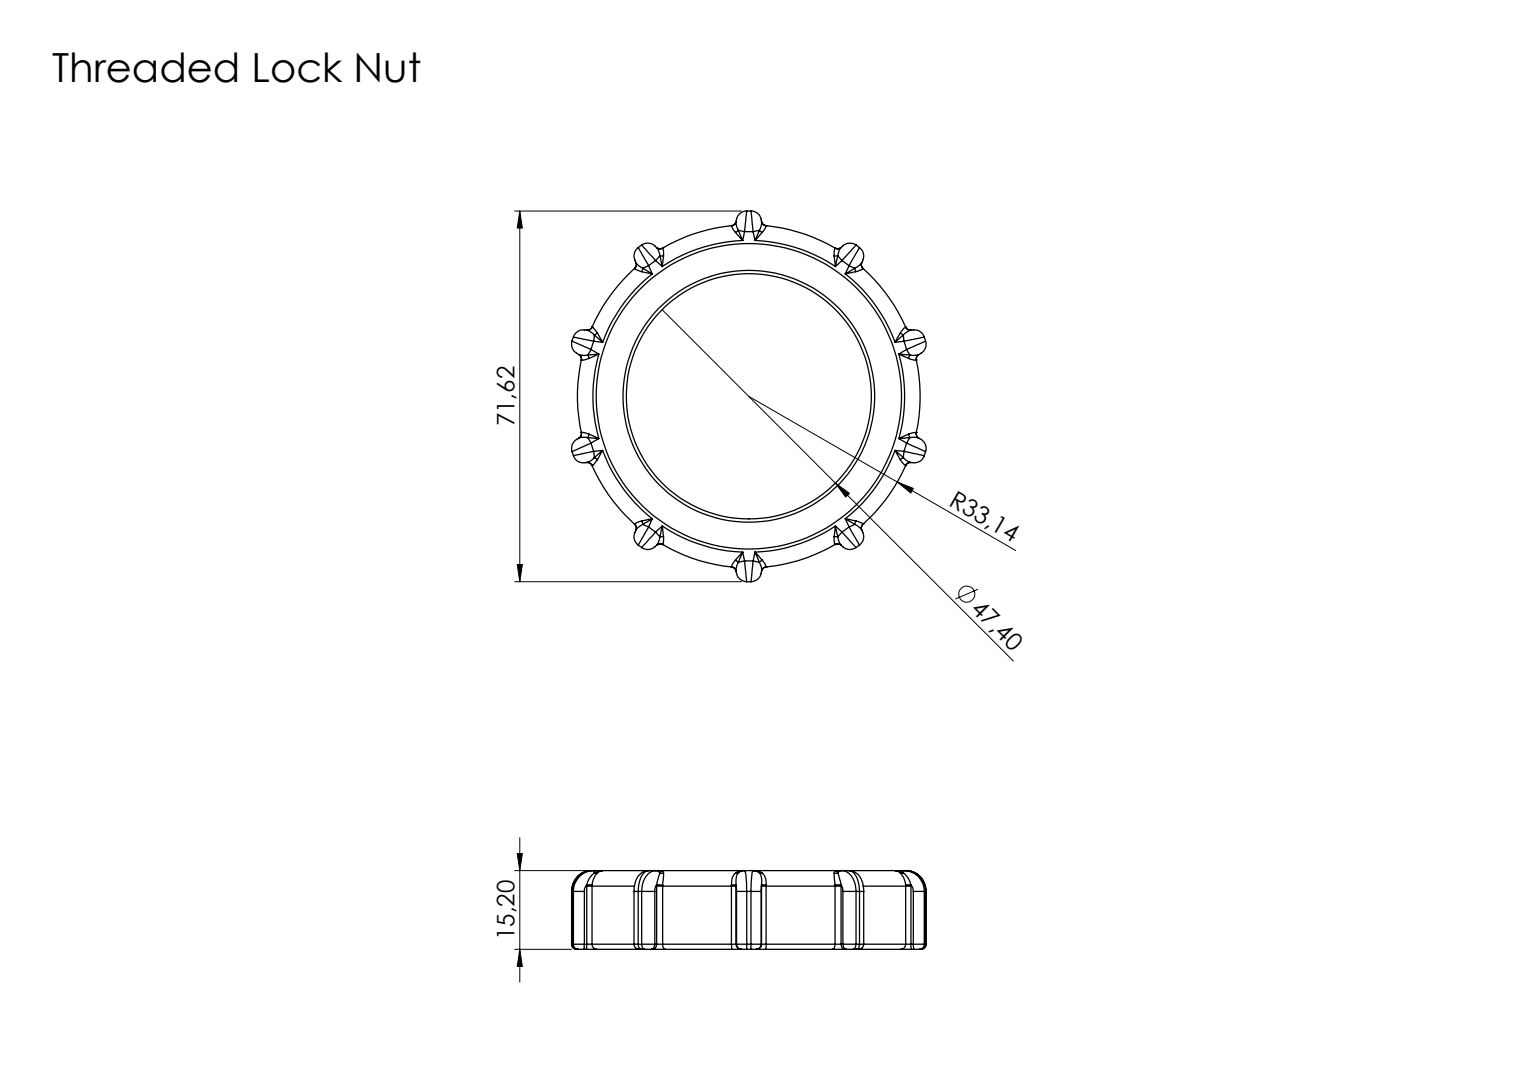
ISO-10303-21;
HEADER;
FILE_DESCRIPTION (('STEP AP214'),
    '1' );
FILE_NAME ('Threaded Lock Nut.step',
    '2026-10-06T09:49:54',
    ( '' ),
    ( '' ),
    'SwSTEP 2.0',
    'SolidWorks 2020',
    '' );
FILE_SCHEMA (( 'AUTOMOTIVE_DESIGN' ));
ENDSEC;

DATA;
#14=( BOUNDED_SURFACE ( )  B_SPLINE_SURFACE ( 3, 2, ( 
 ( #99288, #98203, #90906 ),
 ( #48377, #13076, #82520 ),
 ( #4699, #39956, #23138 ),
 ( #107158, #74130, #50021 ),
 ( #94768, #67940, #76875 ),
 ( #33745, #24238, #102047 ) ),
 .UNSPECIFIED., .F., .F., .F. ) 
 B_SPLINE_SURFACE_WITH_KNOTS ( ( 4, 2, 4 ),
 ( 3, 3 ),
 ( -1.474514954580286030E-17, 0.001312027981647312597, 0.002624055963294639939 ),
 ( 0.000000000000000000, 1.000000000000000000 ),
 .UNSPECIFIED. ) 
 GEOMETRIC_REPRESENTATION_ITEM ( )  RATIONAL_B_SPLINE_SURFACE ( (
 ( 1.000000000000000000, 0.9376006582765906705, 1.000000000000000000),
 ( 1.000000000000000000, 0.9569320108021501792, 1.000000000000000000),
 ( 1.000000000000000000, 0.9725743441620362528, 1.000000000000000000),
 ( 1.000000000000000000, 0.9942095667134138726, 1.000000000000000000),
 ( 1.000000000000000000, 1.000043666450818769, 1.000000000000000000),
 ( 1.000000000000000000, 1.000000000000000000, 1.000000000000000000) ) ) 
 REPRESENTATION_ITEM ( '' )  SURFACE ( )  );
#35=AXIS2_PLACEMENT_3D ( 'NONE', #53186, #17882, #45348 ) ;
#47=ORIENTED_EDGE ( 'NONE', *, *, #28974, .T. ) ;
#67=CARTESIAN_POINT ( 'NONE',  ( -1.491506560153236682, 1512.187213306747481, 242.6732489767341576 ) ) ;
#79=CARTESIAN_POINT ( 'NONE',  ( 21.64985223704960049, 1524.547395018738371, 234.6923279487310197 ) ) ;
#92=AXIS2_PLACEMENT_3D ( 'NONE', #81436, #4747, #22069 ) ;
#98=CARTESIAN_POINT ( 'NONE',  ( 32.97913964219430483, 1512.187213306747481, 197.9697544589745632 ) ) ;
#103=CARTESIAN_POINT ( 'NONE',  ( -2.622430729442981168, 1523.621879633028584, 242.1535192357228254 ) ) ;
#104=CARTESIAN_POINT ( 'NONE',  ( 2.470168521978398868, 1512.187213306747481, 175.3649660270905315 ) ) ;
#113=ORIENTED_EDGE ( 'NONE', *, *, #67279, .T. ) ;
#132=AXIS2_PLACEMENT_3D ( 'NONE', #29173, #87435, #11285 ) ;
#135=ORIENTED_EDGE ( 'NONE', *, *, #51675, .F. ) ;
#155=ORIENTED_EDGE ( 'NONE', *, *, #76478, .F. ) ;
#158=DIRECTION ( 'NONE',  ( 0.8672669759446630655, 0.000000000000000000, -0.4978433412588735285 ) ) ;
#164=AXIS2_PLACEMENT_3D ( 'NONE', #96746, #87233, #71584 ) ;
#171=ORIENTED_EDGE ( 'NONE', *, *, #62426, .F. ) ;
#178=DIRECTION ( 'NONE',  ( 0.000000000000000000, 0.000000000000000000, 1.000000000000000000 ) ) ;
#184=CIRCLE ( 'NONE', #28783, 1.000000000000007994 ) ;
#191=CARTESIAN_POINT ( 'NONE',  ( -20.12564951288306503, 1512.187213306747481, 180.7149624981946658 ) ) ;
#194=DIRECTION ( 'NONE',  ( -0.000000000000000000, -1.000000000000000000, 0.000000000000000000 ) ) ;
#196=CARTESIAN_POINT ( 'NONE',  ( 17.03788438627352519, 1524.775785348137333, 181.0918340916085754 ) ) ;
#216=CARTESIAN_POINT ( 'NONE',  ( 21.50855465202003813, 1524.374578187333327, 184.1253178261501660 ) ) ;
#237=VERTEX_POINT ( 'NONE', #65385 ) ;
#265=EDGE_CURVE ( 'NONE', #68013, #83547, #85444, .T. ) ;
#275=EDGE_LOOP ( 'NONE', ( #35605, #7044, #107686, #49764, #7625 ) ) ;
#282=AXIS2_PLACEMENT_3D ( 'NONE', #69728, #96558, #36645 ) ;
#285=LINE ( 'NONE', #92652, #110374 ) ;
#287=B_SPLINE_CURVE_WITH_KNOTS ( 'NONE', 3,
 ( #66514, #15499, #49697, #83827, #109592, #28341 ),
 .UNSPECIFIED., .F., .F.,
 ( 4, 2, 4 ),
 ( 2.797157557069881010E-17, 0.001087661325621732452, 0.002175322651243436715 ),
 .UNSPECIFIED. ) ;
#298=CARTESIAN_POINT ( 'NONE',  ( 18.86027053263898168, 1512.187213306747481, 230.7762769316004778 ) ) ;
#313=CARTESIAN_POINT ( 'NONE',  ( 31.55762699681125127, 1523.390106123591067, 196.3178534513329794 ) ) ;
#324=EDGE_CURVE ( 'NONE', #40683, #47896, #52438, .T. ) ;
#330=DIRECTION ( 'NONE',  ( -0.4978433412588676998, 0.000000000000000000, 0.8672669759446663962 ) ) ;
#338=B_SPLINE_CURVE_WITH_KNOTS ( 'NONE', 3,
 ( #14649, #33638, #59986, #52681 ),
 .UNSPECIFIED., .F., .F.,
 ( 4, 4 ),
 ( 0.000000000000000000, 0.0002960034161023847852 ),
 .UNSPECIFIED. ) ;
#359=EDGE_CURVE ( 'NONE', #10483, #4434, #57345, .T. ) ;
#394=TOROIDAL_SURFACE ( 'NONE', #71885, 30.13701971169416538, 3.000000000000000000 ) ;
#397=CARTESIAN_POINT ( 'NONE',  ( -29.67375955050042791, 1525.697946996596102, 221.2718133379099186 ) ) ;
#411=CARTESIAN_POINT ( 'NONE',  ( -33.93019615848938741, 1501.977400791986611, 220.5829544587966211 ) ) ;
#425=CARTESIAN_POINT ( 'NONE',  ( 2.570812331889315683, 1525.317349363550647, 176.7848501982247740 ) ) ;
#431=CARTESIAN_POINT ( 'NONE',  ( 16.66231036550702882, 1523.604703353109699, 180.4882076302513383 ) ) ;
#442=CARTESIAN_POINT ( 'NONE',  ( 0.000000000000000000, 1523.382868172864164, 209.1218459616979999 ) ) ;
#447=CARTESIAN_POINT ( 'NONE',  ( -19.53786426059057746, 1512.187213306747481, 181.5239794925695946 ) ) ;
#457=LINE ( 'NONE', #76585, #6239 ) ;
#461=CARTESIAN_POINT ( 'NONE',  ( 2.470955845399090300, 1523.580203803270933, 175.3687159542604377 ) ) ;
#490=DIRECTION ( 'NONE',  ( -0.000000000000000000, -1.000000000000000000, -0.000000000000000000 ) ) ;
#492=ORIENTED_EDGE ( 'NONE', *, *, #6899, .T. ) ;
#498=EDGE_LOOP ( 'NONE', ( #7346, #75123, #33311, #49048 ) ) ;
#501=CARTESIAN_POINT ( 'NONE',  ( -2.478666945488134932, 1524.659148609483054, 175.7709333987998548 ) ) ;
#506=CARTESIAN_POINT ( 'NONE',  ( 34.18677586421181758, 1522.382868172863937, 198.4504086008745389 ) ) ;
#518=DIRECTION ( 'NONE',  ( 0.000000000000000000, 0.000000000000000000, 1.000000000000000000 ) ) ;
#554=DIRECTION ( 'NONE',  ( -0.9942586961433764747, 0.000000000000000000, -0.1070030146457237041 ) ) ;
#563=DIRECTION ( 'NONE',  ( 0.000000000000000000, 0.000000000000000000, 1.000000000000000000 ) ) ;
#621=LINE ( 'NONE', #33094, #954 ) ;
#626=B_SPLINE_CURVE_WITH_KNOTS ( 'NONE', 3,
 ( #68362, #23563, #84575, #93517, #75649, #76185, #40921, #67801 ),
 .UNSPECIFIED., .F., .F.,
 ( 4, 2, 2, 4 ),
 ( 3.035766082959412415E-18, 0.001073044933456185606, 0.001609567400184306381, 0.002146089866912427591 ),
 .UNSPECIFIED. ) ;
#645=ORIENTED_EDGE ( 'NONE', *, *, #26884, .F. ) ;
#650=LINE ( 'NONE', #52152, #84998 ) ;
#657=ORIENTED_EDGE ( 'NONE', *, *, #45659, .F. ) ;
#680=CARTESIAN_POINT ( 'NONE',  ( -16.68062049856743201, 1524.382868172863937, 181.4122394607864521 ) ) ;
#682=( BOUNDED_CURVE ( )  B_SPLINE_CURVE ( 3, ( #67217, #42542, #1115, #52615 ),
 .UNSPECIFIED., .F., .F. ) 
 B_SPLINE_CURVE_WITH_KNOTS ( ( 4, 4 ),
 ( 2.436781329611985569, 3.141592653589793116 ),
 .UNSPECIFIED. ) 
 CURVE ( )  GEOMETRIC_REPRESENTATION_ITEM ( )  RATIONAL_B_SPLINE_CURVE ( ( 1.000000000000000000, 0.9590300661663091475, 0.9590300661663091475, 1.000000000000000000 ) ) 
 REPRESENTATION_ITEM ( '' )  );
#718=LINE ( 'NONE', #6885, #16918 ) ;
#728=CARTESIAN_POINT ( 'NONE',  ( -19.53786426059057746, 1512.187213306747481, 179.5239794925695946 ) ) ;
#736=CARTESIAN_POINT ( 'NONE',  ( 17.24701964721146297, 1523.844782250842400, 180.8504346226932569 ) ) ;
#749=FACE_OUTER_BOUND ( 'NONE', #68574, .T. ) ;
#812=CARTESIAN_POINT ( 'NONE',  ( 156.6846457583361882, 1524.382868172863937, 340.9912860285725174 ) ) ;
#821=CARTESIAN_POINT ( 'NONE',  ( 20.06033034266344828, 1526.189892541618974, 233.0619703228597643 ) ) ;
#830=EDGE_LOOP ( 'NONE', ( #94254, #75571, #96496 ) ) ;
#838=CARTESIAN_POINT ( 'NONE',  ( 34.68852446352940433, 1522.382868172863937, 199.9946320047950223 ) ) ;
#845=DIRECTION ( 'NONE',  ( -0.9125304618754018771, 0.000000000000000000, 0.4090087482554204401 ) ) ;
#848=CARTESIAN_POINT ( 'NONE',  ( 18.66420869458043441, 1526.382868172864164, 185.4599087859680537 ) ) ;
#850=ORIENTED_EDGE ( 'NONE', *, *, #22937, .F. ) ;
#858=CARTESIAN_POINT ( 'NONE',  ( 18.69816095120771493, 1522.382868172863937, 234.8576566410002897 ) ) ;
#863=EDGE_CURVE ( 'NONE', #108182, #30075, #109280, .T. ) ;
#870=EDGE_CURVE ( 'NONE', #24039, #32377, #39575, .T. ) ;
#875=EDGE_LOOP ( 'NONE', ( #11921, #86315, #53502, #106235 ) ) ;
#897=CARTESIAN_POINT ( 'NONE',  ( -30.95751052620455468, 1525.821544997590081, 201.4531494772889744 ) ) ;
#911=VERTEX_POINT ( 'NONE', #76256 ) ;
#912=FACE_OUTER_BOUND ( 'NONE', #72919, .T. ) ;
#941=CARTESIAN_POINT ( 'NONE',  ( -30.57821243133623668, 1525.253972588461693, 221.5701747116904130 ) ) ;
#942=VECTOR ( 'NONE', #92209, 1000.000000000000000 ) ;
#949=CARTESIAN_POINT ( 'NONE',  ( 22.08622291482349809, 1523.382868172864164, 233.8253038720783650 ) ) ;
#954=VECTOR ( 'NONE', #58866, 1000.000000000000114 ) ;
#956=EDGE_CURVE ( 'NONE', #90273, #106841, #7354, .T. ) ;
#957=DIRECTION ( 'NONE',  ( 0.000000000000000000, 1.000000000000000000, 0.000000000000000000 ) ) ;
#967=VERTEX_POINT ( 'NONE', #52531 ) ;
#970=CARTESIAN_POINT ( 'NONE',  ( 3.351189091698004940, 1524.075132568163781, 176.2264789961865006 ) ) ;
#972=CARTESIAN_POINT ( 'NONE',  ( -30.15585515321768995, 1524.425415513989719, 195.8365654344459870 ) ) ;
#988=FACE_OUTER_BOUND ( 'NONE', #72451, .T. ) ;
#989=DIRECTION ( 'NONE',  ( 0.000000000000000000, 0.000000000000000000, -1.000000000000000000 ) ) ;
#996=LINE ( 'NONE', #18854, #12421 ) ;
#1008=DIRECTION ( 'NONE',  ( 6.938893903907222067E-15, 0.000000000000000000, 1.000000000000000000 ) ) ;
#1017=DIRECTION ( 'NONE',  ( 0.03006000153033951128, -0.4884709562387339332, -0.8720622232497018400 ) ) ;
#1019=ADVANCED_FACE ( 'NONE', ( #35713 ), #50299, .T. ) ;
#1042=ORIENTED_EDGE ( 'NONE', *, *, #56606, .F. ) ;
#1054=DIRECTION ( 'NONE',  ( 0.000000000000000000, 1.000000000000000000, 0.000000000000000000 ) ) ;
#1071=CIRCLE ( 'NONE', #13577, 1.000000000000000888 ) ;
#1087=DIRECTION ( 'NONE',  ( 0.9977304882603014180, -0.06733403890946067227, 0.000000000000000000 ) ) ;
#1091=CARTESIAN_POINT ( 'NONE',  ( 30.04668324475564489, 1524.739563915922872, 195.9292732422738084 ) ) ;
#1093=CARTESIAN_POINT ( 'NONE',  ( -16.50400130224786466, 1525.907212628473644, 181.9890130758379030 ) ) ;
#1098=CARTESIAN_POINT ( 'NONE',  ( -1.336192060408252891, 1526.382868172863937, 178.6759496289172091 ) ) ;
#1115=CARTESIAN_POINT ( 'NONE',  ( 33.28034951413929576, 1522.862737210649584, 217.4407153818819438 ) ) ;
#1118=EDGE_CURVE ( 'NONE', #65949, #81284, #12787, .T. ) ;
#1127=EDGE_LOOP ( 'NONE', ( #104674, #75950, #35545, #11204 ) ) ;
#1142=DIRECTION ( 'NONE',  ( -0.7454942576402798782, -1.849942558231146277E-14, 0.6665120492724555534 ) ) ;
#1143=DIRECTION ( 'NONE',  ( 0.000000000000000000, 0.000000000000000000, 1.000000000000000000 ) ) ;
#1159=CARTESIAN_POINT ( 'NONE',  ( -30.04822308544821041, 1524.382868172804365, 221.7633950662771838 ) ) ;
#1193=CARTESIAN_POINT ( 'NONE',  ( -20.58427237330537096, 1512.187213306747481, 216.4826520421591738 ) ) ;
#1195=ORIENTED_EDGE ( 'NONE', *, *, #21286, .F. ) ;
#1198=CARTESIAN_POINT ( 'NONE',  ( 0.000000000000000000, 1518.913060387330006, 209.1218459616979999 ) ) ;
#1228=CARTESIAN_POINT ( 'NONE',  ( 29.86461515634908892, 1525.960063244516959, 197.2746849027934957 ) ) ;
#1229=CARTESIAN_POINT ( 'NONE',  ( -21.15382147014703662, 1525.425665131969254, 234.2558076767862190 ) ) ;
#1233=ORIENTED_EDGE ( 'NONE', *, *, #80838, .T. ) ;
#1250=EDGE_CURVE ( 'NONE', #83385, #104688, #28736, .T. ) ;
#1252=CARTESIAN_POINT ( 'NONE',  ( 17.73223409949387275, 1524.152444737676660, 237.7705223289944172 ) ) ;
#1265=CARTESIAN_POINT ( 'NONE',  ( 32.38845791999495560, 1518.913060387330006, 202.1182848005512085 ) ) ;
#1268=FACE_OUTER_BOUND ( 'NONE', #50912, .T. ) ;
#1287=CARTESIAN_POINT ( 'NONE',  ( 16.62425451295026946, 1524.075000532257491, 180.5391494807173842 ) ) ;
#1297=CARTESIAN_POINT ( 'NONE',  ( -19.53786426059057746, 1501.977400791986611, 181.5239794925695946 ) ) ;
#1306=CARTESIAN_POINT ( 'NONE',  ( 21.30905559964021023, 1524.964230758883104, 184.3256122676305893 ) ) ;
#1308=CARTESIAN_POINT ( 'NONE',  ( -0.4151546846821903003, 1512.187213306747481, 174.3106345060153046 ) ) ;
#1319=CARTESIAN_POINT ( 'NONE',  ( 32.78250617288045987, 1511.187213306747708, 218.3079823578266314 ) ) ;
#1324=ORIENTED_EDGE ( 'NONE', *, *, #28391, .T. ) ;
#1350=CARTESIAN_POINT ( 'NONE',  ( -31.34137657934001098, 1512.187213306747481, 221.9025654077414345 ) ) ;
#1362=ORIENTED_EDGE ( 'NONE', *, *, #19366, .T. ) ;
#1381=FACE_OUTER_BOUND ( 'NONE', #3200, .T. ) ;
#1385=DIRECTION ( 'NONE',  ( -0.000000000000000000, -1.000000000000000000, 0.000000000000000000 ) ) ;
#1386=ADVANCED_FACE ( 'NONE', ( #90829 ), #74050, .T. ) ;
#1398=CARTESIAN_POINT ( 'NONE',  ( -31.81407709660784988, 1522.382868172863937, 196.2902540610631945 ) ) ;
#1400=DIRECTION ( 'NONE',  ( -0.03006000153037464637, -0.4884709562387478665, -0.8720622232496929582 ) ) ;
#1431=CARTESIAN_POINT ( 'NONE',  ( -32.09351624765574940, 1524.374142163904025, 201.5415833658115901 ) ) ;
#1433=CARTESIAN_POINT ( 'NONE',  ( 16.66231036550724198, 1523.604703353109699, 237.7554842931445478 ) ) ;
#1438=DIRECTION ( 'NONE',  ( -0.9942586961433761417, -1.225281874271768203E-16, -0.1070030146457283393 ) ) ;
#1452=ORIENTED_EDGE ( 'NONE', *, *, #34105, .T. ) ;
#1464=EDGE_CURVE ( 'NONE', #13274, #40624, #28589, .T. ) ;
#1467=EDGE_CURVE ( 'NONE', #89438, #10483, #27113, .T. ) ;
#1481=CARTESIAN_POINT ( 'NONE',  ( 17.17241001986483795, 1512.187213306747481, 179.6185504016043240 ) ) ;
#1485=EDGE_LOOP ( 'NONE', ( #33168, #31647, #63478, #110389 ) ) ;
#1487=CARTESIAN_POINT ( 'NONE',  ( 2.470168521978401088, 1523.481610426287716, 242.8787258963054683 ) ) ;
#1506=EDGE_LOOP ( 'NONE', ( #67420, #97199, #19165, #75833 ) ) ;
#1516=CARTESIAN_POINT ( 'NONE',  ( -30.24841015875323791, 1524.082740465118832, 195.7700776127339566 ) ) ;
#1525=CARTESIAN_POINT ( 'NONE',  ( 2.397475438392864255, 1525.713797967456685, 243.2249543484664400 ) ) ;
#1531=CIRCLE ( 'NONE', #87365, 1.000000000000000888 ) ;
#1539=CIRCLE ( 'NONE', #69491, 2.000000000000001776 ) ;
#1550=VERTEX_POINT ( 'NONE', #21250 ) ;
#1567=DIRECTION ( 'NONE',  ( 0.000000000000000000, 0.000000000000000000, -1.000000000000000000 ) ) ;
#1568=CARTESIAN_POINT ( 'NONE',  ( 8.840620885073873225, 1512.187213306747481, 223.8289249455313268 ) ) ;
#1575=DIRECTION ( 'NONE',  ( 0.000000000000000000, 0.000000000000000000, 1.000000000000000000 ) ) ;
#1576=EDGE_CURVE ( 'NONE', #57810, #42994, #14529, .T. ) ;
#1584=DIRECTION ( 'NONE',  ( 0.000000000000000000, 0.000000000000000000, -1.000000000000000000 ) ) ;
#1594=ORIENTED_EDGE ( 'NONE', *, *, #76038, .T. ) ;
#1617=VECTOR ( 'NONE', #90374, 1000.000000000000114 ) ;
#1648=CARTESIAN_POINT ( 'NONE',  ( -32.86802468386279941, 1523.382868172864164, 217.2040256693919957 ) ) ;
#1651=CARTESIAN_POINT ( 'NONE',  ( 19.37374569213946174, 1526.382868172863937, 234.3668155954418921 ) ) ;
#1654=CARTESIAN_POINT ( 'NONE',  ( -22.69876404240057965, 1501.977400791986611, 236.8953202675781426 ) ) ;
#1665=CARTESIAN_POINT ( 'NONE',  ( -1.191524307911308700, 1526.382868172864164, 239.2353018730791518 ) ) ;
#1677=CARTESIAN_POINT ( 'NONE',  ( 30.90487439922560498, 1525.907212628473644, 216.4335774778780035 ) ) ;
#1685=EDGE_LOOP ( 'NONE', ( #19186, #71769, #109831, #40295 ) ) ;
#1689=CARTESIAN_POINT ( 'NONE',  ( -16.66936639845609491, 1523.382868172864164, 237.7608804993221838 ) ) ;
#1710=EDGE_CURVE ( 'NONE', #5224, #18098, #40044, .T. ) ;
#1737=VECTOR ( 'NONE', #83866, 1000.000000000000227 ) ;
#1751=DIRECTION ( 'NONE',  ( -0.7414773880254664773, 0.000000000000000000, 0.6709778558543730842 ) ) ;
#1753=EDGE_CURVE ( 'NONE', #23788, #59464, #24444, .T. ) ;
#1757=CARTESIAN_POINT ( 'NONE',  ( 17.84338787571921969, 1512.187213306747481, 180.3600277896298110 ) ) ;
#1790=VECTOR ( 'NONE', #84858, 1000.000000000000000 ) ;
#1795=DIRECTION ( 'NONE',  ( -0.000000000000000000, -1.000000000000000000, -0.000000000000000000 ) ) ;
#1813=CARTESIAN_POINT ( 'NONE',  ( -32.92528853941059452, 1523.611961620354123, 217.2368972417797863 ) ) ;
#1832=DIRECTION ( 'NONE',  ( 0.000000000000000000, 1.000000000000000000, 0.000000000000000000 ) ) ;
#1834=CARTESIAN_POINT ( 'NONE',  ( -30.15498238787951379, 1525.730671215514803, 196.9950476445848722 ) ) ;
#1854=CARTESIAN_POINT ( 'NONE',  ( 3.246772394788719929, 1511.187213306747708, 177.1492560608742224 ) ) ;
#1865=DIRECTION ( 'NONE',  ( 7.105427357601001859E-15, 0.000000000000000000, 1.000000000000000000 ) ) ;
#1870=CARTESIAN_POINT ( 'NONE',  ( -34.18677586421173231, 1512.187213306747481, 219.7932833225216882 ) ) ;
#1872=ORIENTED_EDGE ( 'NONE', *, *, #17077, .F. ) ;
#1875=CARTESIAN_POINT ( 'NONE',  ( 21.42841630977322254, 1524.678872986481338, 184.2224299175816782 ) ) ;
#1879=CARTESIAN_POINT ( 'NONE',  ( -32.37018134260410562, 1511.187213306747708, 200.1723992780599986 ) ) ;
#1882=CARTESIAN_POINT ( 'NONE',  ( 0.4151546846821903003, 1512.187213306747481, 174.3106345060153046 ) ) ;
#1895=VERTEX_POINT ( 'NONE', #51314 ) ;
#1919=FACE_OUTER_BOUND ( 'NONE', #94382, .T. ) ;
#1926=DIRECTION ( 'NONE',  ( 0.000000000000000000, 0.000000000000000000, -1.000000000000000000 ) ) ;
#1932=CARTESIAN_POINT ( 'NONE',  ( 30.15954682509860518, 1524.412928176728883, 222.4099428256023145 ) ) ;
#1963=EDGE_LOOP ( 'NONE', ( #6488, #63190, #36975, #109476, #109814 ) ) ;
#1974=CIRCLE ( 'NONE', #59192, 2.000000000000001776 ) ;
#1975=B_SPLINE_CURVE_WITH_KNOTS ( 'NONE', 3,
 ( #55220, #37302, #79860, #82037, #11547, #12644 ),
 .UNSPECIFIED., .F., .F.,
 ( 4, 2, 4 ),
 ( -1.285435071114344984E-05, 0.001079388306740470182, 0.002171630964192083728 ),
 .UNSPECIFIED. ) ;
#1999=ORIENTED_EDGE ( 'NONE', *, *, #72805, .F. ) ;
#2007=CARTESIAN_POINT ( 'NONE',  ( -32.54505059146748636, 1524.547395018738371, 201.1603553390793877 ) ) ;
#2029=AXIS2_PLACEMENT_3D ( 'NONE', #73611, #81412, #69901 ) ;
#2032=CARTESIAN_POINT ( 'NONE',  ( 30.31052258194596760, 1523.604703353109699, 222.4930856806589645 ) ) ;
#2039=ORIENTED_EDGE ( 'NONE', *, *, #25225, .T. ) ;
#2049=CARTESIAN_POINT ( 'NONE',  ( -29.86461515634905695, 1525.960063244516959, 220.9690070206026178 ) ) ;
#2057=CARTESIAN_POINT ( 'NONE',  ( 21.84020450211309949, 1523.481610118014487, 234.9798068777342621 ) ) ;
#2062=TOROIDAL_SURFACE ( 'NONE', #27074, 2.000000000000000000, 1.000000000000000000 ) ;
#2073=CARTESIAN_POINT ( 'NONE',  ( -19.91074080903786481, 1526.211528530236592, 184.7300577086374460 ) ) ;
#2075=AXIS2_PLACEMENT_3D ( 'NONE', #44071, #94439, #26132 ) ;
#2084=CARTESIAN_POINT ( 'NONE',  ( 34.18677586421183889, 1524.726013923371283, 198.4504086008744821 ) ) ;
#2104=ADVANCED_FACE ( 'NONE', ( #59734 ), #62997, .F. ) ;
#2107=DIRECTION ( 'NONE',  ( -0.000000000000000000, -1.000000000000000000, -0.000000000000000000 ) ) ;
#2119=CARTESIAN_POINT ( 'NONE',  ( 21.41971086555086501, 1512.187213306747481, 185.1638823089577670 ) ) ;
#2133=DIRECTION ( 'NONE',  ( 0.9942586961433768078, -1.225281874271768203E-16, 0.1070030146457215670 ) ) ;
#2134=ORIENTED_EDGE ( 'NONE', *, *, #30820, .F. ) ;
#2142=AXIS2_PLACEMENT_3D ( 'NONE', #10875, #61851, #26549 ) ;
#2148=( BOUNDED_CURVE ( )  B_SPLINE_CURVE ( 3, ( #59261, #8266, #50841, #58699 ),
 .UNSPECIFIED., .F., .T. ) 
 B_SPLINE_CURVE_WITH_KNOTS ( ( 4, 4 ),
 ( 0.000000000000000000, 0.7048113239778038830 ),
 .UNSPECIFIED. ) 
 CURVE ( )  GEOMETRIC_REPRESENTATION_ITEM ( )  RATIONAL_B_SPLINE_CURVE ( ( 1.000000000000000000, 0.9590300661663093695, 0.9590300661663093695, 1.000000000000000000 ) ) 
 REPRESENTATION_ITEM ( '' )  );
#2152=CARTESIAN_POINT ( 'NONE',  ( -76.99707197885047094, 1526.382868172863937, 398.8876973329340672 ) ) ;
#2166=CARTESIAN_POINT ( 'NONE',  ( -28.27139721233049485, 1526.382868172864164, 198.6830693683576499 ) ) ;
#2182=FACE_BOUND ( 'NONE', #61413, .T. ) ;
#2207=ADVANCED_FACE ( 'NONE', ( #57418 ), #23769, .T. ) ;
#2212=EDGE_LOOP ( 'NONE', ( #89470, #53230, #10682, #27900 ) ) ;
#2214=FACE_OUTER_BOUND ( 'NONE', #35175, .T. ) ;
#2219=AXIS2_PLACEMENT_3D ( 'NONE', #101752, #25040, #67643 ) ;
#2234=AXIS2_PLACEMENT_3D ( 'NONE', #36746, #10997, #20467 ) ;
#2236=DIRECTION ( 'NONE',  ( 0.000000000000000000, 0.000000000000000000, 1.000000000000000000 ) ) ;
#2251=CARTESIAN_POINT ( 'NONE',  ( -32.09337683451324352, 1524.374578187333555, 216.7020508011439972 ) ) ;
#2268=EDGE_CURVE ( 'NONE', #106220, #56418, #68854, .T. ) ;
#2279=CARTESIAN_POINT ( 'NONE',  ( 32.09337683451773415, 1524.374578187332645, 201.5416411222501267 ) ) ;
#2305=ORIENTED_EDGE ( 'NONE', *, *, #6899, .F. ) ;
#2326=ORIENTED_EDGE ( 'NONE', *, *, #108860, .T. ) ;
#2351=CARTESIAN_POINT ( 'NONE',  ( -18.88880210473032761, 1524.667648926078527, 179.4140113511354855 ) ) ;
#2354=( BOUNDED_SURFACE ( )  B_SPLINE_SURFACE ( 3, 2, ( 
 ( #65120, #13571, #21961 ),
 ( #48879, #74620, #64030 ),
 ( #48321, #30945, #98144 ),
 ( #4651, #30392, #5760 ),
 ( #38243, #99231, #22509 ),
 ( #56711, #90846, #14131 ),
 ( #99787, #64582, #107103 ),
 ( #98702, #90290, #47211 ),
 ( #5194, #23078, #55630 ),
 ( #15224, #4118, #39901 ) ),
 .UNSPECIFIED., .F., .F., .T. ) 
 B_SPLINE_SURFACE_WITH_KNOTS ( ( 4, 2, 2, 2, 4 ),
 ( 3, 3 ),
 ( 1.570796326794896558, 1.963495408493620697, 2.356194490192344837, 2.748893571891068976, 3.141592653589793116 ),
 ( 0.000000000000000000, 1.000000000000000000 ),
 .UNSPECIFIED. ) 
 GEOMETRIC_REPRESENTATION_ITEM ( )  RATIONAL_B_SPLINE_SURFACE ( (
 ( 1.000000000000000000, 0.7071067811865862085, 1.000000000000000000),
 ( 1.000000000000000000, 0.7166207884822426433, 1.000000000000000000),
 ( 1.000000000000000000, 0.7259222650906650420, 1.000000000000000000),
 ( 1.000000000000000000, 0.7428408967930791862, 1.000000000000000000),
 ( 1.000000000000000000, 0.7504512394528564112, 1.000000000000000000),
 ( 1.000000000000000000, 0.7630177051946440692, 1.000000000000000000),
 ( 1.000000000000000000, 0.7679730451973161287, 1.000000000000000000),
 ( 1.000000000000000000, 0.7746454561797309069, 1.000000000000000000),
 ( 1.000000000000000000, 0.7763684247035169683, 1.000000000000000000),
 ( 1.000000000000000000, 0.7763623250684379418, 1.000000000000000000) ) ) 
 REPRESENTATION_ITEM ( '' )  SURFACE ( )  );
#2363=DIRECTION ( 'NONE',  ( 0.000000000000000000, 1.000000000000000000, 0.000000000000000000 ) ) ;
#2365=ADVANCED_FACE ( 'NONE', ( #55352 ), #21144, .T. ) ;
#2377=CARTESIAN_POINT ( 'NONE',  ( 20.79738390328738973, 1512.187213306747481, 237.0406858230487899 ) ) ;
#2379=CARTESIAN_POINT ( 'NONE',  ( 17.43549085681724620, 1525.211473355384896, 237.2113236654630555 ) ) ;
#2387=CARTESIAN_POINT ( 'NONE',  ( 19.53786426059039982, 1512.187213306747481, 236.7197124308265188 ) ) ;
#2394=DIRECTION ( 'NONE',  ( -0.8090169943749422332, 0.000000000000000000, 0.5877852522924802425 ) ) ;
#2406=DIRECTION ( 'NONE',  ( -0.000000000000000000, -1.000000000000000000, -0.000000000000000000 ) ) ;
#2419=DIRECTION ( 'NONE',  ( -0.9510565162951559737, 0.000000000000000000, 0.3090169943749403458 ) ) ;
#2428=( LENGTH_UNIT ( ) NAMED_UNIT ( * ) SI_UNIT ( .MILLI., .METRE. ) );
#2431=ORIENTED_EDGE ( 'NONE', *, *, #101280, .T. ) ;
#2450=ORIENTED_EDGE ( 'NONE', *, *, #90057, .F. ) ;
#2457=FACE_OUTER_BOUND ( 'NONE', #57047, .T. ) ;
#2465=DIRECTION ( 'NONE',  ( 0.000000000000000000, 0.000000000000000000, 1.000000000000000000 ) ) ;
#2470=B_SPLINE_CURVE_WITH_KNOTS ( 'NONE', 3,
 ( #80697, #56045, #90172, #47644, #14015, #91291, #48205, #99120, #82343, #65559 ),
 .UNSPECIFIED., .F., .F.,
 ( 4, 2, 2, 2, 4 ),
 ( 0.000000000000000000, 0.0007403986298595355894, 0.001480797259719071179, 0.002221195889578606551, 0.002961594519438142357 ),
 .UNSPECIFIED. ) ;
#2472=ORIENTED_EDGE ( 'NONE', *, *, #39779, .T. ) ;
#2479=DIRECTION ( 'NONE',  ( -0.5877852522924780221, 0.000000000000000000, -0.8090169943749438985 ) ) ;
#2486=CARTESIAN_POINT ( 'NONE',  ( -31.55061275096994322, 1525.712830164893376, 217.0331825386441835 ) ) ;
#2494=CARTESIAN_POINT ( 'NONE',  ( -16.55387768533248760, 1524.739563915921963, 237.4558587828119300 ) ) ;
#2514=LINE ( 'NONE', #19254, #14480 ) ;
#2553=CIRCLE ( 'NONE', #40081, 33.13701971169416538 ) ;
#2560=DIRECTION ( 'NONE',  ( 0.000000000000000000, 0.000000000000000000, 1.000000000000000000 ) ) ;
#2566=CARTESIAN_POINT ( 'NONE',  ( -32.70818033930468971, 1524.201670966335314, 201.1172547305815499 ) ) ;
#2568=CARTESIAN_POINT ( 'NONE',  ( 32.37018134260406299, 1511.187213306747708, 218.0712926453362002 ) ) ;
#2574=VERTEX_POINT ( 'NONE', #32870 ) ;
#2598=LINE ( 'NONE', #45147, #87430 ) ;
#2608=ORIENTED_EDGE ( 'NONE', *, *, #64704, .T. ) ;
#2614=CARTESIAN_POINT ( 'NONE',  ( -41.95590887306661187, 1512.187213306747481, 225.5974093378525254 ) ) ;
#2627=CARTESIAN_POINT ( 'NONE',  ( -20.79738390328697761, 1512.187213306747481, 237.0406858230491025 ) ) ;
#2634=CARTESIAN_POINT ( 'NONE',  ( -34.09079054513859575, 1524.667648926078755, 200.3377533957330172 ) ) ;
#2635=CARTESIAN_POINT ( 'NONE',  ( -20.87481493262672316, 1525.712830164893376, 234.0672365764787628 ) ) ;
#2643=CARTESIAN_POINT ( 'NONE',  ( 0.4260839224734190300, 1523.429859730332510, 244.8289481157567593 ) ) ;
#2650=CARTESIAN_POINT ( 'NONE',  ( -2.136371150128812957, 1525.856065479248173, 241.3693944374256546 ) ) ;
#2664=ORIENTED_EDGE ( 'NONE', *, *, #37056, .F. ) ;
#2667=CARTESIAN_POINT ( 'NONE',  ( -18.69816095120731347, 1522.382868172863937, 234.8576566410005171 ) ) ;
#2676=AXIS2_PLACEMENT_3D ( 'NONE', #83147, #74218, #41693 ) ;
#2690=ORIENTED_EDGE ( 'NONE', *, *, #104370, .F. ) ;
#2696=FACE_OUTER_BOUND ( 'NONE', #32323, .T. ) ;
#2698=DIRECTION ( 'NONE',  ( 0.8386695113602744556, -0.4884709562387554715, 0.2408932868012610695 ) ) ;
#2719=AXIS2_PLACEMENT_3D ( 'NONE', #1308, #2982, #44980 ) ;
#2724=DIRECTION ( 'NONE',  ( -0.000000000000000000, -1.000000000000000000, -0.000000000000000000 ) ) ;
#2760=B_SPLINE_CURVE_WITH_KNOTS ( 'NONE', 3,
 ( #91547, #40036, #5890, #83688, #100491, #6984, #76396, #68026, #75852, #57959, #24862, #25414 ),
 .UNSPECIFIED., .F., .F.,
 ( 4, 2, 2, 2, 2, 4 ),
 ( 0.000000000000000000, 0.0007194225121803652289, 0.001079133768270242044, 0.001438845024360118968, 0.002158267536539317053, 0.002877690048718515789 ),
 .UNSPECIFIED. ) ;
#2805=CARTESIAN_POINT ( 'NONE',  ( 32.37018134260397062, 1512.187213306747481, 200.1723992780595438 ) ) ;
#2812=ORIENTED_EDGE ( 'NONE', *, *, #94728, .T. ) ;
#2813=VERTEX_POINT ( 'NONE', #60303 ) ;
#2828=CARTESIAN_POINT ( 'NONE',  ( 22.08622291482349809, 1523.456872492435195, 233.8253038720783366 ) ) ;
#2834=CIRCLE ( 'NONE', #61915, 0.9999999999999981126 ) ;
#2854=LINE ( 'NONE', #9023, #17151 ) ;
#2862=CARTESIAN_POINT ( 'NONE',  ( 19.37374569213945463, 1524.382868172863937, 234.3668155954418637 ) ) ;
#2876=ADVANCED_FACE ( 'NONE', ( #80412 ), #17111, .F. ) ;
#2877=VECTOR ( 'NONE', #103941, 1000.000000000000000 ) ;
#2896=CARTESIAN_POINT ( 'NONE',  ( -19.67623451925548039, 1525.581535527370761, 181.0581612214988638 ) ) ;
#2910=CARTESIAN_POINT ( 'NONE',  ( -17.17241001986463189, 1523.382868172864164, 238.6251415217917895 ) ) ;
#2920=ADVANCED_FACE ( 'NONE', ( #14838 ), #57974, .T. ) ;
#2926=CARTESIAN_POINT ( 'NONE',  ( 32.22536377336282953, 1523.621879633028811, 216.8351145222429466 ) ) ;
#2934=ORIENTED_EDGE ( 'NONE', *, *, #96685, .F. ) ;
#2937=CARTESIAN_POINT ( 'NONE',  ( 33.42844755917185751, 1522.382868172863937, 196.1165140606791226 ) ) ;
#2941=CARTESIAN_POINT ( 'NONE',  ( -29.75841426815548019, 1525.320827368860364, 196.2321946361128653 ) ) ;
#2953=DIRECTION ( 'NONE',  ( -3.469446951953611033E-14, 0.000000000000000000, 1.000000000000000000 ) ) ;
#2957=LINE ( 'NONE', #64506, #87287 ) ;
#2964=FACE_OUTER_BOUND ( 'NONE', #105643, .T. ) ;
#2973=DIRECTION ( 'NONE',  ( -0.000000000000000000, -1.000000000000000000, -0.000000000000000000 ) ) ;
#2982=DIRECTION ( 'NONE',  ( -1.000000000000000000, -0.000000000000000000, -0.000000000000000000 ) ) ;
#2998=EDGE_CURVE ( 'NONE', #65697, #94153, #105190, .T. ) ;
#3001=EDGE_LOOP ( 'NONE', ( #74480, #135, #9524, #81135 ) ) ;
#3015=B_SPLINE_CURVE_WITH_KNOTS ( 'NONE', 3,
 ( #84972, #110740, #16106, #42999 ),
 .UNSPECIFIED., .F., .F.,
 ( 4, 4 ),
 ( 0.000000000000000000, 0.0002960034161023847310 ),
 .UNSPECIFIED. ) ;
#3020=ORIENTED_EDGE ( 'NONE', *, *, #23524, .F. ) ;
#3024=DIRECTION ( 'NONE',  ( -0.8672669759446620663, -1.225281874271767957E-16, 0.4978433412588753049 ) ) ;
#3035=CARTESIAN_POINT ( 'NONE',  ( -31.34491535884016855, 1525.848196786131666, 217.0523381734421662 ) ) ;
#3038=CARTESIAN_POINT ( 'NONE',  ( -3.246772394788723481, 1512.187213306747481, 177.1492560608742224 ) ) ;
#3044=CARTESIAN_POINT ( 'NONE',  ( -17.50742245788202922, 1524.972383263453139, 237.3784165796199375 ) ) ;
#3046=CARTESIAN_POINT ( 'NONE',  ( 29.00779973304128134, 1526.382868172864164, 217.2942086403122630 ) ) ;
#3092=DIRECTION ( 'NONE',  ( 0.000000000000000000, -1.000000000000000000, -0.000000000000000000 ) ) ;
#3110=DIRECTION ( 'NONE',  ( -0.9510565162951566398, 0.000000000000000000, -0.3090169943749383474 ) ) ;
#3114=ADVANCED_FACE ( 'NONE', ( #29317 ), #55103, .T. ) ;
#3115=CARTESIAN_POINT ( 'NONE',  ( -32.06267705388219014, 1524.739563915922645, 202.1338641996698016 ) ) ;
#3124=ORIENTED_EDGE ( 'NONE', *, *, #73570, .F. ) ;
#3134=ORIENTED_EDGE ( 'NONE', *, *, #50453, .T. ) ;
#3148=CIRCLE ( 'NONE', #17389, 1.000000000000000888 ) ;
#3158=CARTESIAN_POINT ( 'NONE',  ( -30.95265250778393806, 1524.659148609483054, 221.7851970717786685 ) ) ;
#3174=CARTESIAN_POINT ( 'NONE',  ( 21.53981368633951377, 1523.542365884048422, 183.9340804168593309 ) ) ;
#3182=DIRECTION ( 'NONE',  ( -0.5877852522924562617, 0.000000000000000000, 0.8090169943749596637 ) ) ;
#3200=EDGE_LOOP ( 'NONE', ( #15746, #77246, #26481, #24802 ) ) ;
#3207=CARTESIAN_POINT ( 'NONE',  ( -2.389870119416070082, 1525.253996226948402, 242.0501772481331386 ) ) ;
#3209=CYLINDRICAL_SURFACE ( 'NONE', #54484, 1.000000000000000888 ) ;
#3217=VERTEX_POINT ( 'NONE', #11300 ) ;
#3220=CYLINDRICAL_SURFACE ( 'NONE', #35381, 3.999999999999993339 ) ;
#3237=VECTOR ( 'NONE', #94239, 1000.000000000000000 ) ;
#3239=CYLINDRICAL_SURFACE ( 'NONE', #30010, 0.9999999999999943379 ) ;
#3267=ADVANCED_FACE ( 'NONE', ( #108507 ), #46009, .F. ) ;
#3270=ORIENTED_EDGE ( 'NONE', *, *, #22830, .T. ) ;
#3281=VECTOR ( 'NONE', #62003, 1000.000000000000000 ) ;
#3303=CARTESIAN_POINT ( 'NONE',  ( 32.22536377336271585, 1523.621879633028584, 201.4085774011528542 ) ) ;
#3309=CARTESIAN_POINT ( 'NONE',  ( 2.485146179491022345, 1524.547395018738143, 242.5342643028157852 ) ) ;
#3311=CARTESIAN_POINT ( 'NONE',  ( 3.448830483803564828, 1512.187213306747481, 175.1594891075192209 ) ) ;
#3316=DIRECTION ( 'NONE',  ( 0.5877852522924831291, 0.000000000000000000, 0.8090169943749401238 ) ) ;
#3321=LINE ( 'NONE', #53729, #4841 ) ;
#3332=CARTESIAN_POINT ( 'NONE',  ( -3.059301852550817102, 1525.343727714918259, 176.8478560800957666 ) ) ;
#3337=CARTESIAN_POINT ( 'NONE',  ( -17.12202622828511522, 1526.104292489133286, 235.9427193670834697 ) ) ;
#3349=CARTESIAN_POINT ( 'NONE',  ( -30.90487439922542734, 1525.907212628473644, 216.4335774778784014 ) ) ;
#3352=EDGE_LOOP ( 'NONE', ( #106947, #4880, #33350, #100023, #30456 ) ) ;
#3363=CARTESIAN_POINT ( 'NONE',  ( -2.372478608332516892, 1522.382868172863937, 174.8996806668726549 ) ) ;
#3365=EDGE_LOOP ( 'NONE', ( #58598, #82587, #92902, #20201 ) ) ;
#3367=B_SPLINE_CURVE_WITH_KNOTS ( 'NONE', 3,
 ( #16187, #25142, #102412, #108618, #49833, #109187 ),
 .UNSPECIFIED., .F., .F.,
 ( 4, 2, 4 ),
 ( -1.285435071109398989E-05, 0.001079388306740562773, 0.002171630964192219470 ),
 .UNSPECIFIED. ) ;
#3371=DIRECTION ( 'NONE',  ( -0.000000000000000000, -1.000000000000000000, -0.000000000000000000 ) ) ;
#3372=CARTESIAN_POINT ( 'NONE',  ( 31.32941610406347266, 1525.856065479242716, 201.1886151593328123 ) ) ;
#3385=AXIS2_PLACEMENT_3D ( 'NONE', #2627, #105625, #3182 ) ;
#3395=ORIENTED_EDGE ( 'NONE', *, *, #68151, .F. ) ;
#3399=ORIENTED_EDGE ( 'NONE', *, *, #91858, .T. ) ;
#3422=CARTESIAN_POINT ( 'NONE',  ( 2.038847259689249736, 1522.382868172863937, 173.3106345060153046 ) ) ;
#3442=DIRECTION ( 'NONE',  ( 0.000000000000000000, 1.000000000000000000, 0.000000000000000000 ) ) ;
#3451=DIRECTION ( 'NONE',  ( -0.5030436214085118873, 0.000000000000000000, 0.8642610224696064547 ) ) ;
#3460=CARTESIAN_POINT ( 'NONE',  ( -21.38516915558527742, 1522.906561336852519, 237.8497028174197965 ) ) ;
#3483=CARTESIAN_POINT ( 'NONE',  ( 30.79697748855962303, 1526.178928173327677, 196.3997152352017110 ) ) ;
#3486=CARTESIAN_POINT ( 'NONE',  ( -30.64453888532113268, 1525.163527997504843, 196.6301324186591160 ) ) ;
#3487=AXIS2_PLACEMENT_3D ( 'NONE', #447, #19973, #10478 ) ;
#3488=CARTESIAN_POINT ( 'NONE',  ( 3.347801439296141268, 1518.913060387330006, 176.1543725841967500 ) ) ;
#3489=CARTESIAN_POINT ( 'NONE',  ( 19.30300490008626468, 1526.348417187218047, 233.1578084719440653 ) ) ;
#3504=DIRECTION ( 'NONE',  ( -0.8642610224695904675, 0.000000000000000000, 0.5030436214085395319 ) ) ;
#3505=DIRECTION ( 'NONE',  ( -0.3090169943749447312, -0.000000000000000000, 0.9510565162951544194 ) ) ;
#3517=CYLINDRICAL_SURFACE ( 'NONE', #87453, 1.999999999999998668 ) ;
#3523=AXIS2_PLACEMENT_3D ( 'NONE', #13851, #98969, #13297 ) ;
#3527=ORIENTED_EDGE ( 'NONE', *, *, #9754, .T. ) ;
#3547=AXIS2_PLACEMENT_3D ( 'NONE', #96990, #88590, #88047 ) ;
#3549=ORIENTED_EDGE ( 'NONE', *, *, #64421, .T. ) ;
#3554=CARTESIAN_POINT ( 'NONE',  ( 32.72609422369145449, 1524.152349020271004, 217.1332896956630520 ) ) ;
#3558=AXIS2_PLACEMENT_3D ( 'NONE', #22540, #5792, #107690 ) ;
#3565=ORIENTED_EDGE ( 'NONE', *, *, #91748, .F. ) ;
#3568=ORIENTED_EDGE ( 'NONE', *, *, #9882, .T. ) ;
#3584=CARTESIAN_POINT ( 'NONE',  ( -32.80315919379393819, 1523.919943579690425, 217.1667904774563453 ) ) ;
#3592=CARTESIAN_POINT ( 'NONE',  ( -17.12670006681592128, 1524.374142163904253, 237.3021637559003523 ) ) ;
#3593=AXIS2_PLACEMENT_3D ( 'NONE', #48663, #91738, #72750 ) ;
#3613=CARTESIAN_POINT ( 'NONE',  ( -18.83964618864532881, 1526.382868172863937, 232.8185072403850313 ) ) ;
#3614=TOROIDAL_SURFACE ( 'NONE', #66194, 1.000000000000000000, 1.000000000000000000 ) ;
#3621=AXIS2_PLACEMENT_3D ( 'NONE', #4859, #38463, #72639 ) ;
#3623=CARTESIAN_POINT ( 'NONE',  ( 20.20959865099491992, 1512.187213306747481, 236.2316688286738611 ) ) ;
#3626=CARTESIAN_POINT ( 'NONE',  ( -33.14208818188998151, 1524.841055067850220, 197.8283574329105647 ) ) ;
#3649=TOROIDAL_SURFACE ( 'NONE', #35, 1.000000000000000000, 1.000000000000000000 ) ;
#3677=CARTESIAN_POINT ( 'NONE',  ( -16.81611548244668342, 1526.382868172864164, 183.6985842798727049 ) ) ;
#3681=ORIENTED_EDGE ( 'NONE', *, *, #18018, .T. ) ;
#3692=VECTOR ( 'NONE', #69071, 1000.000000000000000 ) ;
#3693=FACE_OUTER_BOUND ( 'NONE', #70319, .T. ) ;
#3697=CARTESIAN_POINT ( 'NONE',  ( -30.61618914730555119, 1525.211473355384669, 196.6453055283535889 ) ) ;
#3715=ORIENTED_EDGE ( 'NONE', *, *, #63601, .F. ) ;
#3724=AXIS2_PLACEMENT_3D ( 'NONE', #5683, #89127, #40366 ) ;
#3741=CARTESIAN_POINT ( 'NONE',  ( -29.30029655192934257, 1525.907212628473644, 221.3719603026177367 ) ) ;
#3745=FACE_OUTER_BOUND ( 'NONE', #71128, .T. ) ;
#3748=ORIENTED_EDGE ( 'NONE', *, *, #10708, .F. ) ;
#3750=EDGE_CURVE ( 'NONE', #10960, #67163, #71013, .T. ) ;
#3755=CARTESIAN_POINT ( 'NONE',  ( 1.435939366446196575, 1526.382868172863937, 239.4992070516220508 ) ) ;
#3780=EDGE_CURVE ( 'NONE', #81290, #58486, #53436, .T. ) ;
#3791=CARTESIAN_POINT ( 'NONE',  ( 34.31402925621353006, 1524.244163922423468, 200.2096061136539618 ) ) ;
#3809=ORIENTED_EDGE ( 'NONE', *, *, #19899, .T. ) ;
#3821=ORIENTED_EDGE ( 'NONE', *, *, #47977, .F. ) ;
#3827=AXIS2_PLACEMENT_3D ( 'NONE', #16214, #50418, #79473 ) ;
#3848=ORIENTED_EDGE ( 'NONE', *, *, #109496, .T. ) ;
#3857=CARTESIAN_POINT ( 'NONE',  ( 32.38845791999494850, 1523.382868172864164, 202.1182848005511801 ) ) ;
#3861=CARTESIAN_POINT ( 'NONE',  ( 2.700472180933962907, 1524.678541297860875, 241.8613664836760506 ) ) ;
#3876=CARTESIAN_POINT ( 'NONE',  ( -32.06031249785756643, 1524.760046179776054, 202.1360311646459422 ) ) ;
#3878=CARTESIAN_POINT ( 'NONE',  ( -3.351006924987864455, 1524.082582765195411, 176.2279596953965779 ) ) ;
#3883=CARTESIAN_POINT ( 'NONE',  ( 33.93019615848955084, 1522.382868172863937, 220.5829544587961095 ) ) ;
#3888=LINE ( 'NONE', #106320, #16463 ) ;
#3906=CARTESIAN_POINT ( 'NONE',  ( 2.622430729442982056, 1523.621879633028584, 242.1535192357228254 ) ) ;
#3917=DIRECTION ( 'NONE',  ( -0.000000000000000000, -1.000000000000000000, -0.000000000000000000 ) ) ;
#3923=CARTESIAN_POINT ( 'NONE',  ( 31.97146249857578937, 1524.678872986499073, 201.5731023188606912 ) ) ;
#3926=CARTESIAN_POINT ( 'NONE',  ( 31.22294729666619162, 1523.678648413191695, 195.3480975247479705 ) ) ;
#3931=ADVANCED_FACE ( 'NONE', ( #49428 ), #87143, .F. ) ;
#3941=EDGE_CURVE ( 'NONE', #20620, #41312, #69230, .T. ) ;
#3950=DIRECTION ( 'NONE',  ( 0.000000000000000000, 1.000000000000000000, 0.000000000000000000 ) ) ;
#3974=CARTESIAN_POINT ( 'NONE',  ( 0.6235920161070117596, 1525.878013734321485, 175.2961586039432120 ) ) ;
#3980=CARTESIAN_POINT ( 'NONE',  ( -18.02257621027557377, 1526.382868172863937, 235.3484976865589147 ) ) ;
#3994=LINE ( 'NONE', #105332, #99178 ) ;
#3997=CARTESIAN_POINT ( 'NONE',  ( 16.55212241053982325, 1524.756004293092246, 237.4472295103155091 ) ) ;
#4001=CARTESIAN_POINT ( 'NONE',  ( -19.53786426058999481, 1512.187213306747481, 236.7197124308268030 ) ) ;
#4004=DIRECTION ( 'NONE',  ( 0.9983395709201744461, 0.05760296116452706672, 0.000000000000000000 ) ) ;
#4007=CARTESIAN_POINT ( 'NONE',  ( -19.37374569213905318, 1526.382868172863937, 234.3668155954421479 ) ) ;
#4015=CARTESIAN_POINT ( 'NONE',  ( 18.19590854888146580, 1522.382868172863937, 180.0410247165184217 ) ) ;
#4020=CARTESIAN_POINT ( 'NONE',  ( 20.64339891394559601, 1523.429859730330236, 179.9837476533122640 ) ) ;
#4025=ORIENTED_EDGE ( 'NONE', *, *, #48403, .F. ) ;
#4032=CARTESIAN_POINT ( 'NONE',  ( 3.347801439296147041, 1523.382868172864164, 176.1543725841967500 ) ) ;
#4041=ADVANCED_FACE ( 'NONE', ( #9601 ), #9961, .T. ) ;
#4043=ORIENTED_EDGE ( 'NONE', *, *, #59929, .T. ) ;
#4059=CARTESIAN_POINT ( 'NONE',  ( 16.53242990339596474, 1526.073434386619283, 235.9344106296537120 ) ) ;
#4096=B_SPLINE_CURVE_WITH_KNOTS ( 'NONE', 3,
 ( #25862, #52214, #60621, #10187, #2379, #26997, #27545, #1252, #35391, #37042 ),
 .UNSPECIFIED., .F., .F.,
 ( 4, 2, 2, 2, 4 ),
 ( 0.000000000000000000, 0.0007406479101618162336, 0.001481295820323632467, 0.002221943730485448701, 0.002962591640647264934 ),
 .UNSPECIFIED. ) ;
#4105=EDGE_LOOP ( 'NONE', ( #83933, #6129, #93015, #63228 ) ) ;
#4118=CARTESIAN_POINT ( 'NONE',  ( -22.69876404240115519, 1522.382868172864164, 181.3483716558183119 ) ) ;
#4128=CARTESIAN_POINT ( 'NONE',  ( 29.86461515634917774, 1525.960063244516959, 220.9690070206021062 ) ) ;
#4138=CARTESIAN_POINT ( 'NONE',  ( 16.81049281788159178, 1526.143142182266047, 182.6472226615215675 ) ) ;
#4142=EDGE_LOOP ( 'NONE', ( #40394, #38865, #62593, #78516 ) ) ;
#4169=ORIENTED_EDGE ( 'NONE', *, *, #52921, .T. ) ;
#4173=CARTESIAN_POINT ( 'NONE',  ( -19.91075572344583478, 1526.211523310372513, 233.5136430000777921 ) ) ;
#4185=ORIENTED_EDGE ( 'NONE', *, *, #91619, .T. ) ;
#4194=LINE ( 'NONE', #82555, #96942 ) ;
#4204=CARTESIAN_POINT ( 'NONE',  ( -17.19739463999676232, 1525.960063244516959, 181.9833109756550868 ) ) ;
#4213=CARTESIAN_POINT ( 'NONE',  ( -29.30029655192942784, 1525.907212628473872, 196.8717316207789736 ) ) ;
#4217=ORIENTED_EDGE ( 'NONE', *, *, #64472, .T. ) ;
#4222=ORIENTED_EDGE ( 'NONE', *, *, #9770, .F. ) ;
#4231=DIRECTION ( 'NONE',  ( 0.4978433412588735285, 0.000000000000000000, 0.8672669759446630655 ) ) ;
#4238=CARTESIAN_POINT ( 'NONE',  ( -31.32995031131179786, 1523.678648413191922, 221.9013357025049231 ) ) ;
#4246=EDGE_LOOP ( 'NONE', ( #1324, #22500, #53830, #103827, #58472 ) ) ;
#4249=CARTESIAN_POINT ( 'NONE',  ( 49.24962907673571522, 1526.382868172863937, 407.9033880519289710 ) ) ;
#4255=VECTOR ( 'NONE', #76634, 1000.000000000000000 ) ;
#4256=ADVANCED_FACE ( 'NONE', ( #40182 ), #87121, .T. ) ;
#4266=ADVANCED_FACE ( 'NONE', ( #31777 ), #65964, .T. ) ;
#4267=CIRCLE ( 'NONE', #88344, 1.999999999999994893 ) ;
#4289=CARTESIAN_POINT ( 'NONE',  ( 31.55061275097025586, 1525.712830164893376, 201.2105093847520436 ) ) ;
#4292=CARTESIAN_POINT ( 'NONE',  ( -3.351189091698004940, 1524.075132568163781, 242.0172129272094992 ) ) ;
#4307=DIRECTION ( 'NONE',  ( -0.9942586961433765858, 0.000000000000000000, -0.1070030146457237041 ) ) ;
#4322=CARTESIAN_POINT ( 'NONE',  ( 32.59719044532401711, 1523.982201850120191, 201.1951351303495130 ) ) ;
#4325=ORIENTED_EDGE ( 'NONE', *, *, #69514, .T. ) ;
#4333=DIRECTION ( 'NONE',  ( 0.7882878497005212370, 0.000000000000000000, -0.6153066438894746470 ) ) ;
#4336=CARTESIAN_POINT ( 'NONE',  ( -30.29107790644756903, 1523.847233649538339, 222.4926083870301454 ) ) ;
#4343=ORIENTED_EDGE ( 'NONE', *, *, #104951, .T. ) ;
#4383=ADVANCED_FACE ( 'NONE', ( #64178 ), #47800, .T. ) ;
#4392=CARTESIAN_POINT ( 'NONE',  ( 30.31940284289302667, 1523.456924617338245, 222.4933038711250219 ) ) ;
#4401=EDGE_CURVE ( 'NONE', #39734, #98871, #3148, .T. ) ;
#4429=ORIENTED_EDGE ( 'NONE', *, *, #64747, .F. ) ;
#4433=CARTESIAN_POINT ( 'NONE',  ( -22.69876404240057965, 1522.382868172863937, 236.8953202675781426 ) ) ;
#4434=VERTEX_POINT ( 'NONE', #49028 ) ;
#4436=ORIENTED_EDGE ( 'NONE', *, *, #58396, .F. ) ;
#4452=CIRCLE ( 'NONE', #31287, 1.000000000000000000 ) ;
#4488=VERTEX_POINT ( 'NONE', #80957 ) ;
#4489=CIRCLE ( 'NONE', #24113, 1.000000000000000888 ) ;
#4506=ORIENTED_EDGE ( 'NONE', *, *, #50041, .T. ) ;
#4508=CARTESIAN_POINT ( 'NONE',  ( 2.180465155517681275, 1524.667648926078527, 173.9851435850430050 ) ) ;
#4510=CARTESIAN_POINT ( 'NONE',  ( 16.89233068642487723, 1526.349684470114653, 234.8971439265459935 ) ) ;
#4524=VERTEX_POINT ( 'NONE', #74233 ) ;
#4534=CARTESIAN_POINT ( 'NONE',  ( 16.64685887467730296, 1523.847248782568840, 237.7436681237527125 ) ) ;
#4542=CARTESIAN_POINT ( 'NONE',  ( -21.19880661588985760, 1524.382868172863937, 233.5487980989313144 ) ) ;
#4562=ORIENTED_EDGE ( 'NONE', *, *, #60333, .F. ) ;
#4567=DIRECTION ( 'NONE',  ( 0.8200914087126649488, -0.4884709562386962411, 0.2980708074718669276 ) ) ;
#4570=CARTESIAN_POINT ( 'NONE',  ( 2.407253779970412566, 1523.313115944345554, 243.1783812783781116 ) ) ;
#4573=CARTESIAN_POINT ( 'NONE',  ( -17.06401309437957892, 1526.329757971584741, 237.1783921619734770 ) ) ;
#4576=DIRECTION ( 'NONE',  ( 0.000000000000000000, 1.000000000000000000, 0.000000000000000000 ) ) ;
#4594=CARTESIAN_POINT ( 'NONE',  ( -31.23437356469425907, 1523.382868172864164, 222.8968241038848248 ) ) ;
#4595=CARTESIAN_POINT ( 'NONE',  ( 17.84338787571943996, 1523.481610426287716, 237.8836641337660467 ) ) ;
#4624=CARTESIAN_POINT ( 'NONE',  ( -16.81464677261302754, 1526.382868172863937, 234.5384874912344344 ) ) ;
#4626=VERTEX_POINT ( 'NONE', #85345 ) ;
#4636=EDGE_LOOP ( 'NONE', ( #19188, #39513, #92344, #51745 ) ) ;
#4638=ORIENTED_EDGE ( 'NONE', *, *, #56372, .T. ) ;
#4639=DIRECTION ( 'NONE',  ( 0.9510565162951518658, 0.000000000000000000, -0.3090169943749528914 ) ) ;
#4640=B_SPLINE_CURVE_WITH_KNOTS ( 'NONE', 3,
 ( #21411, #99223, #80803, #81328, #72417, #6287, #13562, #97603, #39341, #55620 ),
 .UNSPECIFIED., .F., .F.,
 ( 4, 2, 2, 2, 4 ),
 ( 2.797157557069881010E-17, 0.0007406479101618366166, 0.001481295820323645261, 0.002221943730485453905, 0.002962591640647262332 ),
 .UNSPECIFIED. ) ;
#4651=CARTESIAN_POINT ( 'NONE',  ( -20.38673671613278771, 1525.878013734320575, 182.1228282333744914 ) ) ;
#4657=EDGE_CURVE ( 'NONE', #83547, #40664, #20996, .T. ) ;
#4665=CARTESIAN_POINT ( 'NONE',  ( -2.273033093151318962, 1525.821544997590308, 177.3097463090895474 ) ) ;
#4699=CARTESIAN_POINT ( 'NONE',  ( -19.92151515271921980, 1526.208281990535852, 184.7237256173605431 ) ) ;
#4727=LINE ( 'NONE', #73050, #1617 ) ;
#4730=FACE_OUTER_BOUND ( 'NONE', #16698, .T. ) ;
#4740=ORIENTED_EDGE ( 'NONE', *, *, #95366, .F. ) ;
#4747=DIRECTION ( 'NONE',  ( 0.000000000000000000, 1.000000000000000000, 0.000000000000000000 ) ) ;
#4770=CARTESIAN_POINT ( 'NONE',  ( -30.51923195337130679, 1524.059547553518769, 221.8697090587693879 ) ) ;
#4780=FACE_OUTER_BOUND ( 'NONE', #40171, .T. ) ;
#4808=ORIENTED_EDGE ( 'NONE', *, *, #14876, .F. ) ;
#4809=CARTESIAN_POINT ( 'NONE',  ( -21.12212911287049977, 1512.187213306747481, 182.4210318429776976 ) ) ;
#4813=CARTESIAN_POINT ( 'NONE',  ( -17.73225504275565712, 1524.152349020271004, 237.7705388627552452 ) ) ;
#4816=CARTESIAN_POINT ( 'NONE',  ( -2.865545859819519148, 1525.651285554128663, 241.1072462093984825 ) ) ;
#4831=ORIENTED_EDGE ( 'NONE', *, *, #70025, .F. ) ;
#4833=DIRECTION ( 'NONE',  ( 0.4090087482554252696, 0.000000000000000000, -0.9125304618753996566 ) ) ;
#4839=FACE_OUTER_BOUND ( 'NONE', #39781, .T. ) ;
#4841=VECTOR ( 'NONE', #104644, 1000.000000000000000 ) ;
#4845=CARTESIAN_POINT ( 'NONE',  ( -19.37182493330903554, 1526.345556099435726, 185.3206052367970358 ) ) ;
#4848=CARTESIAN_POINT ( 'NONE',  ( 34.18677586421183179, 1522.382868172863937, 198.4504086008745389 ) ) ;
#4851=ORIENTED_EDGE ( 'NONE', *, *, #79634, .T. ) ;
#4853=EDGE_CURVE ( 'NONE', #91781, #5224, #285, .T. ) ;
#4858=CARTESIAN_POINT ( 'NONE',  ( 0.000000000000000000, 1524.340287715038357, 209.1218459616979999 ) ) ;
#4859=CARTESIAN_POINT ( 'NONE',  ( -14.22993178683297266, 1512.187213306747481, 236.2420368605362455 ) ) ;
#4862=DIRECTION ( 'NONE',  ( 0.5032920991128869703, 0.8641163480518950779, 0.000000000000000000 ) ) ;
#4868=ORIENTED_EDGE ( 'NONE', *, *, #109812, .F. ) ;
#4871=CIRCLE ( 'NONE', #67483, 1.000000000000000888 ) ;
#4876=DIRECTION ( 'NONE',  ( 0.8090169943749507819, -0.000000000000000000, 0.5877852522924685852 ) ) ;
#4880=ORIENTED_EDGE ( 'NONE', *, *, #70826, .T. ) ;
#4899=EDGE_CURVE ( 'NONE', #81284, #7253, #83585, .T. ) ;
#4901=CARTESIAN_POINT ( 'NONE',  ( -32.85805783624297760, 1523.678648413191695, 217.1983043299907763 ) ) ;
#4902=CARTESIAN_POINT ( 'NONE',  ( 32.02808312589922224, 1512.187213306747481, 219.9649204700462235 ) ) ;
#4910=CARTESIAN_POINT ( 'NONE',  ( 32.02808312589916540, 1512.187213306747481, 198.2787714533495489 ) ) ;
#4913=DIRECTION ( 'NONE',  ( 0.7414773880254664773, 0.000000000000000000, -0.6709778558543730842 ) ) ;
#4917=FACE_OUTER_BOUND ( 'NONE', #83327, .T. ) ;
#4918=CARTESIAN_POINT ( 'NONE',  ( -18.69816095120789612, 1522.382868172863937, 183.3860352823957953 ) ) ;
#4920=AXIS2_PLACEMENT_3D ( 'NONE', #49390, #14667, #75694 ) ;
#4928=B_SPLINE_CURVE_WITH_KNOTS ( 'NONE', 3,
 ( #87832, #44164, #9443, #104610 ),
 .UNSPECIFIED., .F., .F.,
 ( 4, 4 ),
 ( 0.000000000000000000, 0.0002220129587134778832 ),
 .UNSPECIFIED. ) ;
#4931=CARTESIAN_POINT ( 'NONE',  ( -16.66231036550740541, 1523.604703353109699, 180.4882076302515372 ) ) ;
#4934=CARTESIAN_POINT ( 'NONE',  ( -21.83863729849021951, 1523.580204110583736, 183.2673815993471464 ) ) ;
#4939=ORIENTED_EDGE ( 'NONE', *, *, #76019, .F. ) ;
#4943=CARTESIAN_POINT ( 'NONE',  ( 18.19590854888146580, 1501.977400791986611, 180.0410247165184217 ) ) ;
#4948=CARTESIAN_POINT ( 'NONE',  ( -30.61443310237114446, 1523.382868172864164, 221.8243310972803783 ) ) ;
#4950=CIRCLE ( 'NONE', #81842, 33.13701971169416538 ) ;
#4955=CARTESIAN_POINT ( 'NONE',  ( 32.38114538885255200, 1523.604703353109699, 216.1203639561429100 ) ) ;
#4958=EDGE_CURVE ( 'NONE', #94153, #88502, #4871, .T. ) ;
#4961=CARTESIAN_POINT ( 'NONE',  ( -31.88717309313515713, 1525.425665131969481, 217.0217438353934369 ) ) ;
#4962=ORIENTED_EDGE ( 'NONE', *, *, #64747, .T. ) ;
#4969=CARTESIAN_POINT ( 'NONE',  ( 1.484157417262786494, 1526.349684470114653, 178.3401290187298684 ) ) ;
#4970=CARTESIAN_POINT ( 'NONE',  ( 2.620401159596264851, 1523.462669333490567, 242.1631858338582788 ) ) ;
#4977=FACE_OUTER_BOUND ( 'NONE', #60016, .T. ) ;
#4978=VERTEX_POINT ( 'NONE', #51094 ) ;
#4981=CARTESIAN_POINT ( 'NONE',  ( 17.07724394729159911, 1524.330813522192102, 237.1903650275838800 ) ) ;
#5002=DIRECTION ( 'NONE',  ( 0.000000000000000000, 1.000000000000000000, 0.000000000000000000 ) ) ;
#5004=ORIENTED_EDGE ( 'NONE', *, *, #54592, .F. ) ;
#5027=EDGE_CURVE ( 'NONE', #38078, #23627, #85342, .T. ) ;
#5032=AXIS2_PLACEMENT_3D ( 'NONE', #93054, #16327, #84651 ) ;
#5040=VERTEX_POINT ( 'NONE', #84123 ) ;
#5069=CARTESIAN_POINT ( 'NONE',  ( -21.38516915557943321, 1522.382868172863937, 237.8497028174240313 ) ) ;
#5079=CARTESIAN_POINT ( 'NONE',  ( 29.30029655192931770, 1525.907212628473872, 221.3719603026171114 ) ) ;
#5082=CARTESIAN_POINT ( 'NONE',  ( 20.49599333844834348, 1525.960063244517187, 184.3798832129035077 ) ) ;
#5085=CARTESIAN_POINT ( 'NONE',  ( 32.02808312589922224, 1512.187213306747481, 221.9649204700462235 ) ) ;
#5090=CARTESIAN_POINT ( 'NONE',  ( 18.88880210473194765, 1524.667648926078982, 179.4140113511355423 ) ) ;
#5097=CARTESIAN_POINT ( 'NONE',  ( -16.49279218151803050, 1525.408327360769363, 181.2883303505538493 ) ) ;
#5108=CARTESIAN_POINT ( 'NONE',  ( 17.84338787571921614, 1523.481610426287716, 180.3600277896298110 ) ) ;
#5112=CARTESIAN_POINT ( 'NONE',  ( 1.488474718485413906, 1526.348417187221685, 178.3303222095514400 ) ) ;
#5137=CIRCLE ( 'NONE', #60636, 1.000000000000000888 ) ;
#5169=ADVANCED_FACE ( 'NONE', ( #29728 ), #52169, .T. ) ;
#5181=ORIENTED_EDGE ( 'NONE', *, *, #70326, .T. ) ;
#5183=AXIS2_PLACEMENT_3D ( 'NONE', #103286, #110608, #16514 ) ;
#5194=CARTESIAN_POINT ( 'NONE',  ( -21.38516915558021125, 1522.906561336852519, 180.3939891059724516 ) ) ;
#5197=CARTESIAN_POINT ( 'NONE',  ( 16.16632277704800558, 1511.187213306747708, 236.8966194768523508 ) ) ;
#5201=AXIS2_PLACEMENT_3D ( 'NONE', #49841, #85612, #75601 ) ;
#5208=CARTESIAN_POINT ( 'NONE',  ( 19.37374569213924502, 1526.382868172863937, 183.8768763279539655 ) ) ;
#5210=ORIENTED_EDGE ( 'NONE', *, *, #75298, .T. ) ;
#5223=CIRCLE ( 'NONE', #83939, 0.9999999999999930056 ) ;
#5224=VERTEX_POINT ( 'NONE', #21848 ) ;
#5227=CARTESIAN_POINT ( 'NONE',  ( -32.85805783624300602, 1523.678648413191695, 217.1983043299907763 ) ) ;
#5242=DIRECTION ( 'NONE',  ( -0.000000000000000000, -1.000000000000000000, -0.000000000000000000 ) ) ;
#5247=CARTESIAN_POINT ( 'NONE',  ( -31.18497486287767728, 1524.152349020271004, 221.8763673812615878 ) ) ;
#5251=CARTESIAN_POINT ( 'NONE',  ( 31.65139097221404541, 1525.320849883639767, 216.1854601993777294 ) ) ;
#5258=EDGE_CURVE ( 'NONE', #49199, #29269, #2470, .T. ) ;
#5272=CIRCLE ( 'NONE', #35641, 2.000000000000001776 ) ;
#5296=CARTESIAN_POINT ( 'NONE',  ( 21.55808780551086556, 1523.844782250846038, 234.2610829425819361 ) ) ;
#5300=DIRECTION ( 'NONE',  ( 0.000000000000000000, 1.000000000000000000, 0.000000000000000000 ) ) ;
#5302=CARTESIAN_POINT ( 'NONE',  ( -29.86461515634922037, 1525.960063244517187, 197.2746849027940641 ) ) ;
#5319=ORIENTED_EDGE ( 'NONE', *, *, #102056, .T. ) ;
#5338=VECTOR ( 'NONE', #14091, 1000.000000000000000 ) ;
#5349=CARTESIAN_POINT ( 'NONE',  ( 31.81407709660777883, 1522.382868172863937, 221.9534378623329474 ) ) ;
#5355=CARTESIAN_POINT ( 'NONE',  ( 21.83550407203919974, 1523.678648413191695, 234.9693198511250785 ) ) ;
#5366=CARTESIAN_POINT ( 'NONE',  ( 20.39893125378086580, 1526.069472839386208, 185.1113182959254857 ) ) ;
#5373=CARTESIAN_POINT ( 'NONE',  ( 32.10254378951870535, 1525.211473355384896, 201.2198347410968893 ) ) ;
#5377=CARTESIAN_POINT ( 'NONE',  ( -32.38114538885259464, 1523.604703353109699, 202.1233279672532888 ) ) ;
#5388=ORIENTED_EDGE ( 'NONE', *, *, #73718, .T. ) ;
#5411=CARTESIAN_POINT ( 'NONE',  ( 16.50400130224771544, 1525.907212628473644, 236.2546788475581820 ) ) ;
#5426=CIRCLE ( 'NONE', #7185, 2.000000000000009770 ) ;
#5429=EDGE_LOOP ( 'NONE', ( #19653, #94004, #43352, #4868, #80229 ) ) ;
#5444=CARTESIAN_POINT ( 'NONE',  ( -17.29393938232498229, 1523.621879633028811, 180.8572348224460882 ) ) ;
#5453=AXIS2_PLACEMENT_3D ( 'NONE', #71828, #2406, #2953 ) ;
#5456=CARTESIAN_POINT ( 'NONE',  ( 2.372478608332516892, 1522.382868172863937, 174.8996806668726549 ) ) ;
#5462=ORIENTED_EDGE ( 'NONE', *, *, #43482, .F. ) ;
#5493=FACE_OUTER_BOUND ( 'NONE', #7590, .T. ) ;
#5498=B_SPLINE_CURVE_WITH_KNOTS ( 'NONE', 3,
 ( #43797, #104806, #43255, #44929, #105362, #103128 ),
 .UNSPECIFIED., .F., .F.,
 ( 4, 2, 4 ),
 ( -1.285435071108283616E-05, 0.001079388306740611128, 0.002171630964192305339 ),
 .UNSPECIFIED. ) ;
#5514=ADVANCED_FACE ( 'NONE', ( #44212 ), #90706, .T. ) ;
#5548=CARTESIAN_POINT ( 'NONE',  ( 18.69816095120750532, 1526.382868172863937, 183.3860352823955679 ) ) ;
#5550=DIRECTION ( 'NONE',  ( 0.000000000000000000, 0.000000000000000000, -1.000000000000000000 ) ) ;
#5582=CARTESIAN_POINT ( 'NONE',  ( -32.37018134260392799, 1511.187213306747708, 218.0712926453366833 ) ) ;
#5584=ORIENTED_EDGE ( 'NONE', *, *, #89323, .T. ) ;
#5587=EDGE_CURVE ( 'NONE', #95653, #19317, #64329, .T. ) ;
#5591=ADVANCED_FACE ( 'NONE', ( #97354 ), #73829, .T. ) ;
#5614=CARTESIAN_POINT ( 'NONE',  ( 29.79244380917030455, 1525.556090473947052, 196.8434936746641881 ) ) ;
#5617=CIRCLE ( 'NONE', #12732, 2.000000000000001776 ) ;
#5619=EDGE_CURVE ( 'NONE', #37975, #94335, #103323, .T. ) ;
#5625=ADVANCED_FACE ( 'NONE', ( #81100 ), #13324, .T. ) ;
#5632=VECTOR ( 'NONE', #96233, 1000.000000000000114 ) ;
#5638=VECTOR ( 'NONE', #55237, 1000.000000000000000 ) ;
#5642=EDGE_CURVE ( 'NONE', #83952, #99467, #48065, .T. ) ;
#5649=ADVANCED_FACE ( 'NONE', ( #90044, #31250 ), #73264, .F. ) ;
#5651=CARTESIAN_POINT ( 'NONE',  ( 0.000000000000000000, 1522.051704408389924, 233.8211094035767985 ) ) ;
#5654=FACE_OUTER_BOUND ( 'NONE', #94713, .T. ) ;
#5656=DIRECTION ( 'NONE',  ( -0.000000000000000000, -1.000000000000000000, -0.000000000000000000 ) ) ;
#5664=CARTESIAN_POINT ( 'NONE',  ( -16.48227125551525418, 1525.651285554130027, 181.5607879932552464 ) ) ;
#5678=CARTESIAN_POINT ( 'NONE',  ( -17.07724394728933248, 1524.330813522192102, 237.1903650275824589 ) ) ;
#5683=CARTESIAN_POINT ( 'NONE',  ( 32.28466283162156714, 1512.187213306747481, 219.1752493337713190 ) ) ;
#5684=EDGE_LOOP ( 'NONE', ( #12010, #46230, #77091 ) ) ;
#5703=CYLINDRICAL_SURFACE ( 'NONE', #55438, 2.000000000000003997 ) ;
#5709=ADVANCED_FACE ( 'NONE', ( #57583 ), #67562, .T. ) ;
#5711=ORIENTED_EDGE ( 'NONE', *, *, #24212, .T. ) ;
#5737=CARTESIAN_POINT ( 'NONE',  ( -2.470168522031893854, 1523.481610118013577, 242.8787258960506961 ) ) ;
#5740=CARTESIAN_POINT ( 'NONE',  ( 30.04019103850634664, 1524.756004293092019, 222.3084691776629711 ) ) ;
#5743=ORIENTED_EDGE ( 'NONE', *, *, #42395, .F. ) ;
#5750=VERTEX_POINT ( 'NONE', #67088 ) ;
#5754=CARTESIAN_POINT ( 'NONE',  ( -1.491506560153236904, 1511.187213306747708, 242.6732489767341576 ) ) ;
#5760=CARTESIAN_POINT ( 'NONE',  ( -21.61975802671013369, 1524.130440953581001, 183.7557183496595599 ) ) ;
#5763=CARTESIAN_POINT ( 'NONE',  ( 2.472529913803022783, 1523.678648413191695, 175.3762130535718597 ) ) ;
#5771=CARTESIAN_POINT ( 'NONE',  ( -17.19739463999606599, 1525.960063244516959, 236.2603809477411971 ) ) ;
#5776=DIRECTION ( 'NONE',  ( 0.000000000000000000, 0.000000000000000000, 1.000000000000000000 ) ) ;
#5783=CARTESIAN_POINT ( 'NONE',  ( 17.19739463999641416, 1525.960063244516959, 181.9833109756548879 ) ) ;
#5785=ADVANCED_FACE ( 'NONE', ( #19260 ), #69405, .T. ) ;
#5788=CARTESIAN_POINT ( 'NONE',  ( 20.79738390328718367, 1512.187213306747481, 181.2030061003470394 ) ) ;
#5789=VERTEX_POINT ( 'NONE', #97104 ) ;
#5792=DIRECTION ( 'NONE',  ( 0.000000000000000000, 1.000000000000000000, 0.000000000000000000 ) ) ;
#5805=EDGE_CURVE ( 'NONE', #83932, #72812, #42512, .T. ) ;
#5806=FACE_OUTER_BOUND ( 'NONE', #14080, .T. ) ;
#5814=CARTESIAN_POINT ( 'NONE',  ( -30.01999388067554619, 1525.848198008145346, 221.1300202120172003 ) ) ;
#5886=CARTESIAN_POINT ( 'NONE',  ( 28.72841836131054194, 1526.333389947990099, 198.1146668274930107 ) ) ;
#5890=CARTESIAN_POINT ( 'NONE',  ( -22.04555908422410582, 1524.082740465118377, 233.7638702259614263 ) ) ;
#5905=DIRECTION ( 'NONE',  ( 0.8672669759446630655, 0.000000000000000000, -0.4978433412588735285 ) ) ;
#5908=EDGE_LOOP ( 'NONE', ( #82449, #56903, #10950, #27179 ) ) ;
#5931=CARTESIAN_POINT ( 'NONE',  ( 32.85805783624304155, 1523.678648413191695, 201.0453875934054508 ) ) ;
#5947=VERTEX_POINT ( 'NONE', #64070 ) ;
#5950=CARTESIAN_POINT ( 'NONE',  ( -20.49599333844828664, 1525.960063244516959, 233.8638087104926058 ) ) ;
#5955=DIRECTION ( 'NONE',  ( 0.000000000000000000, 0.000000000000000000, 1.000000000000000000 ) ) ;
#5980=ORIENTED_EDGE ( 'NONE', *, *, #33687, .F. ) ;
#6001=AXIS2_PLACEMENT_3D ( 'NONE', #71815, #63404, #78520 ) ;
#6008=DIRECTION ( 'NONE',  ( 0.000000000000000000, 1.000000000000000000, 0.000000000000000000 ) ) ;
#6018=CARTESIAN_POINT ( 'NONE',  ( -17.84338787571901364, 1523.481610426287716, 237.8836641337663309 ) ) ;
#6036=EDGE_CURVE ( 'NONE', #97770, #67358, #53252, .T. ) ;
#6059=CARTESIAN_POINT ( 'NONE',  ( -30.31940284292399923, 1523.382868172864164, 222.4933038710547635 ) ) ;
#6089=CARTESIAN_POINT ( 'NONE',  ( -22.07680858347428909, 1523.847233649538339, 184.4451117503444664 ) ) ;
#6092=CARTESIAN_POINT ( 'NONE',  ( 31.44837959398582328, 1511.187213306747708, 197.3353852117981262 ) ) ;
#6102=CARTESIAN_POINT ( 'NONE',  ( 30.37359097063795588, 1526.143142182265819, 201.3152257445537714 ) ) ;
#6109=FACE_OUTER_BOUND ( 'NONE', #105250, .T. ) ;
#6125=CARTESIAN_POINT ( 'NONE',  ( -31.23437356469455040, 1511.187213306747708, 195.3468678195118287 ) ) ;
#6129=ORIENTED_EDGE ( 'NONE', *, *, #52429, .T. ) ;
#6166=ORIENTED_EDGE ( 'NONE', *, *, #45039, .F. ) ;
#6175=DIRECTION ( 'NONE',  ( -0.000000000000000000, 1.000000000000000000, -0.000000000000000000 ) ) ;
#6179=CARTESIAN_POINT ( 'NONE',  ( 31.92108011125350231, 1511.187213306747708, 220.9591791661896139 ) ) ;
#6181=AXIS2_PLACEMENT_3D ( 'NONE', #52948, #36138, #2560 ) ;
#6183=CARTESIAN_POINT ( 'NONE',  ( -21.84020450222019250, 1501.977400791986611, 234.9798068779743403 ) ) ;
#6192=EDGE_LOOP ( 'NONE', ( #12769, #72333, #88301, #56256, #29573 ) ) ;
#6204=CARTESIAN_POINT ( 'NONE',  ( -20.92767404034479028, 1511.187213306747708, 235.3888156262297571 ) ) ;
#6207=CARTESIAN_POINT ( 'NONE',  ( 2.472529913803023227, 1523.678648413191695, 242.8674788698241400 ) ) ;
#6216=ORIENTED_EDGE ( 'NONE', *, *, #60493, .T. ) ;
#6236=VECTOR ( 'NONE', #42122, 999.9999999999998863 ) ;
#6239=VECTOR ( 'NONE', #25609, 1000.000000000000000 ) ;
#6241=EDGE_LOOP ( 'NONE', ( #67711, #37297, #18313, #71605, #62776 ) ) ;
#6253=EDGE_CURVE ( 'NONE', #4626, #43885, #108696, .T. ) ;
#6255=CYLINDRICAL_SURFACE ( 'NONE', #91173, 2.000000000000009770 ) ;
#6268=CARTESIAN_POINT ( 'NONE',  ( -18.02257621027615642, 1526.382868172863937, 182.8951942368373977 ) ) ;
#6286=EDGE_LOOP ( 'NONE', ( #78337, #645, #104751, #38738 ) ) ;
#6287=CARTESIAN_POINT ( 'NONE',  ( -17.55387852034892049, 1524.816846803860926, 180.7603862146448250 ) ) ;
#6290=EDGE_CURVE ( 'NONE', #16710, #105489, #106925, .T. ) ;
#6291=VECTOR ( 'NONE', #61511, 1000.000000000000114 ) ;
#6292=LINE ( 'NONE', #5754, #20381 ) ;
#6304=ADVANCED_FACE ( 'NONE', ( #9632 ), #105111, .T. ) ;
#6313=CARTESIAN_POINT ( 'NONE',  ( -2.165176160184186571, 1526.186458717538699, 177.9542909903756538 ) ) ;
#6329=EDGE_CURVE ( 'NONE', #37474, #77339, #10306, .T. ) ;
#6331=AXIS2_PLACEMENT_3D ( 'NONE', #103287, #27165, #330 ) ;
#6354=CARTESIAN_POINT ( 'NONE',  ( 32.70818033930520841, 1524.201670966336224, 217.1264371928152457 ) ) ;
#6362=CARTESIAN_POINT ( 'NONE',  ( 31.34137657934019927, 1523.382868172864164, 221.9025654077410081 ) ) ;
#6398=SHAPE_REPRESENTATION_RELATIONSHIP ( 'NONE' , 'NONE' ,  #10812, #13206 ) ;
#6405=ORIENTED_EDGE ( 'NONE', *, *, #9651, .T. ) ;
#6434=EDGE_CURVE ( 'NONE', #19317, #36910, #47879, .T. ) ;
#6437=CARTESIAN_POINT ( 'NONE',  ( 29.30029655192928928, 1525.907212628473644, 196.8717316207784620 ) ) ;
#6438=CARTESIAN_POINT ( 'NONE',  ( -156.6846457583352503, 1524.382868172863937, 77.25240589482224607 ) ) ;
#6444=DIRECTION ( 'NONE',  ( 0.000000000000000000, 0.8286769424886414326, -0.5597271880011518430 ) ) ;
#6448=CARTESIAN_POINT ( 'NONE',  ( 31.34137657934008558, 1523.382868172864164, 196.3411265156547358 ) ) ;
#6455=CARTESIAN_POINT ( 'NONE',  ( -19.53786426059057746, 1511.187213306747708, 181.5239794925695946 ) ) ;
#6457=CARTESIAN_POINT ( 'NONE',  ( 29.78220350812352990, 1526.382868172863709, 221.7347658002323953 ) ) ;
#6485=CARTESIAN_POINT ( 'NONE',  ( 32.86802468386292730, 1523.382868172864164, 217.2040256693915410 ) ) ;
#6488=ORIENTED_EDGE ( 'NONE', *, *, #15968, .T. ) ;
#6493=ORIENTED_EDGE ( 'NONE', *, *, #49415, .T. ) ;
#6495=CARTESIAN_POINT ( 'NONE',  ( -19.30300490007669367, 1526.348417187222140, 233.1578084719505171 ) ) ;
#6500=DIRECTION ( 'NONE',  ( 0.000000000000000000, 0.000000000000000000, 1.000000000000000000 ) ) ;
#6508=AXIS2_PLACEMENT_3D ( 'NONE', #33420, #75996, #67617 ) ;
#6549=DIRECTION ( 'NONE',  ( 0.000000000000000000, 0.000000000000000000, 1.000000000000000000 ) ) ;
#6555=CARTESIAN_POINT ( 'NONE',  ( 3.246772394788723481, 1511.187213306747708, 241.0944358625217774 ) ) ;
#6563=AXIS2_PLACEMENT_3D ( 'NONE', #30992, #38288, #90337 ) ;
#6574=CARTESIAN_POINT ( 'NONE',  ( 21.83550407203921040, 1523.678648413191695, 234.9693198511251069 ) ) ;
#6591=CARTESIAN_POINT ( 'NONE',  ( 21.84020450222037724, 1501.977400791986611, 183.2638850454218016 ) ) ;
#6596=CARTESIAN_POINT ( 'NONE',  ( 0.000000000000000000, 1523.382868172864164, 209.1218459616979999 ) ) ;
#6603=DIRECTION ( 'NONE',  ( 0.000000000000000000, 1.000000000000000000, 0.000000000000000000 ) ) ;
#6626=DIRECTION ( 'NONE',  ( 0.000000000000000000, 0.000000000000000000, 1.000000000000000000 ) ) ;
#6651=DIRECTION ( 'NONE',  ( -0.3090169943749582204, -0.000000000000000000, -0.9510565162951499785 ) ) ;
#6653=CARTESIAN_POINT ( 'NONE',  ( 32.38845791999495560, 1523.382868172864164, 202.1182848005512085 ) ) ;
#6675=ORIENTED_EDGE ( 'NONE', *, *, #27442, .F. ) ;
#6691=ORIENTED_EDGE ( 'NONE', *, *, #74662, .F. ) ;
#6724=DIRECTION ( 'NONE',  ( 1.000000000000000000, 0.000000000000000000, 0.000000000000000000 ) ) ;
#6727=DIRECTION ( 'NONE',  ( 0.000000000000000000, 0.000000000000000000, 1.000000000000000000 ) ) ;
#6747=CARTESIAN_POINT ( 'NONE',  ( -21.83550407203883736, 1523.678648413191695, 234.9693198511253627 ) ) ;
#6749=CIRCLE ( 'NONE', #22877, 1.000000000000000888 ) ;
#6755=CARTESIAN_POINT ( 'NONE',  ( -19.67623451925489775, 1525.581535527370761, 237.1855307018975054 ) ) ;
#6768=DIRECTION ( 'NONE',  ( -0.4090087482554184417, 0.000000000000000000, 0.9125304618754027652 ) ) ;
#6774=VECTOR ( 'NONE', #20623, 1000.000000000000000 ) ;
#6778=CIRCLE ( 'NONE', #12384, 1.000000000000000888 ) ;
#6825=VERTEX_POINT ( 'NONE', #92636 ) ;
#6841=CARTESIAN_POINT ( 'NONE',  ( 1.491506560153237793, 1511.187213306747708, 175.5704429466618421 ) ) ;
#6848=ORIENTED_EDGE ( 'NONE', *, *, #33831, .F. ) ;
#6863=AXIS2_PLACEMENT_3D ( 'NONE', #11598, #29485, #63681 ) ;
#6868=CIRCLE ( 'NONE', #5032, 1.000000000000000888 ) ;
#6871=EDGE_CURVE ( 'NONE', #6988, #100587, #84886, .T. ) ;
#6885=CARTESIAN_POINT ( 'NONE',  ( -31.34137657934027388, 1501.977400791986611, 196.3411265156551906 ) ) ;
#6899=EDGE_CURVE ( 'NONE', #56418, #10960, #95872, .T. ) ;
#6907=EDGE_CURVE ( 'NONE', #71433, #108182, #46276, .T. ) ;
#6946=ORIENTED_EDGE ( 'NONE', *, *, #78980, .F. ) ;
#6950=VECTOR ( 'NONE', #66871, 1000.000000000000000 ) ;
#6958=FACE_OUTER_BOUND ( 'NONE', #84212, .T. ) ;
#6960=TOROIDAL_SURFACE ( 'NONE', #96319, 32.13701971169416538, 1.000000000000000000 ) ;
#6975=CIRCLE ( 'NONE', #62409, 1.000000000000000888 ) ;
#6984=CARTESIAN_POINT ( 'NONE',  ( -21.82415348264071753, 1524.756004293092019, 233.6168747274685700 ) ) ;
#6988=VERTEX_POINT ( 'NONE', #67579 ) ;
#7000=CARTESIAN_POINT ( 'NONE',  ( 31.40702543711093497, 1523.611961620354123, 221.9096305968278671 ) ) ;
#7005=AXIS2_PLACEMENT_3D ( 'NONE', #80933, #4231, #38365 ) ;
#7014=VECTOR ( 'NONE', #48384, 1000.000000000000000 ) ;
#7032=CARTESIAN_POINT ( 'NONE',  ( 16.48231804958387059, 1525.661276915132476, 181.5746648898756348 ) ) ;
#7034=EDGE_CURVE ( 'NONE', #92642, #40565, #91648, .T. ) ;
#7040=ORIENTED_EDGE ( 'NONE', *, *, #102955, .T. ) ;
#7044=ORIENTED_EDGE ( 'NONE', *, *, #97353, .T. ) ;
#7064=ORIENTED_EDGE ( 'NONE', *, *, #83873, .F. ) ;
#7076=DIRECTION ( 'NONE',  ( -0.000000000000000000, -1.000000000000000000, -0.000000000000000000 ) ) ;
#7080=CARTESIAN_POINT ( 'NONE',  ( 2.485517042439642221, 1524.599984580802357, 242.5124281696222965 ) ) ;
#7083=ORIENTED_EDGE ( 'NONE', *, *, #54592, .T. ) ;
#7102=AXIS2_PLACEMENT_3D ( 'NONE', #12045, #30492, #45680 ) ;
#7111=CIRCLE ( 'NONE', #109032, 0.9999999999999880096 ) ;
#7129=EDGE_CURVE ( 'NONE', #77376, #31615, #18258, .T. ) ;
#7133=CIRCLE ( 'NONE', #69751, 1.999999999999995559 ) ;
#7142=DIRECTION ( 'NONE',  ( 0.000000000000000000, 1.000000000000000000, 0.000000000000000000 ) ) ;
#7143=CARTESIAN_POINT ( 'NONE',  ( 2.691662542991876794, 1524.776010967675802, 176.4305926583369342 ) ) ;
#7147=CIRCLE ( 'NONE', #28654, 0.9999999999999987788 ) ;
#7155=ORIENTED_EDGE ( 'NONE', *, *, #24852, .F. ) ;
#7165=CARTESIAN_POINT ( 'NONE',  ( -30.31052258194577576, 1523.604703353109699, 222.4930856806593908 ) ) ;
#7166=CARTESIAN_POINT ( 'NONE',  ( 17.61183580542134663, 1523.982201850120191, 180.5695639321423300 ) ) ;
#7173=FACE_OUTER_BOUND ( 'NONE', #86809, .T. ) ;
#7174=AXIS2_PLACEMENT_3D ( 'NONE', #100986, #56804, #108849 ) ;
#7184=FACE_OUTER_BOUND ( 'NONE', #60503, .T. ) ;
#7185=AXIS2_PLACEMENT_3D ( 'NONE', #90101, #5002, #22328 ) ;
#7190=CARTESIAN_POINT ( 'NONE',  ( -2.620401159595194596, 1523.462669333492386, 176.0805060895363852 ) ) ;
#7201=( BOUNDED_CURVE ( )  B_SPLINE_CURVE ( 3, ( #51098, #78501, #85223, #104248 ),
 .UNSPECIFIED., .F., .F. ) 
 B_SPLINE_CURVE_WITH_KNOTS ( ( 4, 4 ),
 ( 4.712388980384689674, 6.283185307179586232 ),
 .UNSPECIFIED. ) 
 CURVE ( )  GEOMETRIC_REPRESENTATION_ITEM ( )  RATIONAL_B_SPLINE_CURVE ( ( 1.000000000000000000, 0.8047378541243649375, 0.8047378541243649375, 1.000000000000000000 ) ) 
 REPRESENTATION_ITEM ( '' )  );
#7204=CARTESIAN_POINT ( 'NONE',  ( 33.36586802512172767, 1512.187213306747481, 201.9069332299488622 ) ) ;
#7216=VECTOR ( 'NONE', #71677, 999.9999999999998863 ) ;
#7234=EDGE_LOOP ( 'NONE', ( #30614, #37440, #98816, #77017, #103197 ) ) ;
#7253=VERTEX_POINT ( 'NONE', #83537 ) ;
#7282=AXIS2_PLACEMENT_3D ( 'NONE', #4594, #29240, #30329 ) ;
#7291=FACE_OUTER_BOUND ( 'NONE', #30719, .T. ) ;
#7292=DIRECTION ( 'NONE',  ( -0.9786619618251657382, 0.000000000000000000, 0.2054769195713179730 ) ) ;
#7293=EDGE_CURVE ( 'NONE', #73940, #72816, #93041, .T. ) ;
#7312=DIRECTION ( 'NONE',  ( 0.06728379684272124683, -0.9969860201949396483, 0.03862338952348206428 ) ) ;
#7316=DIRECTION ( 'NONE',  ( -0.000000000000000000, -1.000000000000000000, -0.000000000000000000 ) ) ;
#7346=ORIENTED_EDGE ( 'NONE', *, *, #59735, .T. ) ;
#7350=CYLINDRICAL_SURFACE ( 'NONE', #102933, 2.000000000000000000 ) ;
#7354=CIRCLE ( 'NONE', #69974, 2.000000000000001776 ) ;
#7362=EDGE_LOOP ( 'NONE', ( #11005, #13102, #31358, #73118, #38631 ) ) ;
#7367=VERTEX_POINT ( 'NONE', #88519 ) ;
#7370=AXIS2_PLACEMENT_3D ( 'NONE', #75224, #56206, #82513 ) ;
#7390=CARTESIAN_POINT ( 'NONE',  ( 21.59396340175304019, 1525.159196711359755, 233.4989680424126561 ) ) ;
#7406=CARTESIAN_POINT ( 'NONE',  ( -21.60819468828554335, 1524.659802833172535, 234.6460983332875685 ) ) ;
#7432=VECTOR ( 'NONE', #9572, 1000.000000000000114 ) ;
#7454=CARTESIAN_POINT ( 'NONE',  ( -20.70484064406366187, 1525.907212628473644, 233.2025904124108706 ) ) ;
#7457=VECTOR ( 'NONE', #34267, 1000.000000000000114 ) ;
#7462=CARTESIAN_POINT ( 'NONE',  ( 16.55387768533850945, 1524.739563915906047, 180.7878331405790675 ) ) ;
#7467=CARTESIAN_POINT ( 'NONE',  ( 17.53704155054290936, 1524.872178180562514, 237.4421490224650313 ) ) ;
#7470=DIRECTION ( 'NONE',  ( 0.9977304882603014180, -0.06733403890946067227, 0.000000000000000000 ) ) ;
#7477=AXIS2_PLACEMENT_3D ( 'NONE', #11984, #55663, #29326 ) ;
#7480=VERTEX_POINT ( 'NONE', #21818 ) ;
#7487=CARTESIAN_POINT ( 'NONE',  ( -18.69816095120789612, 1526.382868172863937, 183.3860352823957953 ) ) ;
#7526=DIRECTION ( 'NONE',  ( -0.3090169943749382919, 2.144236138472229863E-15, 0.9510565162951565288 ) ) ;
#7528=DIRECTION ( 'NONE',  ( -0.4978433412588614271, 0.000000000000000000, 0.8672669759446700599 ) ) ;
#7529=AXIS2_PLACEMENT_3D ( 'NONE', #92724, #28288, #54623 ) ;
#7539=( BOUNDED_SURFACE ( )  B_SPLINE_SURFACE ( 3, 2, ( 
 ( #49576, #58526, #5349 ),
 ( #39509, #56313, #41159 ),
 ( #13723, #40053, #40605 ),
 ( #48478, #74234, #41708 ),
 ( #22668, #7554, #7000 ),
 ( #32208, #14288, #108365 ),
 ( #73682, #82616, #66935 ),
 ( #101043, #64738, #66389 ),
 ( #31646, #65278, #47908 ),
 ( #108916, #6457, #100508 ) ),
 .UNSPECIFIED., .F., .F., .F. ) 
 B_SPLINE_SURFACE_WITH_KNOTS ( ( 4, 2, 2, 2, 4 ),
 ( 3, 3 ),
 ( 0.000000000000000000, 0.3926990816987241395, 0.7853981633974482790, 1.178097245096172418, 1.570796326794896558 ),
 ( 0.000000000000000000, 1.000000000000000000 ),
 .UNSPECIFIED. ) 
 GEOMETRIC_REPRESENTATION_ITEM ( )  RATIONAL_B_SPLINE_SURFACE ( (
 ( 1.000000000000000000, 0.7763623250684322796, 1.000000000000000000),
 ( 1.000000000000000000, 0.7763684247038049602, 1.000000000000000000),
 ( 1.000000000000000000, 0.7746454561793517657, 1.000000000000000000),
 ( 1.000000000000000000, 0.7679730451976943817, 1.000000000000000000),
 ( 1.000000000000000000, 0.7630177051949541545, 1.000000000000000000),
 ( 1.000000000000000000, 0.7504512394525465480, 1.000000000000000000),
 ( 1.000000000000000000, 0.7428408967918798123, 1.000000000000000000),
 ( 1.000000000000000000, 0.7259222650918639719, 1.000000000000000000),
 ( 1.000000000000000000, 0.7166207884813426965, 1.000000000000000000),
 ( 1.000000000000000000, 0.7071067811865868746, 1.000000000000000000) ) ) 
 REPRESENTATION_ITEM ( '' )  SURFACE ( )  );
#7554=CARTESIAN_POINT ( 'NONE',  ( 32.74318896774105525, 1524.667648926078300, 222.0534297170919160 ) ) ;
#7557=AXIS2_PLACEMENT_3D ( 'NONE', #55350, #104632, #71068 ) ;
#7561=CARTESIAN_POINT ( 'NONE',  ( 30.31940284292409515, 1512.187213306747481, 195.7503880523414352 ) ) ;
#7571=CARTESIAN_POINT ( 'NONE',  ( -21.37468300741611316, 1525.408337840050081, 184.8352431113903265 ) ) ;
#7590=EDGE_LOOP ( 'NONE', ( #2326, #71859, #88162, #11047 ) ) ;
#7618=DIRECTION ( 'NONE',  ( 0.3090169943749383474, -0.000000000000000000, -0.9510565162951566398 ) ) ;
#7625=ORIENTED_EDGE ( 'NONE', *, *, #95512, .F. ) ;
#7645=CARTESIAN_POINT ( 'NONE',  ( 20.70484064406359437, 1525.907212628473872, 185.0411015109854134 ) ) ;
#7680=ORIENTED_EDGE ( 'NONE', *, *, #8925, .F. ) ;
#7686=CARTESIAN_POINT ( 'NONE',  ( 3.261863598262784603, 1524.739915903631982, 176.4692008623654829 ) ) ;
#7707=CARTESIAN_POINT ( 'NONE',  ( 20.71343476517511917, 1522.382868172863937, 179.9059455038194812 ) ) ;
#7728=CARTESIAN_POINT ( 'NONE',  ( -21.54116136312493879, 1523.382868172864164, 234.3126182787005689 ) ) ;
#7754=ADVANCED_FACE ( 'NONE', ( #53157 ), #103531, .T. ) ;
#7763=CARTESIAN_POINT ( 'NONE',  ( -2.744860781518600579, 1525.790286462510494, 177.2996071530072300 ) ) ;
#7771=ORIENTED_EDGE ( 'NONE', *, *, #8363, .F. ) ;
#7779=ADVANCED_FACE ( 'NONE', ( #73250 ), #27939, .T. ) ;
#7790=ORIENTED_EDGE ( 'NONE', *, *, #68617, .T. ) ;
#7794=EDGE_LOOP ( 'NONE', ( #49867, #22893, #74763, #96499 ) ) ;
#7800=ADVANCED_FACE ( 'NONE', ( #22254 ), #83843, .T. ) ;
#7825=AXIS2_PLACEMENT_3D ( 'NONE', #110230, #68272, #85023 ) ;
#7835=CARTESIAN_POINT ( 'NONE',  ( -2.425477467415915189, 1523.390106123591067, 175.1521078860136527 ) ) ;
#7836=( BOUNDED_SURFACE ( )  B_SPLINE_SURFACE ( 3, 2, ( 
 ( #86491, #52915, #1398 ),
 ( #88168, #61883, #87047 ),
 ( #52371, #80310, #69732 ),
 ( #27697, #87616, #45077 ),
 ( #3626, #10335, #103851 ),
 ( #37206, #61335, #105515 ),
 ( #79220, #18719, #54582 ),
 ( #44507, #28806, #78654 ),
 ( #36106, #70292, #63003 ),
 ( #36649, #97111, #95999 ) ),
 .UNSPECIFIED., .F., .F., .F. ) 
 B_SPLINE_SURFACE_WITH_KNOTS ( ( 4, 2, 2, 2, 4 ),
 ( 3, 3 ),
 ( 0.000000000000000000, 0.3926990816987241395, 0.7853981633974482790, 1.178097245096172418, 1.570796326794896558 ),
 ( 0.000000000000000000, 1.000000000000000000 ),
 .UNSPECIFIED. ) 
 GEOMETRIC_REPRESENTATION_ITEM ( )  RATIONAL_B_SPLINE_SURFACE ( (
 ( 1.000000000000000000, 0.7763623250684343891, 1.000000000000000000),
 ( 1.000000000000000000, 0.7763684247033950658, 1.000000000000000000),
 ( 1.000000000000000000, 0.7746454561798882255, 1.000000000000000000),
 ( 1.000000000000000000, 0.7679730451971521488, 1.000000000000000000),
 ( 1.000000000000000000, 0.7630177051937461208, 1.000000000000000000),
 ( 1.000000000000000000, 0.7504512394537481423, 1.000000000000000000),
 ( 1.000000000000000000, 0.7428408967937900620, 1.000000000000000000),
 ( 1.000000000000000000, 0.7259222650899548324, 1.000000000000000000),
 ( 1.000000000000000000, 0.7166207884827766605, 1.000000000000000000),
 ( 1.000000000000000000, 0.7071067811865866526, 1.000000000000000000) ) ) 
 REPRESENTATION_ITEM ( '' )  SURFACE ( )  );
#7841=DIRECTION ( 'NONE',  ( 0.000000000000000000, 1.000000000000000000, 0.000000000000000000 ) ) ;
#7854=AXIS2_PLACEMENT_3D ( 'NONE', #65378, #101136, #6549 ) ;
#7868=ORIENTED_EDGE ( 'NONE', *, *, #30820, .T. ) ;
#7896=CARTESIAN_POINT ( 'NONE',  ( 21.60845823726257464, 1524.659148609483054, 234.6463771270923360 ) ) ;
#7953=ADVANCED_FACE ( 'NONE', ( #68725 ), #54806, .T. ) ;
#7975=CARTESIAN_POINT ( 'NONE',  ( 19.53786426059019021, 1512.187213306747481, 181.5239794925693388 ) ) ;
#7989=CARTESIAN_POINT ( 'NONE',  ( 34.18677586421189574, 1522.382868172863937, 219.7932833225211766 ) ) ;
#7996=AXIS2_PLACEMENT_3D ( 'NONE', #10466, #88833, #63659 ) ;
#8009=CARTESIAN_POINT ( 'NONE',  ( 16.54283724222780450, 1524.843178112495707, 180.8452489027513934 ) ) ;
#8014=DIRECTION ( 'NONE',  ( -0.000000000000000000, -1.000000000000000000, -0.000000000000000000 ) ) ;
#8016=DIRECTION ( 'NONE',  ( -0.000000000000000000, -1.000000000000000000, -0.000000000000000000 ) ) ;
#8017=DIRECTION ( 'NONE',  ( 0.5117323852940948159, -0.8591449038673372174, 0.000000000000000000 ) ) ;
#8029=VERTEX_POINT ( 'NONE', #25570 ) ;
#8055=DIRECTION ( 'NONE',  ( -0.000000000000000000, -1.000000000000000000, -0.000000000000000000 ) ) ;
#8057=EDGE_CURVE ( 'NONE', #13119, #42516, #63528, .T. ) ;
#8060=ORIENTED_EDGE ( 'NONE', *, *, #92004, .F. ) ;
#8062=DIRECTION ( 'NONE',  ( -0.1070030146457459225, 0.000000000000000000, -0.9942586961433740322 ) ) ;
#8099=CARTESIAN_POINT ( 'NONE',  ( -19.53786426058999481, 1512.187213306747481, 236.7197124308268030 ) ) ;
#8105=DIRECTION ( 'NONE',  ( -0.05752486295818479839, -0.9969860201949398704, -0.05205540968523020284 ) ) ;
#8111=CARTESIAN_POINT ( 'NONE',  ( -21.14962954805721296, 1525.231909165033585, 184.4343201733738340 ) ) ;
#8112=AXIS2_PLACEMENT_3D ( 'NONE', #109161, #92330, #518 ) ;
#8130=ORIENTED_EDGE ( 'NONE', *, *, #42653, .T. ) ;
#8133=ORIENTED_EDGE ( 'NONE', *, *, #40616, .T. ) ;
#8136=CARTESIAN_POINT ( 'NONE',  ( -30.31940284292427634, 1518.913060387330006, 195.7503880523418616 ) ) ;
#8168=VERTEX_POINT ( 'NONE', #79321 ) ;
#8176=CARTESIAN_POINT ( 'NONE',  ( 32.78250617288038171, 1512.187213306747481, 199.9357095655690841 ) ) ;
#8177=CIRCLE ( 'NONE', #74394, 30.10786454236638576 ) ;
#8178=( BOUNDED_SURFACE ( )  B_SPLINE_SURFACE ( 3, 2, ( 
 ( #1651, #11682, #27378 ),
 ( #105760, #35786, #96244 ),
 ( #104083, #11149, #62118 ),
 ( #95692, #95141, #36326 ),
 ( #69970, #61559, #12223 ),
 ( #46417, #18958, #86736 ),
 ( #97335, #62681, #54267 ),
 ( #104638, #53724, #63231 ),
 ( #53154, #96803, #36880 ),
 ( #105198, #87292, #19519 ) ),
 .UNSPECIFIED., .F., .F., .F. ) 
 B_SPLINE_SURFACE_WITH_KNOTS ( ( 4, 2, 2, 2, 4 ),
 ( 3, 3 ),
 ( 1.570796326794896558, 1.963495408493620697, 2.356194490192344837, 2.748893571891068976, 3.141592653589793116 ),
 ( 0.000000000000000000, 1.000000000000000000 ),
 .UNSPECIFIED. ) 
 GEOMETRIC_REPRESENTATION_ITEM ( )  RATIONAL_B_SPLINE_SURFACE ( (
 ( 1.000000000000000000, 0.7071067811865878738, 1.000000000000000000),
 ( 1.000000000000000000, 0.7166207884821444996, 1.000000000000000000),
 ( 1.000000000000000000, 0.7259222650907969365, 1.000000000000000000),
 ( 1.000000000000000000, 0.7428408967929446272, 1.000000000000000000),
 ( 1.000000000000000000, 0.7504512394529284647, 1.000000000000000000),
 ( 1.000000000000000000, 0.7630177051945691291, 1.000000000000000000),
 ( 1.000000000000000000, 0.7679730451975484984, 1.000000000000000000),
 ( 1.000000000000000000, 0.7746454561794965388, 1.000000000000000000),
 ( 1.000000000000000000, 0.7763684247036931607, 1.000000000000000000),
 ( 1.000000000000000000, 0.7763623250684325017, 1.000000000000000000) ) ) 
 REPRESENTATION_ITEM ( '' )  SURFACE ( )  );
#8185=CARTESIAN_POINT ( 'NONE',  ( -3.347801439296141268, 1512.187213306747481, 176.1543725841967500 ) ) ;
#8203=CARTESIAN_POINT ( 'NONE',  ( -2.596261494520238688, 1525.907212628473644, 240.7735774411713123 ) ) ;
#8211=CARTESIAN_POINT ( 'NONE',  ( 0.000000000000000000, 1522.051704408389924, 209.1218459616979999 ) ) ;
#8224=CARTESIAN_POINT ( 'NONE',  ( 2.214868538355918570, 1525.730671215507982, 176.6953666955783433 ) ) ;
#8225=LINE ( 'NONE', #6591, #89729 ) ;
#8231=FACE_OUTER_BOUND ( 'NONE', #81918, .T. ) ;
#8238=CARTESIAN_POINT ( 'NONE',  ( -32.02808312589908013, 1512.187213306747481, 219.9649204700466782 ) ) ;
#8240=CARTESIAN_POINT ( 'NONE',  ( -1.682117298743253553, 1526.345556099435726, 178.4797647222532930 ) ) ;
#8255=CARTESIAN_POINT ( 'NONE',  ( 32.39315898239710378, 1526.178928173328131, 216.9314351822641243 ) ) ;
#8265=DIRECTION ( 'NONE',  ( -0.000000000000000000, -1.000000000000000000, -0.000000000000000000 ) ) ;
#8266=CARTESIAN_POINT ( 'NONE',  ( -2.372478608332516892, 1522.862737210649811, 243.3440112565233449 ) ) ;
#8269=CARTESIAN_POINT ( 'NONE',  ( -21.84020450222019960, 1523.382868172864164, 234.9798068779743687 ) ) ;
#8270=CARTESIAN_POINT ( 'NONE',  ( -32.28466283162165240, 1522.382868172863937, 199.0684425896249081 ) ) ;
#8305=ADVANCED_FACE ( 'NONE', ( #110023 ), #55777, .T. ) ;
#8309=CARTESIAN_POINT ( 'NONE',  ( -2.599446155150084259, 1525.231909165033812, 176.7177777100700951 ) ) ;
#8325=DIRECTION ( 'NONE',  ( 0.9942586961433741433, 0.000000000000000000, -0.1070030146457454784 ) ) ;
#8333=ORIENTED_EDGE ( 'NONE', *, *, #82212, .T. ) ;
#8353=ORIENTED_EDGE ( 'NONE', *, *, #101981, .T. ) ;
#8354=CARTESIAN_POINT ( 'NONE',  ( -32.38845791999505508, 1523.382868172864164, 202.1182848005516348 ) ) ;
#8363=EDGE_CURVE ( 'NONE', #63441, #50666, #87000, .T. ) ;
#8380=CARTESIAN_POINT ( 'NONE',  ( -2.397475438394535363, 1525.713797967456685, 175.0187375749330272 ) ) ;
#8409=FACE_OUTER_BOUND ( 'NONE', #75817, .T. ) ;
#8413=CARTESIAN_POINT ( 'NONE',  ( 33.23571934791672788, 1511.187213306747708, 219.4842663281462478 ) ) ;
#8424=CARTESIAN_POINT ( 'NONE',  ( -30.61611611310621583, 1526.069472839374157, 216.5565799337567796 ) ) ;
#8429=CARTESIAN_POINT ( 'NONE',  ( -31.10384971727474479, 1525.795403621571268, 216.3488199036669926 ) ) ;
#8433=DIRECTION ( 'NONE',  ( -0.2054769195713187224, -0.000000000000000000, -0.9786619618251655162 ) ) ;
#8441=CYLINDRICAL_SURFACE ( 'NONE', #83764, 1.000000000000000888 ) ;
#8445=SHAPE_DEFINITION_REPRESENTATION ( #53566, #10812 ) ;
#8457=CARTESIAN_POINT ( 'NONE',  ( -16.78480385485633519, 1526.748660780343471, 236.7163225783323526 ) ) ;
#8460=TOROIDAL_SURFACE ( 'NONE', #90715, 2.000000000000000000, 1.000000000000000000 ) ;
#8462=DIRECTION ( 'NONE',  ( -0.7414773880254725835, -1.225281874271767957E-16, -0.6709778558543664229 ) ) ;
#8473=ORIENTED_EDGE ( 'NONE', *, *, #69990, .T. ) ;
#8476=CARTESIAN_POINT ( 'NONE',  ( 22.04556278850125040, 1524.082582765195411, 233.7638865113347038 ) ) ;
#8479=MANIFOLD_SOLID_BREP ( 'Stock-MAS-682-1', #41329 ) ;
#8493=CARTESIAN_POINT ( 'NONE',  ( -21.92026280708428132, 1524.524650307242837, 233.6742115692356094 ) ) ;
#8512=ORIENTED_EDGE ( 'NONE', *, *, #82945, .T. ) ;
#8543=AXIS2_PLACEMENT_3D ( 'NONE', #22574, #109393, #32669 ) ;
#8562=CARTESIAN_POINT ( 'NONE',  ( 2.372478608332516892, 1522.382868172863937, 243.3440112565233449 ) ) ;
#8574=ORIENTED_EDGE ( 'NONE', *, *, #5027, .T. ) ;
#8577=CARTESIAN_POINT ( 'NONE',  ( 21.55491250604723064, 1524.059663615499858, 184.0356616387038002 ) ) ;
#8581=CARTESIAN_POINT ( 'NONE',  ( 30.25425994617009096, 1522.382868172863937, 218.9520509131588994 ) ) ;
#8618=CARTESIAN_POINT ( 'NONE',  ( 19.37374569213924858, 1526.382868172863937, 183.8768763279539655 ) ) ;
#8628=CARTESIAN_POINT ( 'NONE',  ( 29.95988583835885066, 1525.317349363550420, 221.5595150200594787 ) ) ;
#8630=ORIENTED_EDGE ( 'NONE', *, *, #98027, .F. ) ;
#8643=CIRCLE ( 'NONE', #35515, 1.000000000000000888 ) ;
#8658=CARTESIAN_POINT ( 'NONE',  ( -21.95768443299153461, 1524.412455883367329, 184.5445616807625981 ) ) ;
#8660=ORIENTED_EDGE ( 'NONE', *, *, #61831, .F. ) ;
#8661=CARTESIAN_POINT ( 'NONE',  ( 20.06031067115782918, 1526.189899547014420, 185.1817256993992942 ) ) ;
#8666=DIRECTION ( 'NONE',  ( -0.3090169943749382919, -2.144236138472229863E-15, 0.9510565162951565288 ) ) ;
#8673=ADVANCED_FACE ( 'NONE', ( #80758 ), #38710, .T. ) ;
#8681=VERTEX_POINT ( 'NONE', #108146 ) ;
#8694=CARTESIAN_POINT ( 'NONE',  ( 21.84020450222056553, 1512.187213306747481, 234.9798068779740277 ) ) ;
#8699=CYLINDRICAL_SURFACE ( 'NONE', #105167, 1.999999999999998668 ) ;
#8708=EDGE_CURVE ( 'NONE', #43597, #77376, #58399, .T. ) ;
#8721=ORIENTED_EDGE ( 'NONE', *, *, #24671, .F. ) ;
#8723=CARTESIAN_POINT ( 'NONE',  ( -21.83550407203936672, 1523.678648413191695, 183.2743720722710634 ) ) ;
#8738=ORIENTED_EDGE ( 'NONE', *, *, #23524, .T. ) ;
#8745=VECTOR ( 'NONE', #16992, 1000.000000000000114 ) ;
#8754=EDGE_LOOP ( 'NONE', ( #39377, #41102, #105605, #72609 ) ) ;
#8758=ORIENTED_EDGE ( 'NONE', *, *, #67838, .F. ) ;
#8764=LINE ( 'NONE', #60300, #25103 ) ;
#8777=CARTESIAN_POINT ( 'NONE',  ( 2.622430729442982944, 1523.621879633028584, 176.0901726876731175 ) ) ;
#8780=CARTESIAN_POINT ( 'NONE',  ( -34.68852446352314445, 1522.861859112239244, 199.9946320047847053 ) ) ;
#8791=DIRECTION ( 'NONE',  ( 0.9942586961433753645, 0.000000000000000000, -0.1070030146457356945 ) ) ;
#8792=CARTESIAN_POINT ( 'NONE',  ( 32.37018134260395641, 1511.187213306747708, 200.1723992780595438 ) ) ;
#8796=TOROIDAL_SURFACE ( 'NONE', #3487, 1.000000000000000000, 1.000000000000000000 ) ;
#8816=CARTESIAN_POINT ( 'NONE',  ( 2.472529913803022783, 1523.678648413191695, 175.3762130535718597 ) ) ;
#8836=VECTOR ( 'NONE', #64356, 1000.000000000000227 ) ;
#8854=AXIS2_PLACEMENT_3D ( 'NONE', #84412, #56601, #67086 ) ;
#8858=CARTESIAN_POINT ( 'NONE',  ( -3.261946504277382086, 1524.739563915922190, 176.4690228988872320 ) ) ;
#8902=CARTESIAN_POINT ( 'NONE',  ( 30.77259778570388704, 1524.972383263453366, 196.5524048554408409 ) ) ;
#8903=CARTESIAN_POINT ( 'NONE',  ( -19.53786426058999481, 1522.382868172863937, 236.7197124308268030 ) ) ;
#8904=CARTESIAN_POINT ( 'NONE',  ( -16.48231778833706684, 1525.661275128775287, 181.5746610185808834 ) ) ;
#8909=CARTESIAN_POINT ( 'NONE',  ( -32.22536377336284374, 1523.621879633028584, 201.4085774011532806 ) ) ;
#8910=DIRECTION ( 'NONE',  ( -0.3090169943749383474, 0.000000000000000000, 0.9510565162951566398 ) ) ;
#8918=FACE_OUTER_BOUND ( 'NONE', #22344, .T. ) ;
#8925=EDGE_CURVE ( 'NONE', #77302, #83385, #53046, .T. ) ;
#8927=AXIS2_PLACEMENT_3D ( 'NONE', #105724, #2724, #20036 ) ;
#8949=EDGE_CURVE ( 'NONE', #36007, #82949, #56748, .T. ) ;
#8950=CARTESIAN_POINT ( 'NONE',  ( -31.87595007833786553, 1525.042412244735488, 216.1377694412481674 ) ) ;
#8952=ORIENTED_EDGE ( 'NONE', *, *, #84469, .F. ) ;
#8958=B_SPLINE_CURVE_WITH_KNOTS ( 'NONE', 3,
 ( #62933, #98117, #3554, #89726, #20856, #13001, #81312, #22484, #56684, #14102 ),
 .UNSPECIFIED., .F., .F.,
 ( 4, 2, 2, 2, 4 ),
 ( 0.000000000000000000, 0.0007403986298595412272, 0.001480797259719082454, 0.002221195889578623898, 0.002961594519438164909 ),
 .UNSPECIFIED. ) ;
#8961=VECTOR ( 'NONE', #102574, 1000.000000000000000 ) ;
#8963=CARTESIAN_POINT ( 'NONE',  ( -22.75273496409615603, 1512.187213306747481, 183.6728937936775310 ) ) ;
#8968=EDGE_LOOP ( 'NONE', ( #93280, #43730, #95274, #90349 ) ) ;
#9002=VECTOR ( 'NONE', #23161, 1000.000000000000114 ) ;
#9012=AXIS2_PLACEMENT_3D ( 'NONE', #16795, #50999, #84582 ) ;
#9022=AXIS2_PLACEMENT_3D ( 'NONE', #90895, #73009, #100399 ) ;
#9023=CARTESIAN_POINT ( 'NONE',  ( 156.6846457583332892, 1526.382868172863937, 77.25240589481997233 ) ) ;
#9041=CARTESIAN_POINT ( 'NONE',  ( -31.64580750758035066, 1523.313115944345554, 221.9353285379001193 ) ) ;
#9059=CARTESIAN_POINT ( 'NONE',  ( -21.08095450300509555, 1525.506916460691400, 234.2045005059986238 ) ) ;
#9102=CARTESIAN_POINT ( 'NONE',  ( -31.25788889088906686, 1523.954924407801172, 196.3501115357356923 ) ) ;
#9107=AXIS2_PLACEMENT_3D ( 'NONE', #43754, #9583, #61143 ) ;
#9113=CARTESIAN_POINT ( 'NONE',  ( 21.84020450222056908, 1523.382868172864164, 234.9798068779740277 ) ) ;
#9116=VECTOR ( 'NONE', #68148, 1000.000000000000114 ) ;
#9131=CARTESIAN_POINT ( 'NONE',  ( -21.05711716160357838, 1526.748660780343471, 184.6313866553786625 ) ) ;
#9132=EDGE_CURVE ( 'NONE', #30026, #54321, #54879, .T. ) ;
#9155=ADVANCED_FACE ( 'NONE', ( #12291 ), #42614, .T. ) ;
#9168=ORIENTED_EDGE ( 'NONE', *, *, #76837, .T. ) ;
#9182=ORIENTED_EDGE ( 'NONE', *, *, #12447, .T. ) ;
#9195=DIRECTION ( 'NONE',  ( -0.8672669759446666182, 0.000000000000000000, -0.4978433412588673113 ) ) ;
#9231=AXIS2_PLACEMENT_3D ( 'NONE', #86726, #23230, #75324 ) ;
#9236=DIRECTION ( 'NONE',  ( 0.000000000000000000, 1.000000000000000000, 0.000000000000000000 ) ) ;
#9237=CARTESIAN_POINT ( 'NONE',  ( -21.15380500792108975, 1525.425686270225015, 183.9878966353793146 ) ) ;
#9246=CARTESIAN_POINT ( 'NONE',  ( 31.03088476499726411, 1523.982201850120191, 196.3745419238240686 ) ) ;
#9247=DIRECTION ( 'NONE',  ( 0.5030436214085290958, 0.000000000000000000, 0.8642610224695965737 ) ) ;
#9248=DIRECTION ( 'NONE',  ( 0.000000000000000000, 0.000000000000000000, -1.000000000000000000 ) ) ;
#9267=CARTESIAN_POINT ( 'NONE',  ( -0.7251570665222378809, 1526.278758871496620, 241.9800489742292484 ) ) ;
#9280=CARTESIAN_POINT ( 'NONE',  ( -32.28368668151615850, 1524.972383263452684, 201.2030582732907931 ) ) ;
#9287=DIRECTION ( 'NONE',  ( -0.1070030146457285891, 0.000000000000000000, 0.9942586961433760306 ) ) ;
#9293=VECTOR ( 'NONE', #95342, 999.9999999999998863 ) ;
#9298=ORIENTED_EDGE ( 'NONE', *, *, #75055, .F. ) ;
#9302=CIRCLE ( 'NONE', #45062, 1.000000000000009326 ) ;
#9323=CARTESIAN_POINT ( 'NONE',  ( -30.11859361092962573, 1525.055402519452173, 221.6904485361513366 ) ) ;
#9331=EDGE_LOOP ( 'NONE', ( #14216, #40534, #21718, #96011 ) ) ;
#9339=CARTESIAN_POINT ( 'NONE',  ( -19.53786426059057746, 1522.382868172863937, 181.5239794925695946 ) ) ;
#9351=EDGE_CURVE ( 'NONE', #49199, #46121, #60022, .T. ) ;
#9354=CARTESIAN_POINT ( 'NONE',  ( -34.09113935470863055, 1523.429859730330008, 198.4929744671656522 ) ) ;
#9375=DIRECTION ( 'NONE',  ( 0.000000000000000000, 1.000000000000000000, 0.000000000000000000 ) ) ;
#9427=CARTESIAN_POINT ( 'NONE',  ( -2.458536830555473340, 1524.871836253796118, 175.9019916315544094 ) ) ;
#9443=CARTESIAN_POINT ( 'NONE',  ( -22.08523692261532290, 1523.530935881284904, 233.8225055907671788 ) ) ;
#9447=ADVANCED_FACE ( 'NONE', ( #51988 ), #99825, .T. ) ;
#9466=CARTESIAN_POINT ( 'NONE',  ( 29.91208173166741702, 1525.042337199240137, 196.0615906098655898 ) ) ;
#9486=CARTESIAN_POINT ( 'NONE',  ( -3.304926999371979868, 1524.538969332612623, 176.3724890512824004 ) ) ;
#9497=( BOUNDED_CURVE ( )  B_SPLINE_CURVE ( 3, ( #27395, #86756, #61578, #3883 ),
 .UNSPECIFIED., .F., .F. ) 
 B_SPLINE_CURVE_WITH_KNOTS ( ( 4, 4 ),
 ( 4.712388980384689674, 6.283185307179586232 ),
 .UNSPECIFIED. ) 
 CURVE ( )  GEOMETRIC_REPRESENTATION_ITEM ( )  RATIONAL_B_SPLINE_CURVE ( ( 1.000000000000000000, 0.8047378541243649375, 0.8047378541243649375, 1.000000000000000000 ) ) 
 REPRESENTATION_ITEM ( '' )  );
#9501=VERTEX_POINT ( 'NONE', #18351 ) ;
#9505=CARTESIAN_POINT ( 'NONE',  ( -32.05521452193857357, 1525.253996226948402, 217.0243583754457859 ) ) ;
#9519=ORIENTED_EDGE ( 'NONE', *, *, #98132, .F. ) ;
#9524=ORIENTED_EDGE ( 'NONE', *, *, #104087, .F. ) ;
#9528=DIRECTION ( 'NONE',  ( -0.9786619618251632957, 0.000000000000000000, -0.2054769195713296581 ) ) ;
#9543=ORIENTED_EDGE ( 'NONE', *, *, #30975, .F. ) ;
#9564=VERTEX_POINT ( 'NONE', #95634 ) ;
#9568=DIRECTION ( 'NONE',  ( -0.000000000000000000, -1.000000000000000000, -0.000000000000000000 ) ) ;
#9569=DIRECTION ( 'NONE',  ( -0.6709778558543639804, 0.000000000000000000, 0.7414773880254746929 ) ) ;
#9572=DIRECTION ( 'NONE',  ( 0.8672669759446699489, -0.000000000000000000, 0.4978433412588613716 ) ) ;
#9583=DIRECTION ( 'NONE',  ( -0.000000000000000000, -1.000000000000000000, -0.000000000000000000 ) ) ;
#9584=CARTESIAN_POINT ( 'NONE',  ( 0.000000000000000000, 1524.340287715038357, 233.4544294405183678 ) ) ;
#9601=FACE_OUTER_BOUND ( 'NONE', #109689, .T. ) ;
#9609=CARTESIAN_POINT ( 'NONE',  ( 20.71343476517534299, 1522.382868172863937, 238.3377464195763764 ) ) ;
#9613=DIRECTION ( 'NONE',  ( -0.000000000000000000, -1.000000000000000000, -0.000000000000000000 ) ) ;
#9625=CARTESIAN_POINT ( 'NONE',  ( 32.86802468363458729, 1523.481610118014942, 217.2040256692604885 ) ) ;
#9628=DIRECTION ( 'NONE',  ( 1.000000000000000000, -0.000000000000000000, 1.224646799147353207E-16 ) ) ;
#9632=FACE_OUTER_BOUND ( 'NONE', #4105, .T. ) ;
#9633=ORIENTED_EDGE ( 'NONE', *, *, #53706, .F. ) ;
#9637=CARTESIAN_POINT ( 'NONE',  ( 31.23437356469446868, 1523.382868172864164, 221.8968241038843416 ) ) ;
#9639=CARTESIAN_POINT ( 'NONE',  ( 29.74901212038063747, 1525.343727714918259, 196.2390656498153305 ) ) ;
#9651=EDGE_CURVE ( 'NONE', #4978, #73756, #52579, .T. ) ;
#9662=CARTESIAN_POINT ( 'NONE',  ( 16.50400130224743833, 1525.907212628473644, 181.9890130758377609 ) ) ;
#9667=DIRECTION ( 'NONE',  ( 0.000000000000000000, 1.000000000000000000, 0.000000000000000000 ) ) ;
#9685=CARTESIAN_POINT ( 'NONE',  ( 21.37469332459763649, 1525.408327360768681, 184.8352391485183546 ) ) ;
#9690=LINE ( 'NONE', #18082, #3237 ) ;
#9725=EDGE_LOOP ( 'NONE', ( #39679, #102762, #71434 ) ) ;
#9735=CARTESIAN_POINT ( 'NONE',  ( 21.33281718256687753, 1523.429859730330008, 180.4846393450492599 ) ) ;
#9736=CARTESIAN_POINT ( 'NONE',  ( 31.34137657934008558, 1512.187213306747481, 196.3411265156547358 ) ) ;
#9743=EDGE_CURVE ( 'NONE', #101207, #68013, #22146, .T. ) ;
#9745=CARTESIAN_POINT ( 'NONE',  ( 29.86281881105859171, 1525.137906803762689, 222.1296981937806549 ) ) ;
#9754=EDGE_CURVE ( 'NONE', #30213, #97183, #73196, .T. ) ;
#9759=EDGE_LOOP ( 'NONE', ( #36585, #80782, #71298, #34062, #26929 ) ) ;
#9762=CIRCLE ( 'NONE', #24037, 1.999999999999998668 ) ;
#9763=CARTESIAN_POINT ( 'NONE',  ( 28.96739426325766331, 1526.189892541618974, 197.4412433453230733 ) ) ;
#9764=CIRCLE ( 'NONE', #81209, 2.000000000000001776 ) ;
#9766=DIRECTION ( 'NONE',  ( -0.000000000000000000, -1.000000000000000000, -0.000000000000000000 ) ) ;
#9767=CARTESIAN_POINT ( 'NONE',  ( 22.03465957474552539, 1522.382868172863937, 182.8300405912328301 ) ) ;
#9770=EDGE_CURVE ( 'NONE', #11785, #49802, #2553, .T. ) ;
#9775=CARTESIAN_POINT ( 'NONE',  ( -22.04658257820682721, 1524.075000532257263, 184.4787014209232154 ) ) ;
#9795=VECTOR ( 'NONE', #48472, 1000.000000000000000 ) ;
#9797=EDGE_CURVE ( 'NONE', #21883, #49707, #108007, .T. ) ;
#9803=FACE_OUTER_BOUND ( 'NONE', #51013, .T. ) ;
#9805=FACE_OUTER_BOUND ( 'NONE', #79545, .T. ) ;
#9814=ADVANCED_FACE ( 'NONE', ( #11381 ), #36029, .T. ) ;
#9824=CARTESIAN_POINT ( 'NONE',  ( -31.97162612955063565, 1524.678541297860875, 201.5730793974714743 ) ) ;
#9832=ORIENTED_EDGE ( 'NONE', *, *, #45377, .F. ) ;
#9836=VECTOR ( 'NONE', #110241, 1000.000000000000000 ) ;
#9865=CARTESIAN_POINT ( 'NONE',  ( -30.25956561551428692, 1524.775785348137561, 221.7839847446165606 ) ) ;
#9882=EDGE_CURVE ( 'NONE', #51216, #90273, #20818, .T. ) ;
#9896=CARTESIAN_POINT ( 'NONE',  ( -32.39315898239558322, 1526.178928173327904, 201.3122567411319324 ) ) ;
#9900=CARTESIAN_POINT ( 'NONE',  ( -28.62254820377545528, 1526.345556099435726, 220.1905584258470867 ) ) ;
#9938=EDGE_CURVE ( 'NONE', #39550, #98801, #103308, .T. ) ;
#9961=( BOUNDED_SURFACE ( )  B_SPLINE_SURFACE ( 3, 2, ( 
 ( #10162, #79049, #77922 ),
 ( #35929, #19658, #19090 ),
 ( #26402, #28064, #43230 ),
 ( #70113, #69553, #45451 ),
 ( #60595, #2351, #71209 ),
 ( #2896, #104225, #105330 ),
 ( #95278, #78479, #43771 ),
 ( #27514, #37015, #94156 ),
 ( #61699, #17426, #53862 ),
 ( #35366, #36466, #680 ) ),
 .UNSPECIFIED., .F., .F., .T. ) 
 B_SPLINE_SURFACE_WITH_KNOTS ( ( 4, 2, 2, 2, 4 ),
 ( 3, 3 ),
 ( 0.000000000000000000, 0.3926990816987241395, 0.7853981633974482790, 1.178097245096172418, 1.570796326794896558 ),
 ( 0.000000000000000000, 1.000000000000000000 ),
 .UNSPECIFIED. ) 
 GEOMETRIC_REPRESENTATION_ITEM ( )  RATIONAL_B_SPLINE_SURFACE ( (
 ( 1.000000000000000000, 0.7763623250684335009, 1.000000000000000000),
 ( 1.000000000000000000, 0.7763684247036998221, 1.000000000000000000),
 ( 1.000000000000000000, 0.7746454561794836602, 1.000000000000000000),
 ( 1.000000000000000000, 0.7679730451975640415, 1.000000000000000000),
 ( 1.000000000000000000, 0.7630177051946724909, 1.000000000000000000),
 ( 1.000000000000000000, 0.7504512394528233266, 1.000000000000000000),
 ( 1.000000000000000000, 0.7428408967931069418, 1.000000000000000000),
 ( 1.000000000000000000, 0.7259222650906337337, 1.000000000000000000),
 ( 1.000000000000000000, 0.7166207884822691776, 1.000000000000000000),
 ( 1.000000000000000000, 0.7071067811865863195, 1.000000000000000000) ) ) 
 REPRESENTATION_ITEM ( '' )  SURFACE ( )  );
#9984=EDGE_LOOP ( 'NONE', ( #89008, #49247, #90211, #108020 ) ) ;
#10011=CARTESIAN_POINT ( 'NONE',  ( 31.34137657934019927, 1501.977400791986611, 221.9025654077410081 ) ) ;
#10023=CARTESIAN_POINT ( 'NONE',  ( 2.744860781518606352, 1525.790286462510267, 240.9440847703890256 ) ) ;
#10031=DIRECTION ( 'NONE',  ( 0.8090169943749551118, 0.000000000000000000, 0.5877852522924625900 ) ) ;
#10034=DIRECTION ( 'NONE',  ( -0.9942586961433758086, 0.000000000000000000, -0.1070030146457303932 ) ) ;
#10046=DIRECTION ( 'NONE',  ( 0.1070030146457445069, 0.000000000000000000, 0.9942586961433742543 ) ) ;
#10058=CARTESIAN_POINT ( 'NONE',  ( -32.38114538885245963, 1523.604703353109699, 216.1203639561433363 ) ) ;
#10101=DIRECTION ( 'NONE',  ( -0.9786619618251657382, 0.000000000000000000, 0.2054769195713179730 ) ) ;
#10116=ORIENTED_EDGE ( 'NONE', *, *, #82206, .T. ) ;
#10138=ORIENTED_EDGE ( 'NONE', *, *, #14374, .T. ) ;
#10162=CARTESIAN_POINT ( 'NONE',  ( -20.71343476517555260, 1522.382868172863937, 179.9059455038196802 ) ) ;
#10164=CARTESIAN_POINT ( 'NONE',  ( 204.2714532754872323, 1524.382868172863937, 194.5341519463041777 ) ) ;
#10181=VECTOR ( 'NONE', #85748, 1000.000000000000114 ) ;
#10187=CARTESIAN_POINT ( 'NONE',  ( 17.37724426307448411, 1525.394057003702756, 237.0493741307235780 ) ) ;
#10190=CARTESIAN_POINT ( 'NONE',  ( 19.53786426059019021, 1511.187213306747708, 181.5239794925693388 ) ) ;
#10203=CARTESIAN_POINT ( 'NONE',  ( -29.79244516855506220, 1525.556089352344543, 196.8434918795948931 ) ) ;
#10225=CARTESIAN_POINT ( 'NONE',  ( -19.53786426059057746, 1512.187213306747481, 181.5239794925695946 ) ) ;
#10231=CARTESIAN_POINT ( 'NONE',  ( -30.68434753601961162, 1526.000688113729211, 201.3936004808175255 ) ) ;
#10236=CIRCLE ( 'NONE', #99653, 1.000000000000000888 ) ;
#10241=CARTESIAN_POINT ( 'NONE',  ( 20.72500064272757214, 1525.697947650400920, 184.6549703297900464 ) ) ;
#10246=DIRECTION ( 'NONE',  ( 0.2054769195713296304, -0.000000000000000000, 0.9786619618251631847 ) ) ;
#10257=VERTEX_POINT ( 'NONE', #100852 ) ;
#10284=CARTESIAN_POINT ( 'NONE',  ( 21.98490254032972047, 1525.713797967456912, 182.9410524212044606 ) ) ;
#10295=CARTESIAN_POINT ( 'NONE',  ( 31.00891611928376790, 1524.547873515805122, 221.8102696095544673 ) ) ;
#10298=CARTESIAN_POINT ( 'NONE',  ( -16.49871405536275404, 1525.320849883625669, 237.0413307544871202 ) ) ;
#10300=EDGE_CURVE ( 'NONE', #92224, #33528, #41529, .T. ) ;
#10301=CARTESIAN_POINT ( 'NONE',  ( 31.12456774391179692, 1525.960063244516959, 217.0912716842395866 ) ) ;
#10306=CIRCLE ( 'NONE', #49725, 1.000000000000003775 ) ;
#10324=CARTESIAN_POINT ( 'NONE',  ( -31.81407709660785699, 1512.187213306747481, 196.2902540610632229 ) ) ;
#10335=CARTESIAN_POINT ( 'NONE',  ( -32.74318896774710907, 1524.667648926107177, 196.1902622063078070 ) ) ;
#10351=PLANE ( 'NONE',  #35331 ) ;
#10371=CARTESIAN_POINT ( 'NONE',  ( -32.05523756949325787, 1525.253972588462375, 201.2193331634007905 ) ) ;
#10383=ORIENTED_EDGE ( 'NONE', *, *, #26874, .F. ) ;
#10394=CIRCLE ( 'NONE', #103406, 29.51505616007316135 ) ;
#10397=CIRCLE ( 'NONE', #40764, 1.000000000000000888 ) ;
#10400=ADVANCED_FACE ( 'NONE', ( #97431 ), #109774, .T. ) ;
#10409=ORIENTED_EDGE ( 'NONE', *, *, #44865, .T. ) ;
#10419=CARTESIAN_POINT ( 'NONE',  ( -29.70307219812743682, 1525.408337840049626, 221.9454045032637737 ) ) ;
#10433=DIRECTION ( 'NONE',  ( -0.8090169943749481174, 0.000000000000000000, 0.5877852522924721379 ) ) ;
#10451=CARTESIAN_POINT ( 'NONE',  ( -33.17484411121699139, 1525.713797967457140, 200.8635405475165499 ) ) ;
#10466=CARTESIAN_POINT ( 'NONE',  ( 17.17241001986483795, 1512.187213306747481, 179.6185504016043240 ) ) ;
#10472=AXIS2_PLACEMENT_3D ( 'NONE', #61075, #77839, #109787 ) ;
#10478=DIRECTION ( 'NONE',  ( 0.000000000000000000, 0.000000000000000000, 1.000000000000000000 ) ) ;
#10479=( BOUNDED_SURFACE ( )  B_SPLINE_SURFACE ( 3, 2, ( 
 ( #21079, #12701, #73167 ),
 ( #30605, #46885, #106752 ),
 ( #30041, #64233, #22172 ),
 ( #56370, #102207, #93258 ),
 ( #68094, #16522, #94347 ),
 ( #33899, #100554, #68639 ),
 ( #17065, #50713, #49626 ),
 ( #9267, #51830, #23834 ),
 ( #43427, #75384, #83760 ),
 ( #84843, #77030, #84309 ) ),
 .UNSPECIFIED., .F., .F., .F. ) 
 B_SPLINE_SURFACE_WITH_KNOTS ( ( 4, 2, 2, 2, 4 ),
 ( 3, 3 ),
 ( 0.000000000000000000, 0.3926990816987241395, 0.7853981633974482790, 1.178097245096172418, 1.570796326794896558 ),
 ( 0.000000000000000000, 1.000000000000000000 ),
 .UNSPECIFIED. ) 
 GEOMETRIC_REPRESENTATION_ITEM ( )  RATIONAL_B_SPLINE_SURFACE ( (
 ( 1.000000000000000000, 0.7763623250684347221, 1.000000000000000000),
 ( 1.000000000000000000, 0.7763684247035179675, 1.000000000000000000),
 ( 1.000000000000000000, 0.7746454561797311289, 1.000000000000000000),
 ( 1.000000000000000000, 0.7679730451973156846, 1.000000000000000000),
 ( 1.000000000000000000, 0.7630177051950743916, 1.000000000000000000),
 ( 1.000000000000000000, 0.7504512394524318619, 1.000000000000000000),
 ( 1.000000000000000000, 0.7428408967929591711, 1.000000000000000000),
 ( 1.000000000000000000, 0.7259222650907819485, 1.000000000000000000),
 ( 1.000000000000000000, 0.7166207884821568230, 1.000000000000000000),
 ( 1.000000000000000000, 0.7071067811865867636, 1.000000000000000000) ) ) 
 REPRESENTATION_ITEM ( '' )  SURFACE ( )  );
#10483=VERTEX_POINT ( 'NONE', #11112 ) ;
#10490=CARTESIAN_POINT ( 'NONE',  ( -31.81407709660785699, 1522.382868172863937, 196.2902540610632229 ) ) ;
#10506=ORIENTED_EDGE ( 'NONE', *, *, #47269, .T. ) ;
#10531=ORIENTED_EDGE ( 'NONE', *, *, #68384, .F. ) ;
#10584=CARTESIAN_POINT ( 'NONE',  ( 2.472529913803048984, 1523.678648413191922, 242.8674788698241400 ) ) ;
#10607=ADVANCED_FACE ( 'NONE', ( #90543 ), #67211, .F. ) ;
#10611=DIRECTION ( 'NONE',  ( -0.8672669759446655080, 0.000000000000000000, -0.4978433412588692542 ) ) ;
#10623=CARTESIAN_POINT ( 'NONE',  ( -31.34137657934000387, 1512.187213306747481, 221.9025654077414345 ) ) ;
#10624=CARTESIAN_POINT ( 'NONE',  ( -32.79520046278567236, 1523.954924407800490, 217.1622218713099528 ) ) ;
#10625=ORIENTED_EDGE ( 'NONE', *, *, #83893, .F. ) ;
#10638=CARTESIAN_POINT ( 'NONE',  ( -2.470168521978398424, 1523.382868172864164, 242.8787258963054683 ) ) ;
#10645=TOROIDAL_SURFACE ( 'NONE', #66047, 2.000000000000000000, 1.000000000000000000 ) ;
#10651=CARTESIAN_POINT ( 'NONE',  ( -33.34040796508153903, 1523.342713519623658, 222.1177029624612658 ) ) ;
#10653=CARTESIAN_POINT ( 'NONE',  ( 31.88717309313577530, 1525.425665131969026, 201.2219480880026197 ) ) ;
#10682=ORIENTED_EDGE ( 'NONE', *, *, #39103, .F. ) ;
#10688=CYLINDRICAL_SURFACE ( 'NONE', #93101, 0.9999999999999976685 ) ;
#10703=EDGE_CURVE ( 'NONE', #15990, #37474, #100799, .T. ) ;
#10708=EDGE_CURVE ( 'NONE', #110178, #49611, #84749, .T. ) ;
#10736=CYLINDRICAL_SURFACE ( 'NONE', #10993, 1.999999999999994893 ) ;
#10741=CARTESIAN_POINT ( 'NONE',  ( 22.75273496409597485, 1512.187213306747481, 234.5707981297185825 ) ) ;
#10742=DIRECTION ( 'NONE',  ( 5.898059818321139072E-14, 0.000000000000000000, 1.000000000000000000 ) ) ;
#10782=DIRECTION ( 'NONE',  ( 0.5030436214085421964, 0.000000000000000000, 0.8642610224695890242 ) ) ;
#10796=DIRECTION ( 'NONE',  ( -0.9510565162951518658, 0.000000000000000000, 0.3090169943749528914 ) ) ;
#10808=CARTESIAN_POINT ( 'NONE',  ( 21.59932114087395405, 1525.137906803776104, 184.7402649365362493 ) ) ;
#10812=SHAPE_REPRESENTATION ( 'Threaded Lock Nut', ( #21632 ), #95028 ) ;
#10823=CARTESIAN_POINT ( 'NONE',  ( -33.36586802512182715, 1512.187213306747481, 201.9069332299493169 ) ) ;
#10828=ORIENTED_EDGE ( 'NONE', *, *, #6329, .T. ) ;
#10843=ORIENTED_EDGE ( 'NONE', *, *, #55441, .T. ) ;
#10847=ORIENTED_EDGE ( 'NONE', *, *, #57868, .F. ) ;
#10852=DIRECTION ( 'NONE',  ( -0.000000000000000000, 1.000000000000000000, -0.000000000000000000 ) ) ;
#10854=CARTESIAN_POINT ( 'NONE',  ( 6.144376325710431352, 1512.187213306747481, 247.6867189913432981 ) ) ;
#10867=CARTESIAN_POINT ( 'NONE',  ( 31.25788889089079703, 1523.954924407802764, 221.8935803876606485 ) ) ;
#10871=CARTESIAN_POINT ( 'NONE',  ( -17.34064570863325372, 1525.506926151471362, 236.9219808115470869 ) ) ;
#10875=CARTESIAN_POINT ( 'NONE',  ( 24.25895011704442084, 1512.187213306747481, 247.1119212070236131 ) ) ;
#10911=AXIS2_PLACEMENT_3D ( 'NONE', #68341, #59935, #110308 ) ;
#10920=CARTESIAN_POINT ( 'NONE',  ( -22.08622291482313926, 1523.382868172864164, 233.8253038720786776 ) ) ;
#10931=VERTEX_POINT ( 'NONE', #24974 ) ;
#10934=ADVANCED_FACE ( 'NONE', ( #95517 ), #32038, .T. ) ;
#10939=CARTESIAN_POINT ( 'NONE',  ( -31.14814740293979511, 1525.697946996596102, 201.5095778062523948 ) ) ;
#10950=ORIENTED_EDGE ( 'NONE', *, *, #863, .F. ) ;
#10954=ORIENTED_EDGE ( 'NONE', *, *, #28974, .F. ) ;
#10960=VERTEX_POINT ( 'NONE', #8185 ) ;
#10974=CARTESIAN_POINT ( 'NONE',  ( -17.84338787571961049, 1512.187213306747481, 180.3600277896300383 ) ) ;
#10983=ORIENTED_EDGE ( 'NONE', *, *, #73548, .F. ) ;
#10993=AXIS2_PLACEMENT_3D ( 'NONE', #54952, #79056, #89078 ) ;
#10997=DIRECTION ( 'NONE',  ( 0.4090087482554189968, 0.000000000000000000, -0.9125304618754023211 ) ) ;
#11005=ORIENTED_EDGE ( 'NONE', *, *, #51793, .F. ) ;
#11006=AXIS2_PLACEMENT_3D ( 'NONE', #65858, #74264, #82646 ) ;
#11012=CARTESIAN_POINT ( 'NONE',  ( -21.19079385647338754, 1525.394057003702756, 234.2786681684617349 ) ) ;
#11029=LINE ( 'NONE', #79339, #100043 ) ;
#11033=CARTESIAN_POINT ( 'NONE',  ( 28.49879435373766157, 1526.382868172571079, 219.8425395114742855 ) ) ;
#11045=FACE_OUTER_BOUND ( 'NONE', #102902, .T. ) ;
#11046=ORIENTED_EDGE ( 'NONE', *, *, #15472, .T. ) ;
#11047=ORIENTED_EDGE ( 'NONE', *, *, #8057, .F. ) ;
#11055=VECTOR ( 'NONE', #50568, 1000.000000000000000 ) ;
#11063=CARTESIAN_POINT ( 'NONE',  ( 2.738357795398948635, 1525.795403383247276, 240.9366230306859222 ) ) ;
#11073=EDGE_CURVE ( 'NONE', #23627, #77339, #69114, .T. ) ;
#11077=EDGE_CURVE ( 'NONE', #24499, #53518, #108932, .T. ) ;
#11087=ORIENTED_EDGE ( 'NONE', *, *, #2998, .F. ) ;
#11096=B_SPLINE_CURVE_WITH_KNOTS ( 'NONE', 3,
 ( #86803, #69483, #87366, #54877, #36398, #95209, #61626, #18470, #80057, #77858 ),
 .UNSPECIFIED., .F., .F.,
 ( 4, 2, 2, 2, 4 ),
 ( 0.000000000000000000, 0.0007403986298595332041, 0.001480797259719066408, 0.002221195889578599612, 0.002961594519438132816 ),
 .UNSPECIFIED. ) ;
#11101=CARTESIAN_POINT ( 'NONE',  ( -28.72841836130733739, 1526.333389947941669, 198.1146668274939202 ) ) ;
#11102=EDGE_CURVE ( 'NONE', #43690, #1895, #40459, .T. ) ;
#11112=CARTESIAN_POINT ( 'NONE',  ( 20.49599333844873783, 1525.960063244516959, 233.8638087104922931 ) ) ;
#11117=ADVANCED_FACE ( 'NONE', ( #96284 ), #94096, .T. ) ;
#11120=FACE_OUTER_BOUND ( 'NONE', #42461, .T. ) ;
#11146=CARTESIAN_POINT ( 'NONE',  ( 2.708826876439114795, 1524.477587234266139, 241.9484498748172143 ) ) ;
#11147=ORIENTED_EDGE ( 'NONE', *, *, #101594, .T. ) ;
#11149=CARTESIAN_POINT ( 'NONE',  ( 21.61625474793598300, 1526.178928173327677, 234.4801574852378394 ) ) ;
#11154=( BOUNDED_SURFACE ( )  B_SPLINE_SURFACE ( 3, 2, ( 
 ( #58782, #8909, #92920 ),
 ( #16192, #43086, #84522 ),
 ( #41978, #85062, #110270 ),
 ( #8354, #76676, #34119 ) ),
 .UNSPECIFIED., .F., .F., .F. ) 
 B_SPLINE_SURFACE_WITH_KNOTS ( ( 4, 4 ),
 ( 3, 3 ),
 ( 0.000000000000000000, 0.0002960034161023851105 ),
 ( 0.000000000000000000, 1.000000000000000000 ),
 .UNSPECIFIED. ) 
 GEOMETRIC_REPRESENTATION_ITEM ( )  RATIONAL_B_SPLINE_SURFACE ( (
 ( 1.000000000000000000, 0.8070209408750074198, 1.000000000000000000),
 ( 1.000000000000000000, 0.8071723757218278728, 1.000000000000000000),
 ( 1.000000000000000000, 0.8072480346917794147, 1.000000000000000000),
 ( 1.000000000000000000, 0.8072480644198116728, 1.000000000000000000) ) ) 
 REPRESENTATION_ITEM ( '' )  SURFACE ( )  );
#11165=ORIENTED_EDGE ( 'NONE', *, *, #26080, .F. ) ;
#11172=VECTOR ( 'NONE', #86312, 1000.000000000000227 ) ;
#11182=ORIENTED_EDGE ( 'NONE', *, *, #106394, .F. ) ;
#11200=CARTESIAN_POINT ( 'NONE',  ( -3.448830483803564828, 1518.913060387330006, 243.0842028158767789 ) ) ;
#11204=ORIENTED_EDGE ( 'NONE', *, *, #104329, .F. ) ;
#11210=CARTESIAN_POINT ( 'NONE',  ( -31.03088476499755899, 1523.982201850120191, 221.8691499995721870 ) ) ;
#11212=CARTESIAN_POINT ( 'NONE',  ( 32.00451504911072931, 1524.843416604514232, 202.1266007667272788 ) ) ;
#11222=CARTESIAN_POINT ( 'NONE',  ( 22.08523692261567817, 1523.530935881284904, 233.8225055907668377 ) ) ;
#11244=ORIENTED_EDGE ( 'NONE', *, *, #359, .T. ) ;
#11271=CARTESIAN_POINT ( 'NONE',  ( 32.38845791999500534, 1523.456872492435195, 216.1254071228445355 ) ) ;
#11272=CARTESIAN_POINT ( 'NONE',  ( 0.4151546846821903003, 1522.382868172863937, 173.3106345060153046 ) ) ;
#11285=DIRECTION ( 'NONE',  ( 0.000000000000000000, 0.000000000000000000, 1.000000000000000000 ) ) ;
#11289=CARTESIAN_POINT ( 'NONE',  ( 0.000000000000000000, 1523.382868172864164, 209.1218459616979999 ) ) ;
#11291=DIRECTION ( 'NONE',  ( 0.000000000000000000, 1.000000000000000000, 0.000000000000000000 ) ) ;
#11300=CARTESIAN_POINT ( 'NONE',  ( -1.393816646507355150, 1511.187213306747708, 175.1051575864439656 ) ) ;
#11308=DIRECTION ( 'NONE',  ( -0.8090169943749402348, 0.000000000000000000, 0.5877852522924831291 ) ) ;
#11310=CARTESIAN_POINT ( 'NONE',  ( 32.23393008293545847, 1523.462669333490567, 216.8400319009756174 ) ) ;
#11321=CARTESIAN_POINT ( 'NONE',  ( 32.09235212274781190, 1525.402221411319260, 196.2603058525789663 ) ) ;
#11325=CARTESIAN_POINT ( 'NONE',  ( -29.41653834772467135, 1525.790287071772127, 196.6777166491189064 ) ) ;
#11327=CARTESIAN_POINT ( 'NONE',  ( 19.34601893677012185, 1526.333389947941441, 233.0427900344711816 ) ) ;
#11350=EDGE_CURVE ( 'NONE', #32684, #100188, #70840, .T. ) ;
#11381=FACE_OUTER_BOUND ( 'NONE', #68666, .T. ) ;
#11384=ORIENTED_EDGE ( 'NONE', *, *, #44367, .F. ) ;
#11422=DIRECTION ( 'NONE',  ( 0.3090169943749582204, 0.000000000000000000, 0.9510565162951499785 ) ) ;
#11447=CARTESIAN_POINT ( 'NONE',  ( -21.80586122364568169, 1523.954914175599924, 183.3405075822116430 ) ) ;
#11459=VECTOR ( 'NONE', #87276, 1000.000000000000000 ) ;
#11467=CARTESIAN_POINT ( 'NONE',  ( 30.31052258194586102, 1523.604703353109699, 195.7506062427368079 ) ) ;
#11483=AXIS2_PLACEMENT_3D ( 'NONE', #15466, #30637, #82132 ) ;
#11491=LINE ( 'NONE', #36684, #67259 ) ;
#11495=DIRECTION ( 'NONE',  ( -0.8090169943749467851, 1.070063492533079265E-14, -0.5877852522924740253 ) ) ;
#11497=ADVANCED_FACE ( 'NONE', ( #7184 ), #42430, .F. ) ;
#11505=CARTESIAN_POINT ( 'NONE',  ( -20.20959865099451847, 1501.977400791986611, 236.2316688286741453 ) ) ;
#11506=CARTESIAN_POINT ( 'NONE',  ( 21.08094518543042284, 1525.506926151471362, 234.2044941741795867 ) ) ;
#11527=CIRCLE ( 'NONE', #74116, 1.000000000000000888 ) ;
#11535=CARTESIAN_POINT ( 'NONE',  ( -30.12464261468167592, 1524.523992613102337, 222.3823409144095535 ) ) ;
#11547=CARTESIAN_POINT ( 'NONE',  ( -30.79107737087808871, 1526.107876515966609, 217.1184129874169741 ) ) ;
#11551=CARTESIAN_POINT ( 'NONE',  ( 22.08523867432351295, 1523.530870145309564, 184.4211813602697134 ) ) ;
#11553=CARTESIAN_POINT ( 'NONE',  ( 16.66936639845630097, 1512.187213306747481, 180.4828114240739296 ) ) ;
#11575=CARTESIAN_POINT ( 'NONE',  ( -30.31052258194604576, 1523.604703353109699, 195.7506062427372058 ) ) ;
#11579=CARTESIAN_POINT ( 'NONE',  ( -3.177670542995198133, 1525.042412244750722, 241.6057155832064325 ) ) ;
#11591=EDGE_LOOP ( 'NONE', ( #38777, #47710, #72689, #105048 ) ) ;
#11598=CARTESIAN_POINT ( 'NONE',  ( 21.41971086555102133, 1512.187213306747481, 233.0798096144380906 ) ) ;
#11623=CARTESIAN_POINT ( 'NONE',  ( -32.02808312589930040, 1522.382868172863937, 198.2787714533499752 ) ) ;
#11636=ORIENTED_EDGE ( 'NONE', *, *, #75415, .F. ) ;
#11647=FACE_OUTER_BOUND ( 'NONE', #7794, .T. ) ;
#11649=ORIENTED_EDGE ( 'NONE', *, *, #81444, .T. ) ;
#11652=EDGE_CURVE ( 'NONE', #94335, #100110, #1974, .T. ) ;
#11679=CARTESIAN_POINT ( 'NONE',  ( 2.664386649655714479, 1523.844782250841263, 242.1314419845511452 ) ) ;
#11681=CYLINDRICAL_SURFACE ( 'NONE', #70614, 4.000000000000000888 ) ;
#11682=CARTESIAN_POINT ( 'NONE',  ( 21.19880661589004589, 1526.382868172863937, 233.5487980989310870 ) ) ;
#11684=EDGE_CURVE ( 'NONE', #59426, #4978, #2148, .T. ) ;
#11687=EDGE_CURVE ( 'NONE', #12956, #71433, #3015, .T. ) ;
#11689=ADVANCED_FACE ( 'NONE', ( #25058 ), #15551, .T. ) ;
#11712=EDGE_CURVE ( 'NONE', #31615, #61519, #108480, .T. ) ;
#11720=CARTESIAN_POINT ( 'NONE',  ( -31.14814639457161860, 1525.697947650476863, 216.7341144156438020 ) ) ;
#11721=VERTEX_POINT ( 'NONE', #91731 ) ;
#11725=AXIS2_PLACEMENT_3D ( 'NONE', #65390, #40713, #16039 ) ;
#11736=CARTESIAN_POINT ( 'NONE',  ( 3.347801439296141268, 1518.913060387330006, 242.0893193391992497 ) ) ;
#11740=ORIENTED_EDGE ( 'NONE', *, *, #16426, .T. ) ;
#11744=CARTESIAN_POINT ( 'NONE',  ( -31.69312280309771879, 1525.713797967456685, 221.9404206525577479 ) ) ;
#11754=CARTESIAN_POINT ( 'NONE',  ( 22.08622291482350519, 1523.382868172864164, 233.8253038720783366 ) ) ;
#11757=CARTESIAN_POINT ( 'NONE',  ( 32.85805783624304155, 1523.678648413191695, 201.0453875934054508 ) ) ;
#11758=EDGE_LOOP ( 'NONE', ( #4939, #88177, #19008, #18202 ) ) ;
#11780=DIRECTION ( 'NONE',  ( -0.8090169943749465631, 0.000000000000000000, 0.5877852522924742473 ) ) ;
#11785=VERTEX_POINT ( 'NONE', #10920 ) ;
#11799=CARTESIAN_POINT ( 'NONE',  ( 0.7800921441517267851, 1526.382868172863937, 176.7869413415625388 ) ) ;
#11818=CARTESIAN_POINT ( 'NONE',  ( 21.84020450222037724, 1523.481610426287489, 183.2638850454218016 ) ) ;
#11861=DIRECTION ( 'NONE',  ( 0.8090169943749466741, 0.000000000000000000, -0.5877852522924743583 ) ) ;
#11864=DIRECTION ( 'NONE',  ( 0.000000000000000000, 1.000000000000000000, 0.000000000000000000 ) ) ;
#11866=CARTESIAN_POINT ( 'NONE',  ( -30.00906612069109869, 1525.856065479233393, 197.1249957521959288 ) ) ;
#11876=CARTESIAN_POINT ( 'NONE',  ( 2.131986625828341086, 1526.000688113688057, 177.5511380990155601 ) ) ;
#11882=CARTESIAN_POINT ( 'NONE',  ( -156.6846457583352503, 1526.382868172863937, 77.25240589482224607 ) ) ;
#11889=CARTESIAN_POINT ( 'NONE',  ( 31.23437356469446158, 1523.382868172864164, 222.8968241038843416 ) ) ;
#11903=ORIENTED_EDGE ( 'NONE', *, *, #109794, .T. ) ;
#11921=ORIENTED_EDGE ( 'NONE', *, *, #110238, .T. ) ;
#11929=AXIS2_PLACEMENT_3D ( 'NONE', #61600, #52641, #86778 ) ;
#11940=ORIENTED_EDGE ( 'NONE', *, *, #28441, .F. ) ;
#11945=DIRECTION ( 'NONE',  ( 0.000000000000000000, 1.000000000000000000, 0.000000000000000000 ) ) ;
#11954=CARTESIAN_POINT ( 'NONE',  ( -32.52419458002813002, 1524.600389084707103, 217.0761871924782156 ) ) ;
#11977=ORIENTED_EDGE ( 'NONE', *, *, #50862, .T. ) ;
#11981=EDGE_CURVE ( 'NONE', #39456, #97183, #14200, .T. ) ;
#11984=CARTESIAN_POINT ( 'NONE',  ( -29.40443212115374649, 1512.187213306747481, 222.0897836382247306 ) ) ;
#11988=DIRECTION ( 'NONE',  ( -0.2113515706023144647, -1.466546124833779360E-15, 0.9774101051267757301 ) ) ;
#11992=ORIENTED_EDGE ( 'NONE', *, *, #9132, .T. ) ;
#11999=EDGE_CURVE ( 'NONE', #29284, #68807, #105960, .T. ) ;
#12002=AXIS2_PLACEMENT_3D ( 'NONE', #42026, #83456, #100274 ) ;
#12009=CARTESIAN_POINT ( 'NONE',  ( 31.32995031131189378, 1523.678648413191695, 196.3423562208913324 ) ) ;
#12010=ORIENTED_EDGE ( 'NONE', *, *, #31489, .F. ) ;
#12021=CARTESIAN_POINT ( 'NONE',  ( 2.470168521978396203, 1512.187213306747481, 242.8787258963054683 ) ) ;
#12030=DIRECTION ( 'NONE',  ( 0.000000000000000000, 1.000000000000000000, 0.000000000000000000 ) ) ;
#12035=CARTESIAN_POINT ( 'NONE',  ( -31.32995031131211761, 1523.678648413191695, 196.3423562208917588 ) ) ;
#12045=CARTESIAN_POINT ( 'NONE',  ( 0.4151546846821903003, 1522.382868172863937, 175.3106345060153046 ) ) ;
#12046=CARTESIAN_POINT ( 'NONE',  ( 21.39312961732869312, 1524.775785348137333, 233.9875869515353202 ) ) ;
#12054=ORIENTED_EDGE ( 'NONE', *, *, #51184, .F. ) ;
#12059=DIRECTION ( 'NONE',  ( 0.000000000000000000, 0.000000000000000000, 1.000000000000000000 ) ) ;
#12063=ORIENTED_EDGE ( 'NONE', *, *, #69514, .F. ) ;
#12073=CARTESIAN_POINT ( 'NONE',  ( -31.00914578553006962, 1524.547395018738371, 221.8103655202198468 ) ) ;
#12080=ORIENTED_EDGE ( 'NONE', *, *, #77220, .F. ) ;
#12089=CARTESIAN_POINT ( 'NONE',  ( 21.84020450222038079, 1523.382868172864164, 183.2638850454218016 ) ) ;
#12096=ORIENTED_EDGE ( 'NONE', *, *, #19891, .T. ) ;
#12121=CARTESIAN_POINT ( 'NONE',  ( -3.350338079455601026, 1523.604703353109699, 242.0808062845893289 ) ) ;
#12136=EDGE_LOOP ( 'NONE', ( #25568, #49174, #91473 ) ) ;
#12142=CARTESIAN_POINT ( 'NONE',  ( 76.99707197885322785, 1526.382868172863937, 398.8876973329328735 ) ) ;
#12153=CARTESIAN_POINT ( 'NONE',  ( -33.36586802512183425, 1523.382868172864164, 201.9069332299493169 ) ) ;
#12155=VERTEX_POINT ( 'NONE', #68788 ) ;
#12169=EDGE_LOOP ( 'NONE', ( #99562, #27080, #8060, #51909 ) ) ;
#12171=ORIENTED_EDGE ( 'NONE', *, *, #51072, .F. ) ;
#12175=AXIS2_PLACEMENT_3D ( 'NONE', #81669, #99575, #97928 ) ;
#12203=VERTEX_POINT ( 'NONE', #59279 ) ;
#12208=CARTESIAN_POINT ( 'NONE',  ( 18.86688640473582268, 1511.187213306747708, 180.7825021045438518 ) ) ;
#12220=CARTESIAN_POINT ( 'NONE',  ( -32.85805783624297760, 1523.678648413191695, 217.1983043299907763 ) ) ;
#12223=CARTESIAN_POINT ( 'NONE',  ( 21.71247731329056307, 1523.982201850120191, 234.6948375436859635 ) ) ;
#12224=AXIS2_PLACEMENT_3D ( 'NONE', #19257, #11988, #55120 ) ;
#12226=ADVANCED_FACE ( 'NONE', ( #90784 ), #16413, .T. ) ;
#12227=VECTOR ( 'NONE', #100363, 1000.000000000000000 ) ;
#12235=EDGE_CURVE ( 'NONE', #43726, #39623, #39840, .T. ) ;
#12237=CARTESIAN_POINT ( 'NONE',  ( -32.86802468386297704, 1512.187213306747481, 201.0396662540046577 ) ) ;
#12252=CARTESIAN_POINT ( 'NONE',  ( -2.038646110889675178, 1525.960063244516959, 177.0579350083066004 ) ) ;
#12265=CARTESIAN_POINT ( 'NONE',  ( 32.02808312589916540, 1511.187213306747708, 198.2787714533495489 ) ) ;
#12274=EDGE_LOOP ( 'NONE', ( #36625, #101627, #12888, #6946 ) ) ;
#12282=CARTESIAN_POINT ( 'NONE',  ( 32.18357971099926118, 1524.059663615499630, 201.4963562058872526 ) ) ;
#12290=CARTESIAN_POINT ( 'NONE',  ( 30.95751052620453692, 1525.821544997590536, 201.4531494772885196 ) ) ;
#12291=FACE_OUTER_BOUND ( 'NONE', #36705, .T. ) ;
#12310=ORIENTED_EDGE ( 'NONE', *, *, #67340, .T. ) ;
#12311=CARTESIAN_POINT ( 'NONE',  ( 173.8335085727383955, 1526.382868172863937, 100.8557906292069930 ) ) ;
#12314=EDGE_LOOP ( 'NONE', ( #106570, #29558, #27303, #64706, #10983 ) ) ;
#12323=CARTESIAN_POINT ( 'NONE',  ( 16.64885258017236680, 1526.344110814218311, 234.9109520333671810 ) ) ;
#12335=CARTESIAN_POINT ( 'NONE',  ( 16.81497685297909683, 1526.382868172864164, 234.5399785031295892 ) ) ;
#12341=LINE ( 'NONE', #46532, #101366 ) ;
#12351=ORIENTED_EDGE ( 'NONE', *, *, #79504, .F. ) ;
#12353=CIRCLE ( 'NONE', #74969, 1.000000000000007994 ) ;
#12361=ORIENTED_EDGE ( 'NONE', *, *, #74879, .F. ) ;
#12376=CARTESIAN_POINT ( 'NONE',  ( -21.30823923614777371, 1524.382868172804365, 233.7929508216643342 ) ) ;
#12384=AXIS2_PLACEMENT_3D ( 'NONE', #94202, #42719, #34305 ) ;
#12391=CARTESIAN_POINT ( 'NONE',  ( 19.39983987835400114, 1522.382868172864164, 178.9515629539735642 ) ) ;
#12392=CARTESIAN_POINT ( 'NONE',  ( 22.03465957474570658, 1522.382868172863937, 235.4136513321629991 ) ) ;
#12399=CARTESIAN_POINT ( 'NONE',  ( 32.74318896774778409, 1524.667648926106949, 196.1902622063073807 ) ) ;
#12406=ADVANCED_FACE ( 'NONE', ( #80482 ), #13243, .T. ) ;
#12413=CARTESIAN_POINT ( 'NONE',  ( 1.775988990184984795, 1526.208281990536761, 177.6737791622277882 ) ) ;
#12419=CARTESIAN_POINT ( 'NONE',  ( 2.372478608332516892, 1512.187213306747481, 174.8996806668726549 ) ) ;
#12421=VECTOR ( 'NONE', #77683, 1000.000000000000114 ) ;
#12427=CARTESIAN_POINT ( 'NONE',  ( 19.37374569213924502, 1526.382868172863937, 183.8768763279539655 ) ) ;
#12430=DIRECTION ( 'NONE',  ( 0.8090169943749551118, -0.000000000000000000, 0.5877852522924625900 ) ) ;
#12447=EDGE_CURVE ( 'NONE', #89941, #24269, #102268, .T. ) ;
#12464=AXIS2_PLACEMENT_3D ( 'NONE', #82281, #23997, #82823 ) ;
#12474=AXIS2_PLACEMENT_3D ( 'NONE', #8099, #49033, #92657 ) ;
#12482=ORIENTED_EDGE ( 'NONE', *, *, #93254, .F. ) ;
#12484=ORIENTED_EDGE ( 'NONE', *, *, #28927, .F. ) ;
#12514=CARTESIAN_POINT ( 'NONE',  ( -17.05907944273172561, 1524.678541297861102, 237.1959721738423070 ) ) ;
#12517=CARTESIAN_POINT ( 'NONE',  ( 29.33952678943222736, 1526.382868172864164, 217.1408869592839324 ) ) ;
#12519=DIRECTION ( 'NONE',  ( -0.000000000000000000, -1.000000000000000000, -0.000000000000000000 ) ) ;
#12523=DIRECTION ( 'NONE',  ( 0.8090169943749551118, -0.000000000000000000, 0.5877852522924624790 ) ) ;
#12530=EDGE_CURVE ( 'NONE', #17686, #41312, #4194, .T. ) ;
#12551=AXIS2_PLACEMENT_3D ( 'NONE', #95636, #53667, #53102 ) ;
#12556=B_SPLINE_CURVE_WITH_KNOTS ( 'NONE', 3,
 ( #75044, #92362, #76678, #101295, #101856, #83417, #34122, #102420, #85064, #66104, #67195, #40868 ),
 .UNSPECIFIED., .F., .F.,
 ( 4, 2, 2, 2, 2, 4 ),
 ( 0.000000000000000000, 0.0007194225121803802993, 0.001079133768270255488, 0.001438845024360130894, 0.002158267536539314451, 0.002877690048718498008 ),
 .UNSPECIFIED. ) ;
#12600=CARTESIAN_POINT ( 'NONE',  ( 21.14962954806519591, 1525.231909165050638, 233.8093717500290154 ) ) ;
#12608=EDGE_CURVE ( 'NONE', #103878, #45131, #60122, .T. ) ;
#12625=PLANE ( 'NONE',  #7005 ) ;
#12644=CARTESIAN_POINT ( 'NONE',  ( -31.12456774391156600, 1525.960063244517187, 217.0912716842400698 ) ) ;
#12647=CIRCLE ( 'NONE', #34064, 0.9999999999999100719 ) ;
#12661=AXIS2_PLACEMENT_3D ( 'NONE', #10741, #36480, #87447 ) ;
#12664=CARTESIAN_POINT ( 'NONE',  ( 17.30126322281369866, 1523.382868172864164, 180.8506073313484990 ) ) ;
#12669=FACE_OUTER_BOUND ( 'NONE', #14083, .T. ) ;
#12670=ORIENTED_EDGE ( 'NONE', *, *, #21286, .T. ) ;
#12676=CARTESIAN_POINT ( 'NONE',  ( 2.385019621457262762, 1526.073429442291626, 240.5311921326816673 ) ) ;
#12677=CARTESIAN_POINT ( 'NONE',  ( -2.410642264446942296, 1525.163527997520532, 242.1266861310988645 ) ) ;
#12687=CARTESIAN_POINT ( 'NONE',  ( 33.93019615848946557, 1522.382868172863937, 197.6607374645996060 ) ) ;
#12689=ORIENTED_EDGE ( 'NONE', *, *, #101059, .F. ) ;
#12701=CARTESIAN_POINT ( 'NONE',  ( -2.038847259689227531, 1522.382868172863937, 244.9330574173806667 ) ) ;
#12707=CARTESIAN_POINT ( 'NONE',  ( 33.28034951413762599, 1522.644714754858114, 200.8029765415147097 ) ) ;
#12717=DIRECTION ( 'NONE',  ( 0.4090087482554383702, -0.000000000000000000, 0.9125304618753937724 ) ) ;
#12721=CARTESIAN_POINT ( 'NONE',  ( -0.4151546846821903003, 1512.187213306747481, 243.9330574173806951 ) ) ;
#12730=ORIENTED_EDGE ( 'NONE', *, *, #98607, .F. ) ;
#12732=AXIS2_PLACEMENT_3D ( 'NONE', #98584, #21850, #82345 ) ;
#12755=EDGE_CURVE ( 'NONE', #50508, #89888, #37658, .T. ) ;
#12769=ORIENTED_EDGE ( 'NONE', *, *, #12755, .F. ) ;
#12771=B_SPLINE_CURVE_WITH_KNOTS ( 'NONE', 3,
 ( #12220, #79446, #46414, #1648 ),
 .UNSPECIFIED., .F., .F.,
 ( 4, 4 ),
 ( 0.000000000000000000, 0.0002960034161023851105 ),
 .UNSPECIFIED. ) ;
#12778=FACE_OUTER_BOUND ( 'NONE', #102231, .T. ) ;
#12787=CIRCLE ( 'NONE', #48542, 2.000000000000001776 ) ;
#12789=CARTESIAN_POINT ( 'NONE',  ( 30.25425994617003767, 1526.382868172863937, 199.2916410102368729 ) ) ;
#12796=ORIENTED_EDGE ( 'NONE', *, *, #93847, .F. ) ;
#12807=DIRECTION ( 'NONE',  ( 0.000000000000000000, 1.000000000000000000, -0.000000000000000000 ) ) ;
#12821=LINE ( 'NONE', #30166, #8836 ) ;
#12827=CARTESIAN_POINT ( 'NONE',  ( 20.71343476517534299, 1522.382868172863937, 238.3377464195763764 ) ) ;
#12834=AXIS2_PLACEMENT_3D ( 'NONE', #54347, #88478, #97956 ) ;
#12848=DIRECTION ( 'NONE',  ( 0.000000000000000000, 0.000000000000000000, 1.000000000000000000 ) ) ;
#12867=CARTESIAN_POINT ( 'NONE',  ( 32.02808312589922224, 1512.187213306747481, 219.9649204700462235 ) ) ;
#12869=ORIENTED_EDGE ( 'NONE', *, *, #77699, .F. ) ;
#12878=ORIENTED_EDGE ( 'NONE', *, *, #68151, .T. ) ;
#12888=ORIENTED_EDGE ( 'NONE', *, *, #85913, .T. ) ;
#12889=CARTESIAN_POINT ( 'NONE',  ( 2.582675909239575240, 1526.178928173327677, 175.9008252398585626 ) ) ;
#12917=CARTESIAN_POINT ( 'NONE',  ( 29.36867415615326493, 1526.382868172863937, 217.2593511714356396 ) ) ;
#12921=CARTESIAN_POINT ( 'NONE',  ( -21.92916355573673570, 1523.390106123591067, 235.1782814742750816 ) ) ;
#12951=CARTESIAN_POINT ( 'NONE',  ( -18.02257621027557377, 1526.382868172863937, 235.3484976865589147 ) ) ;
#12954=CARTESIAN_POINT ( 'NONE',  ( -2.622430729442961184, 1523.621879633028811, 176.0901726876731459 ) ) ;
#12956=VERTEX_POINT ( 'NONE', #104716 ) ;
#12975=EDGE_LOOP ( 'NONE', ( #31553, #92556, #58473, #34003, #52841 ) ) ;
#13001=CARTESIAN_POINT ( 'NONE',  ( 32.10255801038882595, 1525.211477436245787, 217.0238529843554716 ) ) ;
#13015=EDGE_LOOP ( 'NONE', ( #81408, #16714, #27284 ) ) ;
#13035=ORIENTED_EDGE ( 'NONE', *, *, #31050, .F. ) ;
#13036=CARTESIAN_POINT ( 'NONE',  ( -17.72020223055791632, 1524.201670966335769, 237.7556192861110560 ) ) ;
#13040=CARTESIAN_POINT ( 'NONE',  ( -31.34137657934027388, 1523.382868172864164, 196.3411265156551906 ) ) ;
#13051=ADVANCED_FACE ( 'NONE', ( #36955 ), #23628, .T. ) ;
#13062=ADVANCED_FACE ( 'NONE', ( #6109 ), #90662, .T. ) ;
#13064=DIRECTION ( 'NONE',  ( 0.000000000000000000, 0.000000000000000000, -1.000000000000000000 ) ) ;
#13076=CARTESIAN_POINT ( 'NONE',  ( -20.28160989820316473, 1526.000688113805609, 184.8337570730359118 ) ) ;
#13102=ORIENTED_EDGE ( 'NONE', *, *, #102697, .T. ) ;
#13108=CARTESIAN_POINT ( 'NONE',  ( -33.42844755917204225, 1501.977400791986611, 196.1165140606796058 ) ) ;
#13109=DIRECTION ( 'NONE',  ( -2.664535259100375697E-15, 0.000000000000000000, 1.000000000000000000 ) ) ;
#13119=VERTEX_POINT ( 'NONE', #108014 ) ;
#13121=CARTESIAN_POINT ( 'NONE',  ( 21.66438254905593652, 1525.042337199239455, 233.5340853539618138 ) ) ;
#13130=ORIENTED_EDGE ( 'NONE', *, *, #32223, .F. ) ;
#13136=ORIENTED_EDGE ( 'NONE', *, *, #95366, .T. ) ;
#13140=CARTESIAN_POINT ( 'NONE',  ( -30.98807061075481428, 1524.600389084707103, 196.4398012796251010 ) ) ;
#13151=CARTESIAN_POINT ( 'NONE',  ( 28.44964981546457850, 1526.382868172864164, 198.3640452512597108 ) ) ;
#13152=CARTESIAN_POINT ( 'NONE',  ( -30.60461244942465342, 1523.621879633029039, 221.8232741897822677 ) ) ;
#13160=ADVANCED_FACE ( 'NONE', ( #95091 ), #85562, .T. ) ;
#13167=CIRCLE ( 'NONE', #54476, 1.000000000000000888 ) ;
#13179=DIRECTION ( 'NONE',  ( -9.714451465470110893E-14, 0.000000000000000000, 1.000000000000000000 ) ) ;
#13190=CARTESIAN_POINT ( 'NONE',  ( 20.53760542139758627, 1525.821544997590763, 184.7213720461153912 ) ) ;
#13192=CYLINDRICAL_SURFACE ( 'NONE', #33121, 4.000000000000002665 ) ;
#13206=ADVANCED_BREP_SHAPE_REPRESENTATION ( '', ( #8479, #21632 ), #95028 ) ;
#13207=ADVANCED_FACE ( 'NONE', ( #19472 ), #82226, .F. ) ;
#13232=CARTESIAN_POINT ( 'NONE',  ( 32.85805783624308418, 1523.678648413191695, 217.1983043299902931 ) ) ;
#13235=CARTESIAN_POINT ( 'NONE',  ( 31.50799703744284130, 1526.382868172863937, 201.8203724569130202 ) ) ;
#13243=CYLINDRICAL_SURFACE ( 'NONE', #39698, 2.000000000000003553 ) ;
#13261=AXIS2_PLACEMENT_3D ( 'NONE', #77834, #25748, #1143 ) ;
#13274=VERTEX_POINT ( 'NONE', #56819 ) ;
#13278=ADVANCED_FACE ( 'NONE', ( #106651 ), #82881, .T. ) ;
#13288=VERTEX_POINT ( 'NONE', #46585 ) ;
#13297=DIRECTION ( 'NONE',  ( 0.1070030146457354309, 0.000000000000000000, 0.9942586961433751425 ) ) ;
#13303=ORIENTED_EDGE ( 'NONE', *, *, #92101, .T. ) ;
#13310=LINE ( 'NONE', #12789, #28175 ) ;
#13324=PLANE ( 'NONE',  #65795 ) ;
#13329=ADVANCED_FACE ( 'NONE', ( #88578 ), #43404, .T. ) ;
#13345=VERTEX_POINT ( 'NONE', #54986 ) ;
#13353=FACE_OUTER_BOUND ( 'NONE', #106258, .T. ) ;
#13365=CARTESIAN_POINT ( 'NONE',  ( 17.43739734485841808, 1526.178928173327449, 237.5162751070522518 ) ) ;
#13406=CARTESIAN_POINT ( 'NONE',  ( -30.31940284292426924, 1523.382868172864164, 195.7503880523418616 ) ) ;
#13420=CARTESIAN_POINT ( 'NONE',  ( 0.7251570665222378809, 1526.278758871496620, 176.2636429491667514 ) ) ;
#13430=CARTESIAN_POINT ( 'NONE',  ( 30.44069153016972251, 1525.425686270224332, 196.7701993420686506 ) ) ;
#13439=AXIS2_PLACEMENT_3D ( 'NONE', #66230, #76804, #74614 ) ;
#13458=CARTESIAN_POINT ( 'NONE',  ( 31.44837959398582328, 1512.187213306747481, 197.3353852117981262 ) ) ;
#13477=CARTESIAN_POINT ( 'NONE',  ( -17.03783583027061255, 1524.776010967693765, 181.0919469249481040 ) ) ;
#13484=CARTESIAN_POINT ( 'NONE',  ( -16.66936639845610202, 1523.382868172864164, 237.7608804993221838 ) ) ;
#13491=CARTESIAN_POINT ( 'NONE',  ( 1.689251544526525040, 1526.344110814223313, 178.4720708657796422 ) ) ;
#13498=EDGE_CURVE ( 'NONE', #11721, #42444, #95108, .T. ) ;
#13500=DIRECTION ( 'NONE',  ( -0.2054769195713317398, -1.225281874271768203E-16, -0.9786619618251628516 ) ) ;
#13512=CARTESIAN_POINT ( 'NONE',  ( 16.73628186595838940, 1526.382868172863937, 234.1845039693043589 ) ) ;
#13527=DIRECTION ( 'NONE',  ( -0.000000000000000000, -1.000000000000000000, -0.000000000000000000 ) ) ;
#13543=ORIENTED_EDGE ( 'NONE', *, *, #100654, .F. ) ;
#13544=ORIENTED_EDGE ( 'NONE', *, *, #64856, .T. ) ;
#13562=CARTESIAN_POINT ( 'NONE',  ( -17.61555691395482626, 1524.600389084707103, 180.6475253884790391 ) ) ;
#13570=DIRECTION ( 'NONE',  ( -0.7882878497004317531, 0.000000000000000000, -0.6153066438895888890 ) ) ;
#13571=CARTESIAN_POINT ( 'NONE',  ( -21.19880661589021642, 1526.382868172863937, 184.6948938244649696 ) ) ;
#13577=AXIS2_PLACEMENT_3D ( 'NONE', #69519, #71170, #60003 ) ;
#13582=CARTESIAN_POINT ( 'NONE',  ( 29.41653834769454079, 1525.790287071785542, 221.5659752742948569 ) ) ;
#13585=CARTESIAN_POINT ( 'NONE',  ( -1.389373685237467404, 1526.382868173645647, 178.7050053866561541 ) ) ;
#13590=CARTESIAN_POINT ( 'NONE',  ( 17.04790460295257049, 1526.208281990536761, 182.6359253440253667 ) ) ;
#13607=DIRECTION ( 'NONE',  ( 0.000000000000000000, 0.000000000000000000, -1.000000000000000000 ) ) ;
#13618=CARTESIAN_POINT ( 'NONE',  ( 1.191524307911315805, 1526.382868172863937, 239.2353018730792087 ) ) ;
#13620=LINE ( 'NONE', #79901, #14253 ) ;
#13624=CARTESIAN_POINT ( 'NONE',  ( 31.14814740298836071, 1525.697946996672272, 216.7341141171428944 ) ) ;
#13635=CARTESIAN_POINT ( 'NONE',  ( -32.28466283162143213, 1522.382868172863937, 219.1752493337717738 ) ) ;
#13664=CARTESIAN_POINT ( 'NONE',  ( -16.64885258016628100, 1526.344110814221949, 183.3327398900398748 ) ) ;
#13671=CARTESIAN_POINT ( 'NONE',  ( -28.27139721233049485, 1526.382868172864164, 198.6830693683576499 ) ) ;
#13673=CARTESIAN_POINT ( 'NONE',  ( 31.23437356469446868, 1512.187213306747481, 221.8968241038843701 ) ) ;
#13679=ADVANCED_FACE ( 'NONE', ( #83453 ), #33053, .T. ) ;
#13686=EDGE_CURVE ( 'NONE', #92019, #4978, #24800, .T. ) ;
#13690=CARTESIAN_POINT ( 'NONE',  ( 2.485500793217951809, 1524.600389084707103, 175.7314721497423591 ) ) ;
#13712=CARTESIAN_POINT ( 'NONE',  ( 30.31940284289168375, 1523.456924617338018, 195.7503880522679651 ) ) ;
#13717=EDGE_CURVE ( 'NONE', #75960, #97242, #94317, .T. ) ;
#13719=CARTESIAN_POINT ( 'NONE',  ( -31.23437356469455040, 1512.187213306747481, 197.3468678195118287 ) ) ;
#13723=CARTESIAN_POINT ( 'NONE',  ( 33.82780500856144101, 1523.429859730330691, 220.5611772381395213 ) ) ;
#13728=CARTESIAN_POINT ( 'NONE',  ( 21.83863730836035444, 1523.580203803270933, 234.9763103460704770 ) ) ;
#13733=( BOUNDED_CURVE ( )  B_SPLINE_CURVE ( 3, ( #48850, #91383, #99759, #50494 ),
 .UNSPECIFIED., .F., .T. ) 
 B_SPLINE_CURVE_WITH_KNOTS ( ( 4, 4 ),
 ( 0.000000000000000000, 0.7048113239778029948 ),
 .UNSPECIFIED. ) 
 CURVE ( )  GEOMETRIC_REPRESENTATION_ITEM ( )  RATIONAL_B_SPLINE_CURVE ( ( 1.000000000000000000, 0.9590300661663095916, 0.9590300661663095916, 1.000000000000000000 ) ) 
 REPRESENTATION_ITEM ( '' )  );
#13744=ORIENTED_EDGE ( 'NONE', *, *, #13498, .T. ) ;
#13757=DIRECTION ( 'NONE',  ( 0.000000000000000000, 1.000000000000000000, 0.000000000000000000 ) ) ;
#13768=CARTESIAN_POINT ( 'NONE',  ( -19.02270174366725541, 1526.382868172864164, 232.8547275633879678 ) ) ;
#13794=EDGE_CURVE ( 'NONE', #82045, #108700, #12353, .T. ) ;
#13802=DIRECTION ( 'NONE',  ( -0.000000000000000000, -1.000000000000000000, -0.000000000000000000 ) ) ;
#13821=CARTESIAN_POINT ( 'NONE',  ( -17.29882006758230162, 1523.542365884046376, 180.8528181918347570 ) ) ;
#13824=VERTEX_POINT ( 'NONE', #10974 ) ;
#13827=EDGE_CURVE ( 'NONE', #44756, #30516, #2598, .T. ) ;
#13851=CARTESIAN_POINT ( 'NONE',  ( 29.99620953741488449, 1524.382868172863937, 198.4974435154498735 ) ) ;
#13852=CARTESIAN_POINT ( 'NONE',  ( 32.85805783624306287, 1523.678648413191695, 201.0453875934054224 ) ) ;
#13856=AXIS2_PLACEMENT_3D ( 'NONE', #75878, #8105, #59092 ) ;
#13861=DIRECTION ( 'NONE',  ( 0.000000000000000000, 1.000000000000000000, 0.000000000000000000 ) ) ;
#13873=CARTESIAN_POINT ( 'NONE',  ( 20.71343476517513338, 1512.187213306747481, 179.9059455038194528 ) ) ;
#13874=VERTEX_POINT ( 'NONE', #29410 ) ;
#13879=DIRECTION ( 'NONE',  ( -0.000000000000000000, -1.000000000000000000, -0.000000000000000000 ) ) ;
#13884=CARTESIAN_POINT ( 'NONE',  ( -16.73628186595804834, 1526.382868172864164, 234.1845039693045862 ) ) ;
#13886=CARTESIAN_POINT ( 'NONE',  ( -31.34137657934000387, 1523.382868172864164, 221.9025654077414345 ) ) ;
#13888=CIRCLE ( 'NONE', #71175, 0.9999999999999309441 ) ;
#13889=DIRECTION ( 'NONE',  ( 0.4090087482554486953, 0.000000000000000000, 0.9125304618753892205 ) ) ;
#13894=VERTEX_POINT ( 'NONE', #61958 ) ;
#13898=CARTESIAN_POINT ( 'NONE',  ( -31.11295512654738715, 1525.790287071770535, 216.3449412819151689 ) ) ;
#13899=VERTEX_POINT ( 'NONE', #72016 ) ;
#13907=ADVANCED_FACE ( 'NONE', ( #97727 ), #12625, .T. ) ;
#13910=TOROIDAL_SURFACE ( 'NONE', #12175, 1.000000000000000000, 1.000000000000000000 ) ;
#13915=CYLINDRICAL_SURFACE ( 'NONE', #30510, 1.000000000000000888 ) ;
#13924=FACE_OUTER_BOUND ( 'NONE', #108589, .T. ) ;
#13932=DIRECTION ( 'NONE',  ( 0.8672669759446689497, 0.000000000000000000, 0.4978433412588633700 ) ) ;
#13954=CARTESIAN_POINT ( 'NONE',  ( 16.66936639838844059, 1523.456924617337791, 237.7608804993615479 ) ) ;
#13957=EDGE_LOOP ( 'NONE', ( #67593, #35701, #36155, #30049 ) ) ;
#13966=AXIS2_PLACEMENT_3D ( 'NONE', #29770, #45511, #96998 ) ;
#13979=ORIENTED_EDGE ( 'NONE', *, *, #55066, .T. ) ;
#13994=AXIS2_PLACEMENT_3D ( 'NONE', #69347, #69908, #1584 ) ;
#13996=EDGE_CURVE ( 'NONE', #36754, #29937, #105326, .T. ) ;
#14007=CARTESIAN_POINT ( 'NONE',  ( 16.48231778833692118, 1525.661275128775515, 236.6690309048151732 ) ) ;
#14011=DIRECTION ( 'NONE',  ( -0.8672669759446595128, 0.000000000000000000, 0.4978433412588795237 ) ) ;
#14015=CARTESIAN_POINT ( 'NONE',  ( -32.39800393421789693, 1524.816548299036867, 201.1912629570496733 ) ) ;
#14016=FACE_OUTER_BOUND ( 'NONE', #57925, .T. ) ;
#14021=DIRECTION ( 'NONE',  ( -0.2054769195713179730, -0.000000000000000000, -0.9786619618251657382 ) ) ;
#14024=DIRECTION ( 'NONE',  ( 0.1070030146457371656, 0.000000000000000000, 0.9942586961433751425 ) ) ;
#14029=DIRECTION ( 'NONE',  ( 0.000000000000000000, 1.000000000000000000, 0.000000000000000000 ) ) ;
#14034=CARTESIAN_POINT ( 'NONE',  ( -16.48400375142206897, 1525.790287071779403, 181.7637264533375685 ) ) ;
#14039=DIRECTION ( 'NONE',  ( 0.9125304618754024322, 0.000000000000000000, -0.4090087482554191078 ) ) ;
#14040=DIRECTION ( 'NONE',  ( 0.5877852522924807976, 0.000000000000000000, 0.8090169943749417891 ) ) ;
#14042=AXIS2_PLACEMENT_3D ( 'NONE', #108566, #14493, #15034 ) ;
#14047=CARTESIAN_POINT ( 'NONE',  ( -18.72690275718909092, 1526.278758871498894, 236.1309272327495421 ) ) ;
#14049=AXIS2_PLACEMENT_3D ( 'NONE', #64050, #98168, #21440 ) ;
#14071=CARTESIAN_POINT ( 'NONE',  ( 0.000000000000000000, 1512.187213306747481, 209.1218459616979999 ) ) ;
#14080=EDGE_LOOP ( 'NONE', ( #57181, #8333, #72917, #4343, #107975 ) ) ;
#14081=ORIENTED_EDGE ( 'NONE', *, *, #78951, .T. ) ;
#14083=EDGE_LOOP ( 'NONE', ( #10847, #85734, #31084, #47666 ) ) ;
#14091=DIRECTION ( 'NONE',  ( -0.000000000000000000, -1.000000000000000000, -0.000000000000000000 ) ) ;
#14093=ADVANCED_FACE ( 'NONE', ( #76953 ), #51192, .T. ) ;
#14102=CARTESIAN_POINT ( 'NONE',  ( 31.12456774391177206, 1525.960063244516959, 217.0912716842394730 ) ) ;
#14131=CARTESIAN_POINT ( 'NONE',  ( -21.86721050905450525, 1523.611961620354123, 183.2036325349451715 ) ) ;
#14136=EDGE_CURVE ( 'NONE', #97990, #109192, #60157, .T. ) ;
#14143=CARTESIAN_POINT ( 'NONE',  ( 31.32995031131198616, 1523.678648413191695, 221.9013357025044115 ) ) ;
#14150=CARTESIAN_POINT ( 'NONE',  ( -1.338895077078837259, 1526.382868172864164, 178.6697305272290635 ) ) ;
#14162=AXIS2_PLACEMENT_3D ( 'NONE', #37837, #105040, #79846 ) ;
#14190=CARTESIAN_POINT ( 'NONE',  ( 31.56778878607238781, 1525.408337840050308, 216.2063969590453496 ) ) ;
#14200=( BOUNDED_CURVE ( )  B_SPLINE_CURVE ( 3, ( #12427, #46617, #104844, #90224 ),
 .UNSPECIFIED., .F., .T. ) 
 B_SPLINE_CURVE_WITH_KNOTS ( ( 4, 4 ),
 ( 4.712388980384689674, 6.283185307179586232 ),
 .UNSPECIFIED. ) 
 CURVE ( )  GEOMETRIC_REPRESENTATION_ITEM ( )  RATIONAL_B_SPLINE_CURVE ( ( 1.000000000000000000, 0.8047378541243649375, 0.8047378541243649375, 1.000000000000000000 ) ) 
 REPRESENTATION_ITEM ( '' )  );
#14205=DIRECTION ( 'NONE',  ( 0.000000000000000000, 0.000000000000000000, 1.000000000000000000 ) ) ;
#14213=AXIS2_PLACEMENT_3D ( 'NONE', #72876, #56624, #30300 ) ;
#14216=ORIENTED_EDGE ( 'NONE', *, *, #52118, .F. ) ;
#14235=CARTESIAN_POINT ( 'NONE',  ( 22.08523692261549698, 1523.530935881284904, 184.4211863326289915 ) ) ;
#14242=CARTESIAN_POINT ( 'NONE',  ( 29.99620953741487384, 1526.382868172863937, 198.4974435154498735 ) ) ;
#14245=ORIENTED_EDGE ( 'NONE', *, *, #67201, .T. ) ;
#14253=VECTOR ( 'NONE', #98751, 1000.000000000000000 ) ;
#14281=CIRCLE ( 'NONE', #80406, 0.9999999999999974465 ) ;
#14284=DIRECTION ( 'NONE',  ( 0.000000000000000000, 0.000000000000000000, 1.000000000000000000 ) ) ;
#14286=DIRECTION ( 'NONE',  ( -0.000000000000000000, -1.000000000000000000, -0.000000000000000000 ) ) ;
#14288=CARTESIAN_POINT ( 'NONE',  ( 32.09235212275375915, 1525.402221411349956, 221.9833860708131397 ) ) ;
#14289=ORIENTED_EDGE ( 'NONE', *, *, #59852, .F. ) ;
#14300=LINE ( 'NONE', #82629, #5638 ) ;
#14304=CARTESIAN_POINT ( 'NONE',  ( 17.19739463999625784, 1525.960063244516959, 181.9833109756548595 ) ) ;
#14311=AXIS2_PLACEMENT_3D ( 'NONE', #40502, #99845, #29889 ) ;
#14316=DIRECTION ( 'NONE',  ( 0.000000000000000000, 0.000000000000000000, 1.000000000000000000 ) ) ;
#14327=ORIENTED_EDGE ( 'NONE', *, *, #47380, .T. ) ;
#14328=EDGE_CURVE ( 'NONE', #6825, #20574, #43899, .T. ) ;
#14352=AXIS2_PLACEMENT_3D ( 'NONE', #37003, #38106, #20734 ) ;
#14374=EDGE_CURVE ( 'NONE', #64042, #50617, #51784, .T. ) ;
#14378=CARTESIAN_POINT ( 'NONE',  ( -16.66936639839001444, 1523.456924617335972, 180.4828114240353329 ) ) ;
#14384=CARTESIAN_POINT ( 'NONE',  ( -28.27139721233027458, 1526.382868172864164, 219.5606225550389468 ) ) ;
#14400=FACE_OUTER_BOUND ( 'NONE', #85668, .T. ) ;
#14406=LINE ( 'NONE', #55902, #62519 ) ;
#14408=CARTESIAN_POINT ( 'NONE',  ( 30.31940284292419108, 1523.382868172864164, 222.4933038710543372 ) ) ;
#14414=ORIENTED_EDGE ( 'NONE', *, *, #56853, .T. ) ;
#14416=DIRECTION ( 'NONE',  ( 0.000000000000000000, 0.000000000000000000, 1.000000000000000000 ) ) ;
#14429=DIRECTION ( 'NONE',  ( 0.3090169943749446757, 0.000000000000000000, -0.9510565162951544194 ) ) ;
#14453=CARTESIAN_POINT ( 'NONE',  ( 33.23421991949457066, 1522.906363951597314, 217.4142352873253685 ) ) ;
#14455=ADVANCED_FACE ( 'NONE', ( #18668 ), #2354, .T. ) ;
#14476=CARTESIAN_POINT ( 'NONE',  ( -20.91563475928094462, 1525.795403383247276, 184.9927169682721910 ) ) ;
#14480=VECTOR ( 'NONE', #44496, 1000.000000000000000 ) ;
#14481=DIRECTION ( 'NONE',  ( -0.6709778558543730842, 0.000000000000000000, -0.7414773880254664773 ) ) ;
#14482=CARTESIAN_POINT ( 'NONE',  ( -33.93019615848550785, 1522.906561336852519, 220.5829544588085014 ) ) ;
#14485=EDGE_CURVE ( 'NONE', #79230, #18078, #14690, .T. ) ;
#14493=DIRECTION ( 'NONE',  ( 0.000000000000000000, 1.000000000000000000, 0.000000000000000000 ) ) ;
#14496=TOROIDAL_SURFACE ( 'NONE', #87913, 2.000000000000000000, 1.000000000000000000 ) ;
#14510=CARTESIAN_POINT ( 'NONE',  ( 17.29393938232482597, 1523.621879633028584, 237.3864571009499969 ) ) ;
#14529=CIRCLE ( 'NONE', #100391, 1.000000000000002442 ) ;
#14530=ORIENTED_EDGE ( 'NONE', *, *, #39541, .T. ) ;
#14549=CIRCLE ( 'NONE', #55759, 32.13701971169416538 ) ;
#14559=ORIENTED_EDGE ( 'NONE', *, *, #20753, .T. ) ;
#14567=CARTESIAN_POINT ( 'NONE',  ( -30.31118248177353536, 1526.186458717539381, 201.5497466985122799 ) ) ;
#14594=CARTESIAN_POINT ( 'NONE',  ( -16.99775931995139189, 1524.964230758882877, 181.1932721696053079 ) ) ;
#14595=CARTESIAN_POINT ( 'NONE',  ( 2.470168522033036496, 1523.481610118015169, 175.3649660273507607 ) ) ;
#14603=CARTESIAN_POINT ( 'NONE',  ( 2.372478608332516892, 1522.862737210649811, 243.3440112565233449 ) ) ;
#14626=CARTESIAN_POINT ( 'NONE',  ( -20.71343476517554905, 1501.977400791986611, 179.9059455038197086 ) ) ;
#14637=DIRECTION ( 'NONE',  ( 0.4882662618185301118, -0.4884709562387606896, -0.7231819843448463736 ) ) ;
#14649=CARTESIAN_POINT ( 'NONE',  ( -17.83486663330526767, 1523.678648413191695, 180.3677388339002334 ) ) ;
#14652=CARTESIAN_POINT ( 'NONE',  ( 32.02808312589922224, 1511.187213306747708, 219.9649204700462235 ) ) ;
#14656=DIRECTION ( 'NONE',  ( 0.000000000000000000, 0.000000000000000000, -1.000000000000000000 ) ) ;
#14667=DIRECTION ( 'NONE',  ( -0.000000000000000000, -1.000000000000000000, -0.000000000000000000 ) ) ;
#14674=ORIENTED_EDGE ( 'NONE', *, *, #78062, .T. ) ;
#14675=VECTOR ( 'NONE', #55034, 1000.000000000000000 ) ;
#14683=DIRECTION ( 'NONE',  ( 0.000000000000000000, 0.000000000000000000, 1.000000000000000000 ) ) ;
#14690=LINE ( 'NONE', #83004, #75042 ) ;
#14704=FACE_OUTER_BOUND ( 'NONE', #34723, .T. ) ;
#14711=CARTESIAN_POINT ( 'NONE',  ( 16.53175237172159839, 1526.069472839387117, 182.3016483747060761 ) ) ;
#14716=VERTEX_POINT ( 'NONE', #77238 ) ;
#14720=LINE ( 'NONE', #83038, #58552 ) ;
#14734=DIRECTION ( 'NONE',  ( 0.9125304618753967700, 0.000000000000000000, -0.4090087482554317089 ) ) ;
#14747=CARTESIAN_POINT ( 'NONE',  ( 31.54872587855177102, 1525.317359687841190, 216.6695404376949057 ) ) ;
#14753=CARTESIAN_POINT ( 'NONE',  ( -2.372478608332516892, 1501.977400791986611, 243.3440112565233449 ) ) ;
#14758=CARTESIAN_POINT ( 'NONE',  ( 17.24701803731020888, 1523.844789899202851, 237.3932575341077325 ) ) ;
#14786=( NAMED_UNIT ( * ) PLANE_ANGLE_UNIT ( ) SI_UNIT ( $, .RADIAN. ) );
#14790=CARTESIAN_POINT ( 'NONE',  ( 30.31940284292409515, 1523.382868172864164, 195.7503880523414352 ) ) ;
#14838=FACE_OUTER_BOUND ( 'NONE', #98381, .T. ) ;
#14845=CARTESIAN_POINT ( 'NONE',  ( -1.491506560153235128, 1512.187213306747481, 175.5704429466618421 ) ) ;
#14861=CARTESIAN_POINT ( 'NONE',  ( 32.72607202732672249, 1524.152444737676660, 201.1104170367456732 ) ) ;
#14869=EDGE_CURVE ( 'NONE', #68723, #32820, #14406, .T. ) ;
#14876=EDGE_CURVE ( 'NONE', #14943, #108182, #100035, .T. ) ;
#14877=ORIENTED_EDGE ( 'NONE', *, *, #31065, .F. ) ;
#14892=CARTESIAN_POINT ( 'NONE',  ( 34.61172972909988488, 1523.342713519622748, 200.0387150244870043 ) ) ;
#14894=EDGE_LOOP ( 'NONE', ( #22705, #108452, #19846, #29392 ) ) ;
#14910=CARTESIAN_POINT ( 'NONE',  ( -22.03465957474532999, 1512.187213306747481, 235.4136513321633117 ) ) ;
#14915=CARTESIAN_POINT ( 'NONE',  ( 33.28034951413924603, 1522.382868172863937, 200.8029765415137433 ) ) ;
#14923=DIRECTION ( 'NONE',  ( -0.000000000000000000, -1.000000000000000000, -0.000000000000000000 ) ) ;
#14928=CARTESIAN_POINT ( 'NONE',  ( 29.86461515634908892, 1525.960063244516959, 197.2746849027934957 ) ) ;
#14929=ORIENTED_EDGE ( 'NONE', *, *, #359, .F. ) ;
#14930=EDGE_LOOP ( 'NONE', ( #171, #105307, #52537, #19094 ) ) ;
#14941=CARTESIAN_POINT ( 'NONE',  ( -20.71343476517491311, 1522.382868172863937, 238.3377464195766890 ) ) ;
#14943=VERTEX_POINT ( 'NONE', #31223 ) ;
#14946=CARTESIAN_POINT ( 'NONE',  ( 34.77865709045956066, 1512.187213306747481, 191.3609956664886624 ) ) ;
#14970=CARTESIAN_POINT ( 'NONE',  ( -31.50799703744299762, 1524.382868172863937, 201.8203724569136739 ) ) ;
#14978=PLANE ( 'NONE',  #60007 ) ;
#14986=CARTESIAN_POINT ( 'NONE',  ( -18.19590854888122422, 1522.862737210649584, 238.2026672068776634 ) ) ;
#14995=ORIENTED_EDGE ( 'NONE', *, *, #101680, .T. ) ;
#15034=DIRECTION ( 'NONE',  ( -0.9510565162951566398, 0.000000000000000000, -0.3090169943749382919 ) ) ;
#15037=VERTEX_POINT ( 'NONE', #102681 ) ;
#15042=B_SPLINE_CURVE_WITH_KNOTS ( 'NONE', 3,
 ( #78111, #23962, #69749, #87067 ),
 .UNSPECIFIED., .F., .F.,
 ( 4, 4 ),
 ( 0.000000000000000000, 0.0002220129587134776663 ),
 .UNSPECIFIED. ) ;
#15051=CARTESIAN_POINT ( 'NONE',  ( 17.84054674791004302, 1523.580204110583509, 237.8810931398604680 ) ) ;
#15069=EDGE_LOOP ( 'NONE', ( #72372, #80247, #49966, #52840, #36696 ) ) ;
#15094=CIRCLE ( 'NONE', #65172, 1.000000000000000888 ) ;
#15102=CYLINDRICAL_SURFACE ( 'NONE', #78145, 1.000000000000000888 ) ;
#15110=CARTESIAN_POINT ( 'NONE',  ( -29.00779973304138437, 1526.382868172864164, 200.9494832830839073 ) ) ;
#15112=ADVANCED_FACE ( 'NONE', ( #64045 ), #51716, .F. ) ;
#15115=FACE_OUTER_BOUND ( 'NONE', #16765, .T. ) ;
#15117=CARTESIAN_POINT ( 'NONE',  ( 0.4151546846821903003, 1501.977400791986611, 242.9330574173806951 ) ) ;
#15119=DIRECTION ( 'NONE',  ( -0.1010290445074252530, 0.000000000000000000, 0.9948834766775036531 ) ) ;
#15121=CARTESIAN_POINT ( 'NONE',  ( -2.127574403379840273, 1524.244163922423468, 173.7332312662362597 ) ) ;
#15122=CYLINDRICAL_SURFACE ( 'NONE', #81365, 2.000000000000003553 ) ;
#15133=CARTESIAN_POINT ( 'NONE',  ( -16.51370421206452122, 1525.137906803775877, 181.0453479566121189 ) ) ;
#15164=CARTESIAN_POINT ( 'NONE',  ( -29.00779973304124582, 1526.382868172864164, 217.2942086403127178 ) ) ;
#15192=EDGE_LOOP ( 'NONE', ( #57609, #17924, #5711, #84064 ) ) ;
#15198=DIRECTION ( 'NONE',  ( 0.000000000000000000, 0.000000000000000000, -1.000000000000000000 ) ) ;
#15203=AXIS2_PLACEMENT_3D ( 'NONE', #15481, #110115, #71342 ) ;
#15208=ORIENTED_EDGE ( 'NONE', *, *, #20041, .T. ) ;
#15213=EDGE_CURVE ( 'NONE', #75901, #29531, #53550, .T. ) ;
#15218=CARTESIAN_POINT ( 'NONE',  ( 20.91563475928075988, 1525.795403383247276, 233.2509749551239224 ) ) ;
#15224=CARTESIAN_POINT ( 'NONE',  ( -21.38516915558008336, 1522.382868172863937, 180.3939891059723664 ) ) ;
#15233=ADVANCED_FACE ( 'NONE', ( #20754 ), #10736, .T. ) ;
#15242=CARTESIAN_POINT ( 'NONE',  ( -1.191524307911313363, 1526.382868172864164, 179.0083900503168479 ) ) ;
#15282=CARTESIAN_POINT ( 'NONE',  ( 32.18358323225305639, 1524.059547553519224, 216.7473625276872156 ) ) ;
#15284=CIRCLE ( 'NONE', #67123, 1.000000000000000888 ) ;
#15294=VECTOR ( 'NONE', #107907, 1000.000000000000000 ) ;
#15311=EDGE_LOOP ( 'NONE', ( #68517, #59588, #40223, #79630 ) ) ;
#15315=ORIENTED_EDGE ( 'NONE', *, *, #53430, .F. ) ;
#15380=EDGE_CURVE ( 'NONE', #85956, #15491, #64789, .T. ) ;
#15383=CARTESIAN_POINT ( 'NONE',  ( -0.8350686643532192477, 1526.382868172863937, 177.3106345060153046 ) ) ;
#15384=CYLINDRICAL_SURFACE ( 'NONE', #50079, 1.000000000000000888 ) ;
#15392=CARTESIAN_POINT ( 'NONE',  ( -20.49599333844833993, 1525.960063244516959, 233.8638087104925489 ) ) ;
#15432=DIRECTION ( 'NONE',  ( 0.000000000000000000, 1.000000000000000000, 0.000000000000000000 ) ) ;
#15450=CARTESIAN_POINT ( 'NONE',  ( 1.912903644476265042, 1526.104292489129193, 240.8844628569918882 ) ) ;
#15452=DIRECTION ( 'NONE',  ( -5.329070518200752183E-15, 0.000000000000000000, -1.000000000000000000 ) ) ;
#15453=CARTESIAN_POINT ( 'NONE',  ( -33.42844755917204225, 1522.382868172863937, 196.1165140606796058 ) ) ;
#15458=CARTESIAN_POINT ( 'NONE',  ( 0.000000000000000000, 1523.051704408389696, 233.8211094035767985 ) ) ;
#15466=CARTESIAN_POINT ( 'NONE',  ( 0.000000000000000000, 1512.187213306747481, 209.1218459616979999 ) ) ;
#15472=EDGE_CURVE ( 'NONE', #90117, #81438, #88400, .T. ) ;
#15481=CARTESIAN_POINT ( 'NONE',  ( -31.23437356469455040, 1511.187213306747708, 195.3468678195118287 ) ) ;
#15488=DIRECTION ( 'NONE',  ( 0.000000000000000000, 1.000000000000000000, 0.000000000000000000 ) ) ;
#15491=VERTEX_POINT ( 'NONE', #71082 ) ;
#15495=ORIENTED_EDGE ( 'NONE', *, *, #13498, .F. ) ;
#15499=CARTESIAN_POINT ( 'NONE',  ( 17.12015143466563671, 1526.107880201381477, 182.3088744090234172 ) ) ;
#15502=CARTESIAN_POINT ( 'NONE',  ( 0.000000000000000000, 1523.382868172864164, 209.1218459616979999 ) ) ;
#15515=CARTESIAN_POINT ( 'NONE',  ( 3.237065521149570912, 1524.843416604498543, 176.5220937283001774 ) ) ;
#15521=CARTESIAN_POINT ( 'NONE',  ( -32.02808312589908013, 1512.187213306747481, 220.9649204700466782 ) ) ;
#15522=DIRECTION ( 'NONE',  ( 0.000000000000000000, 0.000000000000000000, -1.000000000000000000 ) ) ;
#15527=ORIENTED_EDGE ( 'NONE', *, *, #90425, .F. ) ;
#15543=CARTESIAN_POINT ( 'NONE',  ( 19.53786426059039982, 1512.187213306747481, 237.7197124308265188 ) ) ;
#15547=ORIENTED_EDGE ( 'NONE', *, *, #110208, .T. ) ;
#15550=LINE ( 'NONE', #41883, #26282 ) ;
#15551=CYLINDRICAL_SURFACE ( 'NONE', #16216, 1.999999999999998668 ) ;
#15555=CARTESIAN_POINT ( 'NONE',  ( -18.19590854888121356, 1522.382868172863937, 238.2026672068777202 ) ) ;
#15562=AXIS2_PLACEMENT_3D ( 'NONE', #61471, #60921, #1008 ) ;
#15586=DIRECTION ( 'NONE',  ( -0.000000000000000000, -1.000000000000000000, -0.000000000000000000 ) ) ;
#15593=CARTESIAN_POINT ( 'NONE',  ( 17.84338787552646366, 1523.481610118012441, 237.8836641335914237 ) ) ;
#15596=VERTEX_POINT ( 'NONE', #23383 ) ;
#15642=CARTESIAN_POINT ( 'NONE',  ( 31.81407709660769001, 1522.382868172863937, 196.2902540610627682 ) ) ;
#15669=ORIENTED_EDGE ( 'NONE', *, *, #20964, .F. ) ;
#15670=CARTESIAN_POINT ( 'NONE',  ( -17.34064885126208466, 1525.506916460679804, 181.3217002936585516 ) ) ;
#15689=EDGE_CURVE ( 'NONE', #23328, #13274, #68249, .T. ) ;
#15714=AXIS2_PLACEMENT_3D ( 'NONE', #86137, #101811, #51997 ) ;
#15743=ORIENTED_EDGE ( 'NONE', *, *, #32296, .F. ) ;
#15746=ORIENTED_EDGE ( 'NONE', *, *, #21409, .T. ) ;
#15768=CARTESIAN_POINT ( 'NONE',  ( -21.80586012576711852, 1523.954924407825956, 234.9031818917333112 ) ) ;
#15771=LINE ( 'NONE', #66794, #63523 ) ;
#15773=ORIENTED_EDGE ( 'NONE', *, *, #27051, .T. ) ;
#15792=VECTOR ( 'NONE', #34654, 1000.000000000000000 ) ;
#15808=AXIS2_PLACEMENT_3D ( 'NONE', #45527, #2973, #79668 ) ;
#15827=EDGE_CURVE ( 'NONE', #54724, #49707, #14300, .T. ) ;
#15834=CARTESIAN_POINT ( 'NONE',  ( 17.12660205615345888, 1524.374578187333555, 237.3020490138461867 ) ) ;
#15838=CARTESIAN_POINT ( 'NONE',  ( -33.35590117750189876, 1523.678648413191695, 216.3310373540461171 ) ) ;
#15849=ORIENTED_EDGE ( 'NONE', *, *, #40174, .T. ) ;
#15855=FACE_OUTER_BOUND ( 'NONE', #59873, .T. ) ;
#15862=LINE ( 'NONE', #50067, #47650 ) ;
#15883=ORIENTED_EDGE ( 'NONE', *, *, #22127, .F. ) ;
#15889=ORIENTED_EDGE ( 'NONE', *, *, #60493, .F. ) ;
#15913=CARTESIAN_POINT ( 'NONE',  ( 17.19739463999625784, 1525.960063244516959, 181.9833109756548595 ) ) ;
#15934=CARTESIAN_POINT ( 'NONE',  ( -31.50799703744286262, 1524.382868172863937, 216.4233194664829796 ) ) ;
#15961=VECTOR ( 'NONE', #78246, 1000.000000000000000 ) ;
#15968=EDGE_CURVE ( 'NONE', #66900, #90799, #79758, .T. ) ;
#15990=VERTEX_POINT ( 'NONE', #66129 ) ;
#16005=ORIENTED_EDGE ( 'NONE', *, *, #104995, .F. ) ;
#16006=CARTESIAN_POINT ( 'NONE',  ( 2.404980717409123336, 1525.211477436245787, 242.0950474068928884 ) ) ;
#16028=CARTESIAN_POINT ( 'NONE',  ( 31.32995031131189378, 1523.678648413191695, 196.3423562208913324 ) ) ;
#16032=CARTESIAN_POINT ( 'NONE',  ( -28.62766089293190674, 1526.344110814220357, 220.1997210291906129 ) ) ;
#16036=CIRCLE ( 'NONE', #94795, 1.000000000000000888 ) ;
#16039=DIRECTION ( 'NONE',  ( 0.000000000000000000, 0.000000000000000000, 1.000000000000000000 ) ) ;
#16048=CARTESIAN_POINT ( 'NONE',  ( -3.300164695495766853, 1524.538768545233779, 241.8639374637165815 ) ) ;
#16074=CARTESIAN_POINT ( 'NONE',  ( 17.17241001986506888, 1523.382868172864164, 237.6251415217915053 ) ) ;
#16079=ORIENTED_EDGE ( 'NONE', *, *, #3941, .T. ) ;
#16080=CARTESIAN_POINT ( 'NONE',  ( 29.13504683812232798, 1526.073434386619056, 221.0961479590759495 ) ) ;
#16082=CARTESIAN_POINT ( 'NONE',  ( -2.596261494520225366, 1525.907212628473644, 177.4701144822246874 ) ) ;
#16084=CARTESIAN_POINT ( 'NONE',  ( -18.07041998555256868, 1523.313115944345100, 238.0891100728149183 ) ) ;
#16094=CARTESIAN_POINT ( 'NONE',  ( 34.68852446352944696, 1522.382868172863937, 218.2490599186007216 ) ) ;
#16106=CARTESIAN_POINT ( 'NONE',  ( 31.33756689035249110, 1523.580203803270933, 196.3415365178082368 ) ) ;
#16118=AXIS2_PLACEMENT_3D ( 'NONE', #37124, #86419, #53965 ) ;
#16123=CARTESIAN_POINT ( 'NONE',  ( 16.87900699709421204, 1524.382868172804365, 237.0109764097478546 ) ) ;
#16147=CARTESIAN_POINT ( 'NONE',  ( -2.136371660471462874, 1525.856064936157054, 176.8742965270300544 ) ) ;
#16148=DIRECTION ( 'NONE',  ( 0.2054769195713296581, -0.000000000000000000, 0.9786619618251632957 ) ) ;
#16150=CARTESIAN_POINT ( 'NONE',  ( -3.350338079455601026, 1523.604703353109699, 176.1628856388066708 ) ) ;
#16156=CARTESIAN_POINT ( 'NONE',  ( 17.83486663330510424, 1523.678648413191695, 237.8759530894959084 ) ) ;
#16162=ORIENTED_EDGE ( 'NONE', *, *, #45458, .T. ) ;
#16187=CARTESIAN_POINT ( 'NONE',  ( 28.27139721233048419, 1526.382868172863937, 219.5606225550385489 ) ) ;
#16188=CARTESIAN_POINT ( 'NONE',  ( -16.58770733237527395, 1524.425415513989265, 180.6486613107830976 ) ) ;
#16191=ORIENTED_EDGE ( 'NONE', *, *, #46375, .F. ) ;
#16192=CARTESIAN_POINT ( 'NONE',  ( -32.38601978689752769, 1523.530870145309564, 202.1199661129167851 ) ) ;
#16214=CARTESIAN_POINT ( 'NONE',  ( 34.68852446352948959, 1501.977400791986611, 218.2490599186006932 ) ) ;
#16216=AXIS2_PLACEMENT_3D ( 'NONE', #49751, #93925, #34031 ) ;
#16218=CARTESIAN_POINT ( 'NONE',  ( 32.38845791999500534, 1523.382868172864164, 216.1254071228445639 ) ) ;
#16230=EDGE_LOOP ( 'NONE', ( #32557, #17878, #25240, #22997 ) ) ;
#16232=CARTESIAN_POINT ( 'NONE',  ( 3.347801439373501609, 1523.456924617337791, 176.1543725842045660 ) ) ;
#16236=CARTESIAN_POINT ( 'NONE',  ( -17.84338787571901364, 1501.977400791986611, 237.8836641337663309 ) ) ;
#16246=ADVANCED_FACE ( 'NONE', ( #83992 ), #2062, .T. ) ;
#16253=ADVANCED_FACE ( 'NONE', ( #7291 ), #92943, .T. ) ;
#16265=AXIS2_PLACEMENT_3D ( 'NONE', #9131, #103166, #8017 ) ;
#16271=VERTEX_POINT ( 'NONE', #71097 ) ;
#16285=CARTESIAN_POINT ( 'NONE',  ( 0.4151546846821903003, 1512.187213306747481, 175.3106345060153046 ) ) ;
#16304=ORIENTED_EDGE ( 'NONE', *, *, #95175, .F. ) ;
#16309=EDGE_LOOP ( 'NONE', ( #44227, #44040, #96477, #71606 ) ) ;
#16323=DIRECTION ( 'NONE',  ( 0.000000000000000000, 1.000000000000000000, 0.000000000000000000 ) ) ;
#16326=AXIS2_PLACEMENT_3D ( 'NONE', #63114, #54146, #62562 ) ;
#16327=DIRECTION ( 'NONE',  ( -0.000000000000000000, -1.000000000000000000, -0.000000000000000000 ) ) ;
#16328=CARTESIAN_POINT ( 'NONE',  ( -21.78049460968791351, 1524.843416604514914, 233.5929001568862873 ) ) ;
#16331=( BOUNDED_SURFACE ( )  B_SPLINE_SURFACE ( 3, 2, ( 
 ( #106471, #99699, #48233 ),
 ( #63407, #99147, #80725 ),
 ( #89117, #46040, #98058 ),
 ( #13484, #97522, #38703 ) ),
 .UNSPECIFIED., .F., .F., .F. ) 
 B_SPLINE_SURFACE_WITH_KNOTS ( ( 4, 4 ),
 ( 3, 3 ),
 ( 0.000000000000000000, 0.0002960034161023847852 ),
 ( 0.000000000000000000, 1.000000000000000000 ),
 .UNSPECIFIED. ) 
 GEOMETRIC_REPRESENTATION_ITEM ( )  RATIONAL_B_SPLINE_SURFACE ( (
 ( 1.000000000000000000, 0.8070209408750061986, 1.000000000000000000),
 ( 1.000000000000000000, 0.8071723757218256523, 1.000000000000000000),
 ( 1.000000000000000000, 0.8072480346917807470, 1.000000000000000000),
 ( 1.000000000000000000, 0.8072480644198134492, 1.000000000000000000) ) ) 
 REPRESENTATION_ITEM ( '' )  SURFACE ( )  );
#16342=LINE ( 'NONE', #75739, #61050 ) ;
#16346=DIRECTION ( 'NONE',  ( 1.000000000000000000, -0.000000000000000000, 1.224646799147353207E-16 ) ) ;
#16351=CARTESIAN_POINT ( 'NONE',  ( -32.22536377336267321, 1523.621879633028584, 216.8351145222433445 ) ) ;
#16356=DIRECTION ( 'NONE',  ( 0.000000000000000000, 0.000000000000000000, -1.000000000000000000 ) ) ;
#16368=CARTESIAN_POINT ( 'NONE',  ( -30.95230591800407893, 1524.659802833171625, 196.4586593495655507 ) ) ;
#16375=CARTESIAN_POINT ( 'NONE',  ( -16.51111913633352302, 1525.159196711359755, 237.1918705644680756 ) ) ;
#16379=AXIS2_PLACEMENT_3D ( 'NONE', #100901, #90866, #73542 ) ;
#16392=DIRECTION ( 'NONE',  ( 0.000000000000000000, 0.000000000000000000, 1.000000000000000000 ) ) ;
#16399=CIRCLE ( 'NONE', #70111, 1.000000000000000888 ) ;
#16413=TOROIDAL_SURFACE ( 'NONE', #88004, 24.69926344187880929, 1.000000000000000000 ) ;
#16426=EDGE_CURVE ( 'NONE', #16271, #81031, #9497, .T. ) ;
#16448=CARTESIAN_POINT ( 'NONE',  ( 22.52214966617865599, 1524.244163922423013, 181.7424121231467211 ) ) ;
#16455=EDGE_CURVE ( 'NONE', #4488, #29284, #61059, .T. ) ;
#16463=VECTOR ( 'NONE', #61045, 1000.000000000000114 ) ;
#16465=ADVANCED_FACE ( 'NONE', ( #38014 ), #20935, .F. ) ;
#16480=CARTESIAN_POINT ( 'NONE',  ( -33.23421991949448540, 1522.906363951597314, 217.4142352873258517 ) ) ;
#16488=DIRECTION ( 'NONE',  ( 0.9983395709201744461, -0.05760296116452706672, 0.000000000000000000 ) ) ;
#16490=CARTESIAN_POINT ( 'NONE',  ( -20.92528168612626871, 1525.790286462515724, 184.9905026533984937 ) ) ;
#16492=DIRECTION ( 'NONE',  ( 0.000000000000000000, 1.000000000000000000, 0.000000000000000000 ) ) ;
#16514=DIRECTION ( 'NONE',  ( -0.6709778558543689764, 0.000000000000000000, 0.7414773880254701410 ) ) ;
#16522=CARTESIAN_POINT ( 'NONE',  ( -2.180465155517607556, 1524.667648926078982, 244.2585483383492715 ) ) ;
#16559=LINE ( 'NONE', #77614, #48068 ) ;
#16591=EDGE_CURVE ( 'NONE', #29937, #17762, #43985, .T. ) ;
#16596=EDGE_LOOP ( 'NONE', ( #89325, #52739, #2134, #62792 ) ) ;
#16601=EDGE_CURVE ( 'NONE', #97770, #61519, #1071, .T. ) ;
#16603=CARTESIAN_POINT ( 'NONE',  ( 2.389870119416070082, 1525.253996226948402, 176.1935146752628611 ) ) ;
#16608=DIRECTION ( 'NONE',  ( 0.000000000000000000, 0.000000000000000000, 1.000000000000000000 ) ) ;
#16609=CARTESIAN_POINT ( 'NONE',  ( -22.03465957474591619, 1522.382868172863937, 182.8300405912331144 ) ) ;
#16620=DIRECTION ( 'NONE',  ( 0.000000000000000000, 1.000000000000000000, 0.000000000000000000 ) ) ;
#16632=CARTESIAN_POINT ( 'NONE',  ( 31.23437356469434789, 1523.382868172864164, 195.3468678195113739 ) ) ;
#16639=ORIENTED_EDGE ( 'NONE', *, *, #12530, .F. ) ;
#16643=DIRECTION ( 'NONE',  ( 0.000000000000000000, 0.000000000000000000, 1.000000000000000000 ) ) ;
#16662=( BOUNDED_SURFACE ( )  B_SPLINE_SURFACE ( 3, 2, ( 
 ( #71711, #12290, #29107 ),
 ( #97408, #54878, #89003 ),
 ( #80616, #6102, #57088 ),
 ( #48126, #108006, #91758 ),
 ( #99596, #23450, #91212 ),
 ( #74439, #57645, #40257 ) ),
 .UNSPECIFIED., .F., .F., .T. ) 
 B_SPLINE_SURFACE_WITH_KNOTS ( ( 4, 2, 4 ),
 ( 3, 3 ),
 ( -3.642919299551294898E-17, 0.001312027981647369626, 0.002624055963294775681 ),
 ( 0.000000000000000000, 1.000000000000000000 ),
 .UNSPECIFIED. ) 
 GEOMETRIC_REPRESENTATION_ITEM ( )  RATIONAL_B_SPLINE_SURFACE ( (
 ( 1.000000000000000000, 0.9376006582765852304, 1.000000000000000000),
 ( 1.000000000000000000, 0.9569320108022569826, 1.000000000000000000),
 ( 1.000000000000000000, 0.9725743441618890373, 1.000000000000000000),
 ( 1.000000000000000000, 0.9942095667135610881, 1.000000000000000000),
 ( 1.000000000000000000, 1.000043666450710411, 1.000000000000000000),
 ( 1.000000000000000000, 1.000000000000000000, 1.000000000000000000) ) ) 
 REPRESENTATION_ITEM ( '' )  SURFACE ( )  );
#16677=VERTEX_POINT ( 'NONE', #62217 ) ;
#16698=EDGE_LOOP ( 'NONE', ( #91172, #53618, #74611, #81134 ) ) ;
#16710=VERTEX_POINT ( 'NONE', #1757 ) ;
#16714=ORIENTED_EDGE ( 'NONE', *, *, #51368, .T. ) ;
#16720=ADVANCED_FACE ( 'NONE', ( #79016 ), #104740, .F. ) ;
#16729=CARTESIAN_POINT ( 'NONE',  ( 2.136371660471265255, 1525.856064936157281, 241.3693953963658316 ) ) ;
#16756=DIRECTION ( 'NONE',  ( 0.9942586961433742543, 0.000000000000000000, -0.1070030146457445069 ) ) ;
#16765=EDGE_LOOP ( 'NONE', ( #8630, #25565, #93984, #90565, #81327 ) ) ;
#16774=DIRECTION ( 'NONE',  ( 0.000000000000000000, 1.000000000000000000, 0.000000000000000000 ) ) ;
#16784=CARTESIAN_POINT ( 'NONE',  ( -17.89234610336693265, 1523.611961620354123, 237.9279674222335359 ) ) ;
#16795=CARTESIAN_POINT ( 'NONE',  ( -4.097009089535903037, 1512.187213306747481, 201.1608118946569448 ) ) ;
#16802=CARTESIAN_POINT ( 'NONE',  ( -29.71163624023675354, 1526.333389947989644, 217.1029916164691826 ) ) ;
#16820=FACE_OUTER_BOUND ( 'NONE', #102866, .T. ) ;
#16836=CARTESIAN_POINT ( 'NONE',  ( 16.66231036550703593, 1523.604703353109699, 180.4882076302513099 ) ) ;
#16839=CIRCLE ( 'NONE', #79472, 2.000000000000001776 ) ;
#16849=ORIENTED_EDGE ( 'NONE', *, *, #105647, .F. ) ;
#16850=DIRECTION ( 'NONE',  ( 0.000000000000000000, 0.000000000000000000, -1.000000000000000000 ) ) ;
#16854=EDGE_CURVE ( 'NONE', #18098, #98801, #2854, .T. ) ;
#16869=ORIENTED_EDGE ( 'NONE', *, *, #91388, .F. ) ;
#16872=CARTESIAN_POINT ( 'NONE',  ( -21.59932114087497013, 1525.137906803776787, 233.5034269868583294 ) ) ;
#16890=ORIENTED_EDGE ( 'NONE', *, *, #45387, .F. ) ;
#16899=CARTESIAN_POINT ( 'NONE',  ( -33.93019615848938741, 1522.382868172863937, 220.5829544587966211 ) ) ;
#16912=CARTESIAN_POINT ( 'NONE',  ( -30.57064947821499246, 1523.844789899200805, 196.3873363930073879 ) ) ;
#16918=VECTOR ( 'NONE', #75220, 1000.000000000000000 ) ;
#16931=CARTESIAN_POINT ( 'NONE',  ( 17.59789087266998919, 1524.659148609499425, 180.6834670445046811 ) ) ;
#16937=CARTESIAN_POINT ( 'NONE',  ( -20.12564951288306858, 1511.187213306747708, 180.7149624981946658 ) ) ;
#16947=ORIENTED_EDGE ( 'NONE', *, *, #61279, .T. ) ;
#16949=CARTESIAN_POINT ( 'NONE',  ( 21.28823305372374719, 1525.253996226948630, 183.8869967656500819 ) ) ;
#16950=ORIENTED_EDGE ( 'NONE', *, *, #6907, .T. ) ;
#16953=DIRECTION ( 'NONE',  ( -0.9125304618754024322, 0.000000000000000000, -0.4090087482554191078 ) ) ;
#16954=CYLINDRICAL_SURFACE ( 'NONE', #60613, 4.000000000000001776 ) ;
#16970=ORIENTED_EDGE ( 'NONE', *, *, #13827, .T. ) ;
#16977=DIRECTION ( 'NONE',  ( 0.000000000000000000, 0.000000000000000000, 1.000000000000000000 ) ) ;
#16980=ORIENTED_EDGE ( 'NONE', *, *, #9132, .F. ) ;
#16984=DIRECTION ( 'NONE',  ( 0.000000000000000000, 0.000000000000000000, 1.000000000000000000 ) ) ;
#16988=ORIENTED_EDGE ( 'NONE', *, *, #79504, .T. ) ;
#16992=DIRECTION ( 'NONE',  ( 0.9942586961433742543, -0.000000000000000000, -0.1070030146457445069 ) ) ;
#16993=CARTESIAN_POINT ( 'NONE',  ( 21.41758936356361076, 1524.330813522192102, 184.2067724269726909 ) ) ;
#16996=DIRECTION ( 'NONE',  ( 0.000000000000000000, 0.000000000000000000, 1.000000000000000000 ) ) ;
#17000=AXIS2_PLACEMENT_3D ( 'NONE', #57189, #16774, #50977 ) ;
#17002=CARTESIAN_POINT ( 'NONE',  ( 30.11857922865945270, 1525.055427061254477, 221.6904370749649047 ) ) ;
#17009=CYLINDRICAL_SURFACE ( 'NONE', #2142, 0.9999999999999983347 ) ;
#17032=CARTESIAN_POINT ( 'NONE',  ( -21.39312961732860785, 1524.775785348137561, 184.2561049718586048 ) ) ;
#17035=VERTEX_POINT ( 'NONE', #65383 ) ;
#17056=EDGE_LOOP ( 'NONE', ( #15773, #24158, #84611, #26292 ) ) ;
#17059=DIRECTION ( 'NONE',  ( 0.000000000000000000, 1.000000000000000000, 0.000000000000000000 ) ) ;
#17065=CARTESIAN_POINT ( 'NONE',  ( -0.6235920161070117596, 1525.878013734321485, 242.9475333194527877 ) ) ;
#17073=ORIENTED_EDGE ( 'NONE', *, *, #10300, .T. ) ;
#17077=EDGE_CURVE ( 'NONE', #100609, #38471, #79802, .T. ) ;
#17093=CARTESIAN_POINT ( 'NONE',  ( 2.469101154908970308, 1524.816548299036640, 242.3848636420295293 ) ) ;
#17096=ORIENTED_EDGE ( 'NONE', *, *, #74781, .F. ) ;
#17111=( BOUNDED_SURFACE ( )  B_SPLINE_SURFACE ( 3, 2, ( 
 ( #29985, #106694, #12089 ),
 ( #79864, #56311, #90444 ),
 ( #11551, #3174, #88806 ),
 ( #105620, #39507, #63099 ) ),
 .UNSPECIFIED., .F., .F., .F. ) 
 B_SPLINE_SURFACE_WITH_KNOTS ( ( 4, 4 ),
 ( 3, 3 ),
 ( 0.000000000000000000, 0.0002960034161023848936 ),
 ( 0.000000000000000000, 1.000000000000000000 ),
 .UNSPECIFIED. ) 
 GEOMETRIC_REPRESENTATION_ITEM ( )  RATIONAL_B_SPLINE_SURFACE ( (
 ( 1.000000000000000000, 0.8072480644198120059, 1.000000000000000000),
 ( 1.000000000000000000, 0.8072480346917830785, 1.000000000000000000),
 ( 1.000000000000000000, 0.8071723757218312034, 1.000000000000000000),
 ( 1.000000000000000000, 0.8070209408750057545, 1.000000000000000000) ) ) 
 REPRESENTATION_ITEM ( '' )  SURFACE ( )  );
#17114=CARTESIAN_POINT ( 'NONE',  ( 31.18497486287775899, 1524.152349020271004, 196.3673245421346394 ) ) ;
#17137=CARTESIAN_POINT ( 'NONE',  ( -16.48227147120495317, 1525.651286436459031, 236.6829015109164516 ) ) ;
#17148=VERTEX_POINT ( 'NONE', #51878 ) ;
#17151=VECTOR ( 'NONE', #28029, 1000.000000000000000 ) ;
#17153=CARTESIAN_POINT ( 'NONE',  ( 2.693001348315085863, 1524.059663615499858, 176.1570368348570241 ) ) ;
#17172=CARTESIAN_POINT ( 'NONE',  ( 28.44964981547635219, 1526.382868172864164, 219.8796466721251477 ) ) ;
#17179=CARTESIAN_POINT ( 'NONE',  ( -3.347801439296141268, 1518.913060387330006, 242.0893193391992497 ) ) ;
#17195=CARTESIAN_POINT ( 'NONE',  ( -2.038847259689231084, 1522.382868172863937, 244.9330574173806951 ) ) ;
#17196=CARTESIAN_POINT ( 'NONE',  ( 22.75273496409577945, 1523.382868172864164, 183.6728937936772184 ) ) ;
#17205=ORIENTED_EDGE ( 'NONE', *, *, #44367, .T. ) ;
#17210=CARTESIAN_POINT ( 'NONE',  ( 0.000000000000000000, 1523.409940573003951, 209.1218459616979999 ) ) ;
#17231=ADVANCED_FACE ( 'NONE', ( #79839 ), #51178, .T. ) ;
#17267=DIRECTION ( 'NONE',  ( 1.387778780781444413E-14, 0.000000000000000000, 1.000000000000000000 ) ) ;
#17278=CARTESIAN_POINT ( 'NONE',  ( 30.83422926911982032, 1524.871836253796118, 196.5181389497718385 ) ) ;
#17284=ORIENTED_EDGE ( 'NONE', *, *, #35693, .F. ) ;
#17307=CIRCLE ( 'NONE', #6563, 1.999999999999995559 ) ;
#17315=( BOUNDED_SURFACE ( )  B_SPLINE_SURFACE ( 3, 2, ( 
 ( #78000, #78559, #44978 ),
 ( #52818, #25918, #36550 ),
 ( #103757, #8577, #19167 ),
 ( #102618, #216, #61782 ),
 ( #76909, #86396, #27058 ),
 ( #62337, #1875, #28147 ),
 ( #42747, #69634, #51151 ),
 ( #17509, #1306, #35446 ),
 ( #10808, #68519, #16949 ),
 ( #95906, #44417, #61244 ),
 ( #9685, #53373, #60116 ),
 ( #94234, #34341, #18618 ),
 ( #86949, #10241, #77458 ),
 ( #36009, #70201, #26480 ) ),
 .UNSPECIFIED., .F., .F., .F. ) 
 B_SPLINE_SURFACE_WITH_KNOTS ( ( 4, 2, 2, 2, 2, 2, 4 ),
 ( 3, 3 ),
 ( 2.252972114424878214E-16, 0.0009440840677147236759, 0.001416126101571972811, 0.001888168135429222055, 0.002360210169286471298, 0.002832252203143720542, 0.003776336270858219029 ),
 ( 0.000000000000000000, 1.000000000000000000 ),
 .UNSPECIFIED. ) 
 GEOMETRIC_REPRESENTATION_ITEM ( )  RATIONAL_B_SPLINE_SURFACE ( (
 ( 1.000000000000000000, 0.8070209408749953184, 1.000000000000000000),
 ( 1.000000000000000000, 0.8215603905291239961, 1.000000000000000000),
 ( 1.000000000000000000, 0.8340988699051420374, 1.000000000000000000),
 ( 1.000000000000000000, 0.8516751610463629829, 1.000000000000000000),
 ( 1.000000000000000000, 0.8573697395147750200, 1.000000000000000000),
 ( 1.000000000000000000, 0.8683586635668578690, 1.000000000000000000),
 ( 1.000000000000000000, 0.8736518481705473071, 1.000000000000000000),
 ( 1.000000000000000000, 0.8840377753033259456, 1.000000000000000000),
 ( 1.000000000000000000, 0.8891294171308693484, 1.000000000000000000),
 ( 1.000000000000000000, 0.8992456600572363845, 1.000000000000000000),
 ( 1.000000000000000000, 0.9042785869256293463, 1.000000000000000000),
 ( 1.000000000000000000, 0.9189749222831727904, 1.000000000000000000),
 ( 1.000000000000000000, 0.9283978182353632702, 1.000000000000000000),
 ( 1.000000000000000000, 0.9376006582765943342, 1.000000000000000000) ) ) 
 REPRESENTATION_ITEM ( '' )  SURFACE ( )  );
#17323=CARTESIAN_POINT ( 'NONE',  ( -32.00451504911058720, 1524.843416604514459, 216.1170911566689767 ) ) ;
#17375=CARTESIAN_POINT ( 'NONE',  ( 21.95768443299136052, 1524.412455883367329, 233.6991302426335437 ) ) ;
#17388=ORIENTED_EDGE ( 'NONE', *, *, #51368, .F. ) ;
#17389=AXIS2_PLACEMENT_3D ( 'NONE', #99389, #98299, #22667 ) ;
#17396=VECTOR ( 'NONE', #8265, 1000.000000000000000 ) ;
#17426=CARTESIAN_POINT ( 'NONE',  ( -17.06401309437357483, 1526.329757971584741, 181.0652997614164974 ) ) ;
#17435=LINE ( 'NONE', #85770, #7457 ) ;
#17451=CARTESIAN_POINT ( 'NONE',  ( 32.38601978689747796, 1523.530870145309109, 216.1237258104796410 ) ) ;
#17464=CARTESIAN_POINT ( 'NONE',  ( 21.54905603439488004, 1524.816548299036867, 234.5808913040066841 ) ) ;
#17473=VECTOR ( 'NONE', #34737, 1000.000000000000000 ) ;
#17478=CIRCLE ( 'NONE', #80091, 33.13701971169416538 ) ;
#17480=DIRECTION ( 'NONE',  ( -0.7414773880254664773, 0.000000000000000000, 0.6709778558543730842 ) ) ;
#17481=ADVANCED_FACE ( 'NONE', ( #1919 ), #79172, .T. ) ;
#17487=CARTESIAN_POINT ( 'NONE',  ( 16.64711273906109668, 1523.843263703802904, 180.4998296529583683 ) ) ;
#17497=CIRCLE ( 'NONE', #110487, 2.000000000000001776 ) ;
#17509=CARTESIAN_POINT ( 'NONE',  ( 21.66432897272961000, 1525.042412244735260, 184.7096312766485084 ) ) ;
#17561=AXIS2_PLACEMENT_3D ( 'NONE', #79727, #47215, #1926 ) ;
#17566=VECTOR ( 'NONE', #28000, 1000.000000000000000 ) ;
#17575=CARTESIAN_POINT ( 'NONE',  ( 3.448830483803564828, 1518.913060387330006, 243.0842028158767789 ) ) ;
#17595=CARTESIAN_POINT ( 'NONE',  ( 19.34601893677221440, 1526.333389947990327, 185.2009018889368406 ) ) ;
#17596=DIRECTION ( 'NONE',  ( -0.5877852522924629231, 0.000000000000000000, 0.8090169943749548898 ) ) ;
#17598=CARTESIAN_POINT ( 'NONE',  ( 19.01764264267215410, 1526.373507135059072, 185.3901233886903128 ) ) ;
#17640=( BOUNDED_CURVE ( )  B_SPLINE_CURVE ( 3, ( #82791, #22302, #56505, #12827 ),
 .UNSPECIFIED., .F., .F. ) 
 B_SPLINE_CURVE_WITH_KNOTS ( ( 4, 4 ),
 ( 4.712388980384695003, 6.283185307179586232 ),
 .UNSPECIFIED. ) 
 CURVE ( )  GEOMETRIC_REPRESENTATION_ITEM ( )  RATIONAL_B_SPLINE_CURVE ( ( 1.000000000000000000, 0.8047378541243662697, 0.8047378541243662697, 1.000000000000000000 ) ) 
 REPRESENTATION_ITEM ( '' )  );
#17642=CARTESIAN_POINT ( 'NONE',  ( -32.00465973459075286, 1524.843178112495480, 202.1266218387728770 ) ) ;
#17655=ORIENTED_EDGE ( 'NONE', *, *, #31489, .T. ) ;
#17663=DIRECTION ( 'NONE',  ( -0.8672669759446636206, 0.000000000000000000, 0.4978433412588729734 ) ) ;
#17672=CARTESIAN_POINT ( 'NONE',  ( 32.28466283162156714, 1512.187213306747481, 219.1752493337713190 ) ) ;
#17682=ORIENTED_EDGE ( 'NONE', *, *, #110148, .F. ) ;
#17686=VERTEX_POINT ( 'NONE', #73522 ) ;
#17705=CARTESIAN_POINT ( 'NONE',  ( 2.472529913803023227, 1523.678648413191695, 242.8674788698241400 ) ) ;
#17711=CARTESIAN_POINT ( 'NONE',  ( 2.410642264446942296, 1525.163527997520532, 176.1170057922971353 ) ) ;
#17747=CARTESIAN_POINT ( 'NONE',  ( 20.20959865099491992, 1511.187213306747708, 236.2316688286738611 ) ) ;
#17762=VERTEX_POINT ( 'NONE', #107655 ) ;
#17782=CIRCLE ( 'NONE', #55398, 1.000000000000000888 ) ;
#17784=VERTEX_POINT ( 'NONE', #56708 ) ;
#17793=CARTESIAN_POINT ( 'NONE',  ( -2.708826876440360909, 1524.477587234266366, 176.2952420485788423 ) ) ;
#17836=CARTESIAN_POINT ( 'NONE',  ( -16.66231036550740541, 1523.604703353109699, 180.4882076302515372 ) ) ;
#17853=EDGE_CURVE ( 'NONE', #31153, #83342, #35221, .T. ) ;
#17860=CIRCLE ( 'NONE', #64433, 1.000000000000000000 ) ;
#17862=CARTESIAN_POINT ( 'NONE',  ( -2.596261494520225366, 1525.907212628473644, 177.4701144822246874 ) ) ;
#17878=ORIENTED_EDGE ( 'NONE', *, *, #94503, .T. ) ;
#17882=DIRECTION ( 'NONE',  ( 0.000000000000000000, 1.000000000000000000, 0.000000000000000000 ) ) ;
#17890=EDGE_CURVE ( 'NONE', #108700, #95777, #53878, .T. ) ;
#17895=FACE_OUTER_BOUND ( 'NONE', #30668, .T. ) ;
#17912=CARTESIAN_POINT ( 'NONE',  ( -22.75273496409615603, 1512.187213306747481, 183.6728937936775310 ) ) ;
#17924=ORIENTED_EDGE ( 'NONE', *, *, #83873, .T. ) ;
#17935=CIRCLE ( 'NONE', #32274, 1.999999999999990452 ) ;
#17954=CIRCLE ( 'NONE', #23326, 1.000000000000003553 ) ;
#17959=( BOUNDED_SURFACE ( )  B_SPLINE_SURFACE ( 3, 2, ( 
 ( #77787, #61011, #86733 ),
 ( #10023, #68307, #16729 ),
 ( #50392, #102415, #44193 ),
 ( #78336, #85060, #76127 ),
 ( #110268, #42515, #33545 ),
 ( #67743, #101852, #25145 ),
 ( #95689, #62678, #96800 ),
 ( #35783, #104080, #62115 ),
 ( #79989, #3861, #87289 ),
 ( #105756, #11146, #88391 ),
 ( #63227, #97332, #3309 ),
 ( #53151, #54801, #69967 ),
 ( #37439, #11679, #71072 ),
 ( #37989, #29041, #10584 ) ),
 .UNSPECIFIED., .F., .F., .T. ) 
 B_SPLINE_SURFACE_WITH_KNOTS ( ( 4, 2, 2, 2, 2, 2, 4 ),
 ( 3, 3 ),
 ( 3.503057219300664826E-16, 0.0009443072508239318524, 0.001416460876235722463, 0.001888614501647513291, 0.002360768127059304118, 0.002832921752471094512, 0.003777229003294676167 ),
 ( 0.000000000000000000, 1.000000000000000000 ),
 .UNSPECIFIED. ) 
 GEOMETRIC_REPRESENTATION_ITEM ( )  RATIONAL_B_SPLINE_SURFACE ( (
 ( 1.000000000000000000, 0.9376006582765973318, 1.000000000000000000),
 ( 1.000000000000000000, 0.9283977714730341502, 1.000000000000000000),
 ( 1.000000000000000000, 0.9189750060488427463, 1.000000000000000000),
 ( 1.000000000000000000, 0.9042792056123200028, 1.000000000000000000),
 ( 1.000000000000000000, 0.8992469033844596726, 1.000000000000000000),
 ( 1.000000000000000000, 0.8891280264680869738, 1.000000000000000000),
 ( 1.000000000000000000, 0.8840337471675274728, 1.000000000000000000),
 ( 1.000000000000000000, 0.8736395124163596204, 1.000000000000000000),
 ( 1.000000000000000000, 0.8683406746556232569, 1.000000000000000000),
 ( 1.000000000000000000, 0.8573361860704289406, 1.000000000000000000),
 ( 1.000000000000000000, 0.8516508399493524228, 1.000000000000000000),
 ( 1.000000000000000000, 0.8340914917071279300, 1.000000000000000000),
 ( 1.000000000000000000, 0.8215597275858022019, 1.000000000000000000),
 ( 1.000000000000000000, 0.8070209408750096403, 1.000000000000000000) ) ) 
 REPRESENTATION_ITEM ( '' )  SURFACE ( )  );
#17985=CARTESIAN_POINT ( 'NONE',  ( 31.34137657934009979, 1512.187213306747481, 196.3411265156547358 ) ) ;
#18007=CYLINDRICAL_SURFACE ( 'NONE', #96758, 1.000000000000000888 ) ;
#18018=EDGE_CURVE ( 'NONE', #69179, #16271, #12341, .T. ) ;
#18021=DIRECTION ( 'NONE',  ( 0.000000000000000000, 0.000000000000000000, 1.000000000000000000 ) ) ;
#18044=DIRECTION ( 'NONE',  ( 0.9970203751124364633, -0.07713865185920967815, 0.000000000000000000 ) ) ;
#18045=CARTESIAN_POINT ( 'NONE',  ( -16.50400130224731754, 1525.907212628473644, 236.2546788475584094 ) ) ;
#18055=CARTESIAN_POINT ( 'NONE',  ( 16.48227147120181257, 1525.651286436459941, 181.5607904124787808 ) ) ;
#18078=VERTEX_POINT ( 'NONE', #37560 ) ;
#18082=CARTESIAN_POINT ( 'NONE',  ( 0.000000000000000000, 1518.913060387330006, 185.4225825198192013 ) ) ;
#18085=CIRCLE ( 'NONE', #39520, 2.000000000000001776 ) ;
#18098=VERTEX_POINT ( 'NONE', #3980 ) ;
#18111=ORIENTED_EDGE ( 'NONE', *, *, #101368, .F. ) ;
#18125=CARTESIAN_POINT ( 'NONE',  ( 21.38516915557947584, 1522.906561336852974, 180.3939891059719969 ) ) ;
#18133=AXIS2_PLACEMENT_3D ( 'NONE', #108180, #31471, #65652 ) ;
#18134=CARTESIAN_POINT ( 'NONE',  ( 30.25946001110534311, 1524.776010967693537, 221.7839220010320105 ) ) ;
#18136=ORIENTED_EDGE ( 'NONE', *, *, #54811, .T. ) ;
#18170=CARTESIAN_POINT ( 'NONE',  ( 30.31052258194586102, 1523.604703353109699, 195.7506062427368079 ) ) ;
#18202=ORIENTED_EDGE ( 'NONE', *, *, #78172, .T. ) ;
#18220=EDGE_LOOP ( 'NONE', ( #110606, #22465, #89670, #101064, #67710 ) ) ;
#18222=CIRCLE ( 'NONE', #7282, 1.000000000000000888 ) ;
#18223=FACE_OUTER_BOUND ( 'NONE', #80654, .T. ) ;
#18249=CARTESIAN_POINT ( 'NONE',  ( -30.00400320040627378, 1524.843178112495707, 222.2744577634231007 ) ) ;
#18258=B_SPLINE_CURVE_WITH_KNOTS ( 'NONE', 3,
 ( #28874, #37276, #64705, #22083, #90410, #71470, #13690, #47875, #105590, #46252 ),
 .UNSPECIFIED., .F., .F.,
 ( 4, 2, 2, 2, 4 ),
 ( 1.301042606982605321E-18, 0.0007406479101618186189, 0.001481295820323635937, 0.002221943730485453471, 0.002962591640647270572 ),
 .UNSPECIFIED. ) ;
#18267=DIRECTION ( 'NONE',  ( -0.000000000000000000, -1.000000000000000000, -0.000000000000000000 ) ) ;
#18281=CARTESIAN_POINT ( 'NONE',  ( -29.74902317390499107, 1525.343710797494850, 196.2390521661037894 ) ) ;
#18291=CARTESIAN_POINT ( 'NONE',  ( 0.6235920161070115375, 1525.878013734321257, 242.9475333194528446 ) ) ;
#18294=LINE ( 'NONE', #8792, #3281 ) ;
#18299=FACE_OUTER_BOUND ( 'NONE', #67158, .T. ) ;
#18300=FACE_OUTER_BOUND ( 'NONE', #98414, .T. ) ;
#18313=ORIENTED_EDGE ( 'NONE', *, *, #21343, .T. ) ;
#18317=DIRECTION ( 'NONE',  ( -1.000000000000000000, 0.000000000000000000, 0.000000000000000000 ) ) ;
#18330=DIRECTION ( 'NONE',  ( 0.9786619618251657382, 0.000000000000000000, 0.2054769195713180563 ) ) ;
#18348=EDGE_LOOP ( 'NONE', ( #19030, #27842, #34218, #70335 ) ) ;
#18351=CARTESIAN_POINT ( 'NONE',  ( 1.191524307911311586, 1526.382868172863937, 179.0083900503167911 ) ) ;
#18400=EDGE_LOOP ( 'NONE', ( #43331, #38803, #34623, #69213 ) ) ;
#18401=DIRECTION ( 'NONE',  ( -0.9510565162951518658, 0.000000000000000000, 0.3090169943749526138 ) ) ;
#18408=CARTESIAN_POINT ( 'NONE',  ( -28.27139721233055170, 1526.382868172863937, 198.6830693683576214 ) ) ;
#18416=DIRECTION ( 'NONE',  ( 0.000000000000000000, 1.000000000000000000, 0.000000000000000000 ) ) ;
#18434=ORIENTED_EDGE ( 'NONE', *, *, #98027, .T. ) ;
#18441=B_SPLINE_CURVE_WITH_KNOTS ( 'NONE', 3,
 ( #54158, #3755, #19963, #98326, #12676, #38418 ),
 .UNSPECIFIED., .F., .F.,
 ( 4, 2, 4 ),
 ( -1.131363979615304141E-05, 0.001067788114096033690, 0.002146889867988220277 ),
 .UNSPECIFIED. ) ;
#18464=CARTESIAN_POINT ( 'NONE',  ( 0.000000000000000000, 1523.382868172864164, 209.1218459616979999 ) ) ;
#18470=CARTESIAN_POINT ( 'NONE',  ( -2.225543501807631053, 1525.712835404586031, 176.6707008850455622 ) ) ;
#18474=EDGE_LOOP ( 'NONE', ( #59799, #42744, #70521, #56888, #4222, #94232, #96298, #99219 ) ) ;
#18493=EDGE_LOOP ( 'NONE', ( #8353, #56267, #23718 ) ) ;
#18497=EDGE_LOOP ( 'NONE', ( #59028, #23226, #84925 ) ) ;
#18515=DIRECTION ( 'NONE',  ( 0.4090087482554164988, -1.225281874271768203E-16, -0.9125304618754035424 ) ) ;
#18516=EDGE_LOOP ( 'NONE', ( #31577, #110495, #2934, #76228 ) ) ;
#18541=DIRECTION ( 'NONE',  ( -0.000000000000000000, -1.000000000000000000, -0.000000000000000000 ) ) ;
#18577=CARTESIAN_POINT ( 'NONE',  ( 16.66936639845630097, 1523.382868172864164, 180.4828114240739296 ) ) ;
#18585=DIRECTION ( 'NONE',  ( 0.000000000000000000, 0.000000000000000000, 1.000000000000000000 ) ) ;
#18606=AXIS2_PLACEMENT_3D ( 'NONE', #92322, #99611, #75003 ) ;
#18618=CARTESIAN_POINT ( 'NONE',  ( 20.85167258422537984, 1525.730671215511848, 184.1901402302743236 ) ) ;
#18628=ADVANCED_FACE ( 'NONE', ( #29309 ), #63185, .F. ) ;
#18638=ORIENTED_EDGE ( 'NONE', *, *, #19256, .F. ) ;
#18640=DIRECTION ( 'NONE',  ( 0.000000000000000000, 0.000000000000000000, 1.000000000000000000 ) ) ;
#18642=ORIENTED_EDGE ( 'NONE', *, *, #68384, .T. ) ;
#18650=ADVANCED_FACE ( 'NONE', ( #14704 ), #97480, .F. ) ;
#18668=FACE_OUTER_BOUND ( 'NONE', #39046, .T. ) ;
#18669=CARTESIAN_POINT ( 'NONE',  ( 34.18677586421189574, 1501.977400791986611, 219.7932833225211766 ) ) ;
#18680=CARTESIAN_POINT ( 'NONE',  ( 30.24977872777046883, 1524.075132568165373, 222.4742436132389685 ) ) ;
#18704=CARTESIAN_POINT ( 'NONE',  ( -19.36857742237540236, 1526.335487865669393, 232.9229765951374986 ) ) ;
#18710=CARTESIAN_POINT ( 'NONE',  ( -21.83550407203938448, 1523.678648413191922, 183.2743720722711203 ) ) ;
#18711=CARTESIAN_POINT ( 'NONE',  ( -19.53786426058999481, 1501.977400791986611, 236.7197124308268030 ) ) ;
#18719=CARTESIAN_POINT ( 'NONE',  ( -31.69312280309501872, 1525.713797967457140, 196.3032712708389909 ) ) ;
#18724=VECTOR ( 'NONE', #93539, 1000.000000000000227 ) ;
#18726=ORIENTED_EDGE ( 'NONE', *, *, #79451, .T. ) ;
#18729=CARTESIAN_POINT ( 'NONE',  ( 30.31940284292408450, 1523.456872492435195, 195.7503880523414352 ) ) ;
#18734=AXIS2_PLACEMENT_3D ( 'NONE', #84209, #102108, #34369 ) ;
#18755=CARTESIAN_POINT ( 'NONE',  ( -31.62137330308219063, 1525.231909165050865, 201.5806583896697646 ) ) ;
#18763=EDGE_CURVE ( 'NONE', #33528, #5040, #81719, .T. ) ;
#18823=EDGE_LOOP ( 'NONE', ( #69631, #90970, #5181, #102016, #20560 ) ) ;
#18845=CARTESIAN_POINT ( 'NONE',  ( 29.33431687954583111, 1526.382868172863937, 217.1433072912829800 ) ) ;
#18847=CARTESIAN_POINT ( 'NONE',  ( 29.55269881708361268, 1525.821544997590536, 221.1141083160992764 ) ) ;
#18852=AXIS2_PLACEMENT_3D ( 'NONE', #17747, #18864, #86091 ) ;
#18854=CARTESIAN_POINT ( 'NONE',  ( -31.44837959398599736, 1511.187213306747708, 197.3353852117985525 ) ) ;
#18862=ORIENTED_EDGE ( 'NONE', *, *, #5027, .F. ) ;
#18864=DIRECTION ( 'NONE',  ( -0.000000000000000000, -1.000000000000000000, -0.000000000000000000 ) ) ;
#18871=DIRECTION ( 'NONE',  ( 0.000000000000000000, 0.000000000000000000, -1.000000000000000000 ) ) ;
#18893=TOROIDAL_SURFACE ( 'NONE', #83252, 2.000000000000000000, 1.000000000000000000 ) ;
#18908=DIRECTION ( 'NONE',  ( 0.4978433412588676998, 0.000000000000000000, -0.8672669759446663962 ) ) ;
#18918=DIRECTION ( 'NONE',  ( 0.000000000000000000, 0.000000000000000000, 1.000000000000000000 ) ) ;
#18935=ADVANCED_FACE ( 'NONE', ( #75050 ), #15102, .F. ) ;
#18937=CARTESIAN_POINT ( 'NONE',  ( 31.43069643840505734, 1526.748660780343471, 216.5579808171732736 ) ) ;
#18958=CARTESIAN_POINT ( 'NONE',  ( 22.41686883764669602, 1524.667648926078300, 236.2663900491572235 ) ) ;
#18970=CARTESIAN_POINT ( 'NONE',  ( 30.90487439922556945, 1525.907212628473644, 201.8101144455177689 ) ) ;
#18972=DIRECTION ( 'NONE',  ( 0.000000000000000000, 1.000000000000000000, 0.000000000000000000 ) ) ;
#19008=ORIENTED_EDGE ( 'NONE', *, *, #14869, .F. ) ;
#19015=CARTESIAN_POINT ( 'NONE',  ( 31.81424859195960408, 1524.964230758883104, 201.5864201284566093 ) ) ;
#19027=ORIENTED_EDGE ( 'NONE', *, *, #55436, .T. ) ;
#19029=DIRECTION ( 'NONE',  ( 1.000000000000000000, 0.000000000000000000, -0.000000000000000000 ) ) ;
#19030=ORIENTED_EDGE ( 'NONE', *, *, #19541, .T. ) ;
#19064=ORIENTED_EDGE ( 'NONE', *, *, #51675, .T. ) ;
#19068=EDGE_LOOP ( 'NONE', ( #21012, #11244, #59704 ) ) ;
#19090=CARTESIAN_POINT ( 'NONE',  ( -18.19590854886883236, 1522.644714754858114, 180.0410247165304156 ) ) ;
#19092=DIRECTION ( 'NONE',  ( -0.1070030146457508768, 0.000000000000000000, -0.9942586961433735881 ) ) ;
#19094=ORIENTED_EDGE ( 'NONE', *, *, #54225, .F. ) ;
#19110=CARTESIAN_POINT ( 'NONE',  ( -33.05665451062209570, 1523.390106123591067, 217.3123061710364254 ) ) ;
#19121=EDGE_CURVE ( 'NONE', #71944, #37474, #3321, .T. ) ;
#19122=LINE ( 'NONE', #63394, #56925 ) ;
#19125=ORIENTED_EDGE ( 'NONE', *, *, #96302, .T. ) ;
#19129=CARTESIAN_POINT ( 'NONE',  ( 21.38516915557987375, 1524.726013923371056, 237.8497028174237755 ) ) ;
#19138=CARTESIAN_POINT ( 'NONE',  ( -19.53786426058999481, 1512.187213306747481, 237.7197124308268030 ) ) ;
#19152=CARTESIAN_POINT ( 'NONE',  ( 0.000000000000000000, 1523.382868172864164, 209.1218459616979999 ) ) ;
#19160=PRESENTATION_STYLE_ASSIGNMENT (( #85841 ) ) ;
#19165=ORIENTED_EDGE ( 'NONE', *, *, #19541, .F. ) ;
#19167=CARTESIAN_POINT ( 'NONE',  ( 21.75647715750188738, 1524.201816949777594, 183.4206492032029416 ) ) ;
#19181=LINE ( 'NONE', #1319, #73331 ) ;
#19186=ORIENTED_EDGE ( 'NONE', *, *, #59143, .T. ) ;
#19188=ORIENTED_EDGE ( 'NONE', *, *, #63496, .F. ) ;
#19211=DIRECTION ( 'NONE',  ( 0.8090169943749465631, 0.000000000000000000, -0.5877852522924742473 ) ) ;
#19222=CARTESIAN_POINT ( 'NONE',  ( 30.87183381296008022, 1524.816846803860926, 221.7488379675505143 ) ) ;
#19228=CARTESIAN_POINT ( 'NONE',  ( -17.26793975759867550, 1525.730671948510917, 236.6572836587323536 ) ) ;
#19254=CARTESIAN_POINT ( 'NONE',  ( 31.34137657934008558, 1501.977400791986611, 196.3411265156547358 ) ) ;
#19256=EDGE_CURVE ( 'NONE', #24484, #30213, #63766, .T. ) ;
#19257=CARTESIAN_POINT ( 'NONE',  ( -31.41104781486828301, 1512.187213306747481, 202.3296363711539527 ) ) ;
#19260=FACE_OUTER_BOUND ( 'NONE', #51168, .T. ) ;
#19308=CARTESIAN_POINT ( 'NONE',  ( -30.90487439922554103, 1525.907212628473644, 201.8101144455182521 ) ) ;
#19317=VERTEX_POINT ( 'NONE', #110152 ) ;
#19328=ADVANCED_FACE ( 'NONE', ( #33423 ), #33039, .T. ) ;
#19332=CIRCLE ( 'NONE', #96247, 1.000000000000000888 ) ;
#19333=EDGE_CURVE ( 'NONE', #7367, #85956, #99018, .T. ) ;
#19349=VECTOR ( 'NONE', #19457, 1000.000000000000000 ) ;
#19360=ORIENTED_EDGE ( 'NONE', *, *, #26884, .T. ) ;
#19366=EDGE_CURVE ( 'NONE', #38471, #38998, #49624, .T. ) ;
#19383=DIRECTION ( 'NONE',  ( -0.1070030146457249254, 0.000000000000000000, 0.9942586961433763637 ) ) ;
#19402=CARTESIAN_POINT ( 'NONE',  ( -2.444956619880277682, 1524.972613296788722, 242.2723289509666529 ) ) ;
#19404=CARTESIAN_POINT ( 'NONE',  ( 28.27139721233034564, 1526.382868172864164, 219.5606225550385204 ) ) ;
#19425=DIRECTION ( 'NONE',  ( -0.7882878497005411100, 0.000000000000000000, 0.6153066438894488899 ) ) ;
#19457=DIRECTION ( 'NONE',  ( 0.4090087482554252696, 0.000000000000000000, -0.9125304618753996566 ) ) ;
#19466=AXIS2_PLACEMENT_3D ( 'NONE', #42241, #85892, #59056 ) ;
#19472=FACE_OUTER_BOUND ( 'NONE', #64725, .T. ) ;
#19484=ORIENTED_EDGE ( 'NONE', *, *, #40616, .F. ) ;
#19490=AXIS2_PLACEMENT_3D ( 'NONE', #75178, #23647, #91417 ) ;
#19508=DIRECTION ( 'NONE',  ( 0.000000000000000000, 1.000000000000000000, 0.000000000000000000 ) ) ;
#19518=CARTESIAN_POINT ( 'NONE',  ( 22.03465957474552539, 1501.977400791986611, 182.8300405912328301 ) ) ;
#19519=CARTESIAN_POINT ( 'NONE',  ( 22.03465957474572079, 1522.382868172863937, 235.4136513321629991 ) ) ;
#19539=AXIS2_PLACEMENT_3D ( 'NONE', #45459, #11291, #105899 ) ;
#19541=EDGE_CURVE ( 'NONE', #79144, #100188, #35297, .T. ) ;
#19555=CARTESIAN_POINT ( 'NONE',  ( -31.97146249857350853, 1524.678872986481565, 216.6705896045354791 ) ) ;
#19558=ORIENTED_EDGE ( 'NONE', *, *, #27442, .T. ) ;
#19576=ORIENTED_EDGE ( 'NONE', *, *, #58040, .F. ) ;
#19578=ADVANCED_FACE ( 'NONE', ( #1381 ), #31775, .T. ) ;
#19584=CARTESIAN_POINT ( 'NONE',  ( 32.70814417905861404, 1524.201816949777822, 201.1172774233197913 ) ) ;
#19588=DIRECTION ( 'NONE',  ( 0.07713599384728243857, -0.9969860201949397593, -0.008301444997534272036 ) ) ;
#19604=VECTOR ( 'NONE', #9375, 1000.000000000000000 ) ;
#19610=ORIENTED_EDGE ( 'NONE', *, *, #48922, .F. ) ;
#19653=ORIENTED_EDGE ( 'NONE', *, *, #34105, .F. ) ;
#19655=AXIS2_PLACEMENT_3D ( 'NONE', #55554, #68924, #92420 ) ;
#19656=DIRECTION ( 'NONE',  ( -0.7414773880254664773, 0.000000000000000000, 0.6709778558543730842 ) ) ;
#19658=CARTESIAN_POINT ( 'NONE',  ( -19.39983987834945012, 1522.861859112239244, 178.9515629540100861 ) ) ;
#19670=CARTESIAN_POINT ( 'NONE',  ( -17.17241001986462123, 1518.913060387330006, 238.6251415217917895 ) ) ;
#19675=AXIS2_PLACEMENT_3D ( 'NONE', #45189, #96683, #62564 ) ;
#19679=CARTESIAN_POINT ( 'NONE',  ( -32.77044109517562021, 1525.581535527370534, 219.1629015078874829 ) ) ;
#19686=FACE_OUTER_BOUND ( 'NONE', #33473, .T. ) ;
#19690=AXIS2_PLACEMENT_3D ( 'NONE', #110486, #70586, #36942 ) ;
#19692=EDGE_CURVE ( 'NONE', #967, #80823, #97869, .T. ) ;
#19693=DIRECTION ( 'NONE',  ( 0.000000000000000000, 0.000000000000000000, -1.000000000000000000 ) ) ;
#19699=CARTESIAN_POINT ( 'NONE',  ( 31.97743984922253446, 1525.878013734321485, 198.0760624713124969 ) ) ;
#19701=CARTESIAN_POINT ( 'NONE',  ( 0.000000000000000000, 1512.187213306747481, 209.1218459616979999 ) ) ;
#19705=CARTESIAN_POINT ( 'NONE',  ( 20.07149347155292318, 1526.186458717542791, 233.0642689910310139 ) ) ;
#19708=DIRECTION ( 'NONE',  ( 0.000000000000000000, 1.000000000000000000, -0.000000000000000000 ) ) ;
#19718=TOROIDAL_SURFACE ( 'NONE', #14352, 24.69926344187880929, 1.000000000000000000 ) ;
#19748=CARTESIAN_POINT ( 'NONE',  ( 0.000000000000000000, 1523.409940573003951, 185.4225825198192013 ) ) ;
#19798=DIRECTION ( 'NONE',  ( -0.9510565162951500895, 0.000000000000000000, 0.3090169943749582759 ) ) ;
#19803=CARTESIAN_POINT ( 'NONE',  ( 30.95751052620453336, 1525.821544997590308, 216.7905424461071959 ) ) ;
#19821=CARTESIAN_POINT ( 'NONE',  ( -30.31052258194577931, 1523.604703353109699, 222.4930856806594193 ) ) ;
#19822=CARTESIAN_POINT ( 'NONE',  ( 33.36586802512172767, 1523.382868172864164, 201.9069332299488906 ) ) ;
#19846=ORIENTED_EDGE ( 'NONE', *, *, #89809, .F. ) ;
#19853=ADVANCED_FACE ( 'NONE', ( #40970 ), #93022, .F. ) ;
#19863=ORIENTED_EDGE ( 'NONE', *, *, #75838, .T. ) ;
#19871=CARTESIAN_POINT ( 'NONE',  ( -31.65139097221453923, 1525.320849883639085, 202.0582317240186399 ) ) ;
#19878=ORIENTED_EDGE ( 'NONE', *, *, #109794, .F. ) ;
#19891=EDGE_CURVE ( 'NONE', #35843, #97183, #40654, .T. ) ;
#19899=EDGE_CURVE ( 'NONE', #63441, #7367, #57616, .T. ) ;
#19907=DIRECTION ( 'NONE',  ( 0.000000000000000000, 1.000000000000000000, 0.000000000000000000 ) ) ;
#19908=AXIS2_PLACEMENT_3D ( 'NONE', #39227, #39794, #30276 ) ;
#19923=VECTOR ( 'NONE', #100499, 1000.000000000000114 ) ;
#19940=ORIENTED_EDGE ( 'NONE', *, *, #3780, .T. ) ;
#19941=AXIS2_PLACEMENT_3D ( 'NONE', #103258, #85360, #16488 ) ;
#19944=CARTESIAN_POINT ( 'NONE',  ( -21.84020450222076448, 1523.382868172864164, 183.2638850454220858 ) ) ;
#19945=LINE ( 'NONE', #63108, #107423 ) ;
#19948=CARTESIAN_POINT ( 'NONE',  ( -29.41145171355100985, 1525.795403621571040, 196.6862065453202320 ) ) ;
#19963=CARTESIAN_POINT ( 'NONE',  ( 1.682117298743263101, 1526.345556099435953, 239.7639272011427636 ) ) ;
#19964=CARTESIAN_POINT ( 'NONE',  ( -3.143084115766277886, 1525.137906803777241, 241.5427217869176104 ) ) ;
#19967=DIRECTION ( 'NONE',  ( 0.4978433412588729179, 0.000000000000000000, -0.8672669759446635096 ) ) ;
#19973=DIRECTION ( 'NONE',  ( 0.000000000000000000, 1.000000000000000000, 0.000000000000000000 ) ) ;
#19982=CARTESIAN_POINT ( 'NONE',  ( 31.64580750758049632, 1523.313115944344872, 221.9353285378996361 ) ) ;
#19990=AXIS2_PLACEMENT_3D ( 'NONE', #13635, #98216, #80878 ) ;
#20000=DIRECTION ( 'NONE',  ( 0.000000000000000000, 1.000000000000000000, 0.000000000000000000 ) ) ;
#20012=DIRECTION ( 'NONE',  ( -1.000000000000000000, 0.000000000000000000, 0.000000000000000000 ) ) ;
#20023=CIRCLE ( 'NONE', #82621, 2.000000000000001776 ) ;
#20036=DIRECTION ( 'NONE',  ( 0.000000000000000000, 0.000000000000000000, -1.000000000000000000 ) ) ;
#20041=EDGE_CURVE ( 'NONE', #55773, #97968, #58777, .T. ) ;
#20043=DIRECTION ( 'NONE',  ( -0.000000000000000000, -1.000000000000000000, -0.000000000000000000 ) ) ;
#20068=DIRECTION ( 'NONE',  ( -0.2054769195713296304, -0.000000000000000000, 0.9786619618251631847 ) ) ;
#20070=EDGE_CURVE ( 'NONE', #50617, #103878, #26418, .T. ) ;
#20085=DIRECTION ( 'NONE',  ( -0.9510565162951518658, 0.000000000000000000, 0.3090169943749528914 ) ) ;
#20091=B_SPLINE_CURVE_WITH_KNOTS ( 'NONE', 3,
 ( #60915, #35129, #69311, #105101 ),
 .UNSPECIFIED., .F., .F.,
 ( 4, 4 ),
 ( 0.000000000000000000, 0.0002220129587134773411 ),
 .UNSPECIFIED. ) ;
#20092=CARTESIAN_POINT ( 'NONE',  ( -19.39983987835376666, 1501.977400791986611, 239.2921289694225777 ) ) ;
#20134=CARTESIAN_POINT ( 'NONE',  ( -31.40702543711121209, 1523.611961620354123, 221.9096305968283787 ) ) ;
#20136=CARTESIAN_POINT ( 'NONE',  ( 32.16538354510014130, 1524.524650307243746, 202.1429721374758230 ) ) ;
#20159=CARTESIAN_POINT ( 'NONE',  ( 17.84338787571943996, 1523.382868172864164, 237.8836641337660467 ) ) ;
#20169=CARTESIAN_POINT ( 'NONE',  ( 20.12564951288285897, 1511.187213306747708, 237.5287294252014192 ) ) ;
#20201=ORIENTED_EDGE ( 'NONE', *, *, #76019, .T. ) ;
#20210=VERTEX_POINT ( 'NONE', #85649 ) ;
#20219=DIRECTION ( 'NONE',  ( 0.05752486295818592249, -0.9969860201949396483, -0.05205540968523067469 ) ) ;
#20231=DIRECTION ( 'NONE',  ( 0.000000000000000000, 0.000000000000000000, -1.000000000000000000 ) ) ;
#20249=CARTESIAN_POINT ( 'NONE',  ( 18.66420869458052323, 1526.382868172864164, 232.7837831374276902 ) ) ;
#20256=CARTESIAN_POINT ( 'NONE',  ( -2.470168521978402421, 1523.382868172864164, 175.3649660270905599 ) ) ;
#20284=VERTEX_POINT ( 'NONE', #42559 ) ;
#20290=( BOUNDED_SURFACE ( )  B_SPLINE_SURFACE ( 3, 2, ( 
 ( #82245, #39696, #86929 ),
 ( #31288, #52798, #99581 ),
 ( #29633, #106885, #63818 ),
 ( #21201, #38580, #73305 ),
 ( #81675, #55410, #89542 ),
 ( #90081, #81137, #72759 ),
 ( #64367, #98489, #21757 ),
 ( #55958, #13365, #4981 ),
 ( #30736, #68237, #16123 ),
 ( #58165, #22864, #109659 ) ),
 .UNSPECIFIED., .F., .F., .F. ) 
 B_SPLINE_SURFACE_WITH_KNOTS ( ( 4, 2, 2, 2, 4 ),
 ( 3, 3 ),
 ( 0.000000000000000000, 0.3926990816987241395, 0.7853981633974482790, 1.178097245096172418, 1.570796326794896558 ),
 ( 0.000000000000000000, 1.000000000000000000 ),
 .UNSPECIFIED. ) 
 GEOMETRIC_REPRESENTATION_ITEM ( )  RATIONAL_B_SPLINE_SURFACE ( (
 ( 1.000000000000000000, 0.7763623250684366095, 1.000000000000000000),
 ( 1.000000000000000000, 0.7763684247028493912, 1.000000000000000000),
 ( 1.000000000000000000, 0.7746454561806210837, 1.000000000000000000),
 ( 1.000000000000000000, 0.7679730451964270621, 1.000000000000000000),
 ( 1.000000000000000000, 0.7630177051946732680, 1.000000000000000000),
 ( 1.000000000000000000, 0.7504512394528241037, 1.000000000000000000),
 ( 1.000000000000000000, 0.7428408967931674489, 1.000000000000000000),
 ( 1.000000000000000000, 0.7259222650905756691, 1.000000000000000000),
 ( 1.000000000000000000, 0.7166207884823141416, 1.000000000000000000),
 ( 1.000000000000000000, 0.7071067811865875408, 1.000000000000000000) ) ) 
 REPRESENTATION_ITEM ( '' )  SURFACE ( )  );
#20299=DIRECTION ( 'NONE',  ( 0.05752486295818382001, -0.9969860201949398704, 0.05205540968523099388 ) ) ;
#20303=EDGE_LOOP ( 'NONE', ( #35400, #23184, #16005, #28543 ) ) ;
#20306=VECTOR ( 'NONE', #110786, 999.9999999999998863 ) ;
#20319=ORIENTED_EDGE ( 'NONE', *, *, #16591, .F. ) ;
#20347=CARTESIAN_POINT ( 'NONE',  ( -16.88555894881161379, 1525.556090473946824, 236.5668007256133194 ) ) ;
#20351=CARTESIAN_POINT ( 'NONE',  ( -32.86802468386297704, 1523.382868172864164, 201.0396662540046577 ) ) ;
#20367=CARTESIAN_POINT ( 'NONE',  ( -0.4151546846821903003, 1512.187213306747481, 242.9330574173806951 ) ) ;
#20381=VECTOR ( 'NONE', #91408, 1000.000000000000114 ) ;
#20407=ORIENTED_EDGE ( 'NONE', *, *, #22164, .T. ) ;
#20410=CARTESIAN_POINT ( 'NONE',  ( -20.12564951288246107, 1511.187213306747708, 237.5287294252017603 ) ) ;
#20423=ORIENTED_EDGE ( 'NONE', *, *, #77871, .T. ) ;
#20424=CARTESIAN_POINT ( 'NONE',  ( -16.53175237170781386, 1526.069472839389164, 182.3016483747010739 ) ) ;
#20428=DIRECTION ( 'NONE',  ( 0.000000000000000000, 0.000000000000000000, 1.000000000000000000 ) ) ;
#20438=CARTESIAN_POINT ( 'NONE',  ( -28.81649562247343255, 1526.349689584397083, 220.0454131225313574 ) ) ;
#20442=CARTESIAN_POINT ( 'NONE',  ( -30.01999557802949070, 1525.848196786131666, 197.1136699524750213 ) ) ;
#20446=AXIS2_PLACEMENT_3D ( 'NONE', #49403, #39338, #4639 ) ;
#20454=CARTESIAN_POINT ( 'NONE',  ( -30.31052258194575444, 1523.604703353109926, 222.4930856806594477 ) ) ;
#20467=DIRECTION ( 'NONE',  ( -0.9125304618754024322, 0.000000000000000000, -0.4090087482554191078 ) ) ;
#20472=ORIENTED_EDGE ( 'NONE', *, *, #67354, .F. ) ;
#20474=CIRCLE ( 'NONE', #54515, 2.000000000000001776 ) ;
#20491=ORIENTED_EDGE ( 'NONE', *, *, #22127, .T. ) ;
#20519=CARTESIAN_POINT ( 'NONE',  ( -32.86802468386279941, 1512.187213306747481, 217.2040256693919957 ) ) ;
#20523=TOROIDAL_SURFACE ( 'NONE', #77700, 2.000000000000000000, 1.000000000000000000 ) ;
#20530=TOROIDAL_SURFACE ( 'NONE', #47332, 1.000000000000000000, 1.000000000000000000 ) ;
#20553=VERTEX_POINT ( 'NONE', #78374 ) ;
#20560=ORIENTED_EDGE ( 'NONE', *, *, #69826, .T. ) ;
#20573=EDGE_LOOP ( 'NONE', ( #86275, #89176, #55454, #75295 ) ) ;
#20574=VERTEX_POINT ( 'NONE', #10623 ) ;
#20586=ORIENTED_EDGE ( 'NONE', *, *, #58975, .T. ) ;
#20592=CARTESIAN_POINT ( 'NONE',  ( 20.20959865099471031, 1501.977400791986611, 182.0120230947219966 ) ) ;
#20603=DIRECTION ( 'NONE',  ( -0.8200914087126203178, -0.4884709562387607451, 0.2980708074718837475 ) ) ;
#20605=LINE ( 'NONE', #19518, #67010 ) ;
#20609=AXIS2_PLACEMENT_3D ( 'NONE', #48639, #13889, #100119 ) ;
#20612=CARTESIAN_POINT ( 'NONE',  ( -0.4151546846821903003, 1522.382868172863937, 173.3106345060153046 ) ) ;
#20620=VERTEX_POINT ( 'NONE', #84965 ) ;
#20622=CARTESIAN_POINT ( 'NONE',  ( 16.66231036550724198, 1523.604703353109699, 237.7554842931445478 ) ) ;
#20623=DIRECTION ( 'NONE',  ( 0.000000000000000000, 1.000000000000000000, 0.000000000000000000 ) ) ;
#20624=CARTESIAN_POINT ( 'NONE',  ( -2.165176160182525233, 1526.186458717538699, 240.2894009330203744 ) ) ;
#20646=AXIS2_PLACEMENT_3D ( 'NONE', #53122, #20043, #77758 ) ;
#20653=FACE_OUTER_BOUND ( 'NONE', #106697, .T. ) ;
#20664=EDGE_CURVE ( 'NONE', #13899, #90367, #20091, .T. ) ;
#20678=CARTESIAN_POINT ( 'NONE',  ( 31.32995031131198616, 1523.678648413191695, 221.9013357025044115 ) ) ;
#20684=CARTESIAN_POINT ( 'NONE',  ( 33.13357216314881981, 1523.313115944345327, 200.8872321731301156 ) ) ;
#20685=AXIS2_PLACEMENT_3D ( 'NONE', #10854, #19211, #2479 ) ;
#20686=EDGE_LOOP ( 'NONE', ( #105973, #78555, #91656, #4436 ) ) ;
#20712=ORIENTED_EDGE ( 'NONE', *, *, #80874, .T. ) ;
#20716=ADVANCED_FACE ( 'NONE', ( #11045 ), #3220, .T. ) ;
#20717=DIRECTION ( 'NONE',  ( 0.000000000000000000, 0.000000000000000000, 1.000000000000000000 ) ) ;
#20718=ORIENTED_EDGE ( 'NONE', *, *, #32164, .T. ) ;
#20725=CARTESIAN_POINT ( 'NONE',  ( 0.4992773797353681764, 1524.841055067849766, 174.1119671515087077 ) ) ;
#20734=DIRECTION ( 'NONE',  ( 0.000000000000000000, 0.000000000000000000, 1.000000000000000000 ) ) ;
#20753=EDGE_CURVE ( 'NONE', #98801, #89436, #22635, .T. ) ;
#20754=FACE_OUTER_BOUND ( 'NONE', #19068, .T. ) ;
#20763=CARTESIAN_POINT ( 'NONE',  ( -21.61975802670946933, 1524.130440953581001, 234.4879735737366673 ) ) ;
#20782=DIRECTION ( 'NONE',  ( -0.7414773880254650340, 5.145032927655519758E-15, 0.6709778558543747495 ) ) ;
#20796=CARTESIAN_POINT ( 'NONE',  ( 17.84054676580419141, 1523.580203803270933, 180.3625987673424618 ) ) ;
#20807=DIRECTION ( 'NONE',  ( 0.9125304618753903307, 0.000000000000000000, -0.4090087482554460863 ) ) ;
#20818=CIRCLE ( 'NONE', #72717, 1.000000000000000888 ) ;
#20828=EDGE_CURVE ( 'NONE', #20993, #96103, #6749, .T. ) ;
#20851=B_SPLINE_CURVE_WITH_KNOTS ( 'NONE', 3,
 ( #40510, #47818, #30457, #6362 ),
 .UNSPECIFIED., .F., .F.,
 ( 4, 4 ),
 ( 0.000000000000000000, 0.0002960034161023850021 ),
 .UNSPECIFIED. ) ;
#20856=CARTESIAN_POINT ( 'NONE',  ( 32.39800393421785429, 1524.816548299036867, 217.0524289663465538 ) ) ;
#20865=DIRECTION ( 'NONE',  ( -0.000000000000000000, -1.000000000000000000, -0.000000000000000000 ) ) ;
#20891=CARTESIAN_POINT ( 'NONE',  ( 30.00906612072600765, 1525.856065479257722, 221.1186961711726155 ) ) ;
#20894=CARTESIAN_POINT ( 'NONE',  ( -16.62425451295051104, 1524.075000532257263, 237.7045424426785019 ) ) ;
#20935=( BOUNDED_SURFACE ( )  B_SPLINE_SURFACE ( 3, 2, ( 
 ( #54290, #88416, #45879 ),
 ( #3337, #105783, #63249 ),
 ( #97358, #88955, #46436 ),
 ( #80568, #55377, #91164 ),
 ( #65997, #108517, #31808 ),
 ( #64333, #13884, #106849 ) ),
 .UNSPECIFIED., .F., .F., .F. ) 
 B_SPLINE_SURFACE_WITH_KNOTS ( ( 4, 2, 4 ),
 ( 3, 3 ),
 ( -2.168404344971008868E-17, 0.001312027981647260989, 0.002624055963294543662 ),
 ( 0.000000000000000000, 1.000000000000000000 ),
 .UNSPECIFIED. ) 
 GEOMETRIC_REPRESENTATION_ITEM ( )  RATIONAL_B_SPLINE_SURFACE ( (
 ( 1.000000000000000000, 0.9376006582765930020, 1.000000000000000000),
 ( 1.000000000000000000, 0.9569320108022597582, 1.000000000000000000),
 ( 1.000000000000000000, 0.9725743441618913687, 1.000000000000000000),
 ( 1.000000000000000000, 0.9942095667135614212, 1.000000000000000000),
 ( 1.000000000000000000, 1.000043666450708191, 1.000000000000000000),
 ( 1.000000000000000000, 1.000000000000000000, 1.000000000000000000) ) ) 
 REPRESENTATION_ITEM ( '' )  SURFACE ( )  );
#20964=EDGE_CURVE ( 'NONE', #71433, #54724, #32402, .T. ) ;
#20965=CARTESIAN_POINT ( 'NONE',  ( -31.34137657934026677, 1523.382868172864164, 196.3411265156551906 ) ) ;
#20975=FACE_OUTER_BOUND ( 'NONE', #98264, .T. ) ;
#20993=VERTEX_POINT ( 'NONE', #71958 ) ;
#20996=CIRCLE ( 'NONE', #62134, 1.000000000000000888 ) ;
#21002=CIRCLE ( 'NONE', #63981, 1.000000000000001554 ) ;
#21012=ORIENTED_EDGE ( 'NONE', *, *, #1467, .T. ) ;
#21048=CARTESIAN_POINT ( 'NONE',  ( -17.27380198137636214, 1525.712835404586031, 236.6835154643348460 ) ) ;
#21049=CARTESIAN_POINT ( 'NONE',  ( 30.60907494343232571, 1526.073429442291854, 216.5595792582588501 ) ) ;
#21051=CARTESIAN_POINT ( 'NONE',  ( -3.261863598262784603, 1524.739915903631982, 241.7744910610305169 ) ) ;
#21073=AXIS2_PLACEMENT_3D ( 'NONE', #88161, #104948, #59781 ) ;
#21078=AXIS2_PLACEMENT_3D ( 'NONE', #19138, #79096, #95873 ) ;
#21079=CARTESIAN_POINT ( 'NONE',  ( -0.4151546846821905778, 1522.382868172863937, 244.9330574173806951 ) ) ;
#21093=FACE_OUTER_BOUND ( 'NONE', #87540, .T. ) ;
#21131=VERTEX_POINT ( 'NONE', #92555 ) ;
#21144=CYLINDRICAL_SURFACE ( 'NONE', #45970, 1.999999999999996669 ) ;
#21145=AXIS2_PLACEMENT_3D ( 'NONE', #62027, #27846, #19425 ) ;
#21147=VERTEX_POINT ( 'NONE', #23143 ) ;
#21150=DIRECTION ( 'NONE',  ( 0.000000000000000000, -0.07083107041561081951, -0.9974883254774358221 ) ) ;
#21162=CARTESIAN_POINT ( 'NONE',  ( 0.5890887500919901321, 1526.382868172863937, 243.2762031678882977 ) ) ;
#21170=DIRECTION ( 'NONE',  ( 0.000000000000000000, 1.000000000000000000, 0.000000000000000000 ) ) ;
#21176=FACE_OUTER_BOUND ( 'NONE', #96653, .T. ) ;
#21177=ORIENTED_EDGE ( 'NONE', *, *, #104951, .F. ) ;
#21182=CYLINDRICAL_SURFACE ( 'NONE', #62652, 0.9999999999999970024 ) ;
#21190=CARTESIAN_POINT ( 'NONE',  ( -30.25425994617014780, 1522.382868172863937, 199.2916410102373277 ) ) ;
#21196=CARTESIAN_POINT ( 'NONE',  ( 20.71343476517534299, 1512.187213306747481, 238.3377464195763764 ) ) ;
#21201=CARTESIAN_POINT ( 'NONE',  ( 20.37381179411493548, 1524.397344074318880, 237.9604625470743997 ) ) ;
#21211=CARTESIAN_POINT ( 'NONE',  ( 2.738357492517908387, 1525.795403621571040, 177.3070692402450845 ) ) ;
#21219=AXIS2_PLACEMENT_3D ( 'NONE', #75978, #23898, #74354 ) ;
#21220=DIRECTION ( 'NONE',  ( 0.000000000000000000, 0.000000000000000000, -1.000000000000000000 ) ) ;
#21227=( BOUNDED_CURVE ( )  B_SPLINE_CURVE ( 3, ( #20612, #31238, #82749, #107391 ),
 .UNSPECIFIED., .F., .F. ) 
 B_SPLINE_CURVE_WITH_KNOTS ( ( 4, 4 ),
 ( 3.141592653589793116, 4.712388980384689674 ),
 .UNSPECIFIED. ) 
 CURVE ( )  GEOMETRIC_REPRESENTATION_ITEM ( )  RATIONAL_B_SPLINE_CURVE ( ( 1.000000000000000000, 0.8047378541243649375, 0.8047378541243649375, 1.000000000000000000 ) ) 
 REPRESENTATION_ITEM ( '' )  );
#21237=VERTEX_POINT ( 'NONE', #42725 ) ;
#21238=ORIENTED_EDGE ( 'NONE', *, *, #45772, .T. ) ;
#21245=CARTESIAN_POINT ( 'NONE',  ( 17.04790460296295507, 1526.208281990540172, 235.6077665793653466 ) ) ;
#21247=EDGE_CURVE ( 'NONE', #44154, #3217, #43286, .T. ) ;
#21250=CARTESIAN_POINT ( 'NONE',  ( -31.23437356469425907, 1523.382868172864164, 221.8968241038847964 ) ) ;
#21264=ADVANCED_FACE ( 'NONE', ( #89135 ), #76534, .F. ) ;
#21268=DIRECTION ( 'NONE',  ( 0.9942586961433758086, 0.000000000000000000, 0.1070030146457303932 ) ) ;
#21286=EDGE_CURVE ( 'NONE', #101260, #81031, #88056, .T. ) ;
#21296=EDGE_CURVE ( 'NONE', #65505, #26062, #71835, .T. ) ;
#21308=DIRECTION ( 'NONE',  ( 0.000000000000000000, 1.000000000000000000, -0.000000000000000000 ) ) ;
#21317=CARTESIAN_POINT ( 'NONE',  ( 20.71343476517376558, 1522.906561336852974, 179.9059455038184581 ) ) ;
#21326=CARTESIAN_POINT ( 'NONE',  ( 20.92767404034517753, 1512.187213306747481, 235.3888156262294444 ) ) ;
#21330=AXIS2_PLACEMENT_3D ( 'NONE', #103227, #42246, #16996 ) ;
#21338=CARTESIAN_POINT ( 'NONE',  ( -31.12456774391181469, 1525.960063244516959, 201.1524202391567258 ) ) ;
#21343=EDGE_CURVE ( 'NONE', #20574, #32804, #80741, .T. ) ;
#21346=DIRECTION ( 'NONE',  ( -0.000000000000000000, -1.000000000000000000, -0.000000000000000000 ) ) ;
#21352=CARTESIAN_POINT ( 'NONE',  ( 4.097009089535375459, 1512.187213306747481, 201.1608118946568311 ) ) ;
#21356=CARTESIAN_POINT ( 'NONE',  ( -32.02808312589908013, 1511.187213306747708, 219.9649204700466782 ) ) ;
#21362=ORIENTED_EDGE ( 'NONE', *, *, #56853, .F. ) ;
#21369=ORIENTED_EDGE ( 'NONE', *, *, #95300, .F. ) ;
#21375=AXIS2_PLACEMENT_3D ( 'NONE', #442, #35113, #26706 ) ;
#21385=ORIENTED_EDGE ( 'NONE', *, *, #83639, .F. ) ;
#21387=CARTESIAN_POINT ( 'NONE',  ( -17.04521188157725931, 1526.211528530236592, 235.5955628457882653 ) ) ;
#21395=AXIS2_PLACEMENT_3D ( 'NONE', #51219, #87023, #34417 ) ;
#21401=CARTESIAN_POINT ( 'NONE',  ( 34.18677586421181758, 1501.977400791986611, 198.4504086008745389 ) ) ;
#21403=EDGE_LOOP ( 'NONE', ( #24724, #94354, #49724, #40139 ) ) ;
#21409=EDGE_CURVE ( 'NONE', #80799, #26062, #69381, .T. ) ;
#21411=CARTESIAN_POINT ( 'NONE',  ( -17.19739463999666285, 1525.960063244516959, 181.9833109756550584 ) ) ;
#21424=ADVANCED_FACE ( 'NONE', ( #44120 ), #3239, .T. ) ;
#21425=CARTESIAN_POINT ( 'NONE',  ( -2.472529913803022783, 1523.678648413191695, 242.8674788698241400 ) ) ;
#21438=CARTESIAN_POINT ( 'NONE',  ( 16.73628186595820111, 1526.382868172864164, 184.0591879540915841 ) ) ;
#21440=DIRECTION ( 'NONE',  ( 0.6709778558543737503, 0.000000000000000000, 0.7414773880254658112 ) ) ;
#21454=VECTOR ( 'NONE', #8055, 1000.000000000000000 ) ;
#21460=AXIS2_PLACEMENT_3D ( 'NONE', #98916, #30621, #4333 ) ;
#21473=CARTESIAN_POINT ( 'NONE',  ( 31.32941717379424063, 1525.856064936179791, 217.0550765750803350 ) ) ;
#21481=CARTESIAN_POINT ( 'NONE',  ( -20.21024070146840046, 1526.107876515966382, 233.6897457629616213 ) ) ;
#21497=ORIENTED_EDGE ( 'NONE', *, *, #96302, .F. ) ;
#21506=AXIS2_PLACEMENT_3D ( 'NONE', #56043, #6724, #108080 ) ;
#21507=B_SPLINE_CURVE_WITH_KNOTS ( 'NONE', 3,
 ( #35839, #105246, #104136, #53202 ),
 .UNSPECIFIED., .F., .F.,
 ( 4, 4 ),
 ( 0.000000000000000000, 0.0002960034161023848936 ),
 .UNSPECIFIED. ) ;
#21508=EDGE_CURVE ( 'NONE', #92642, #90688, #78302, .T. ) ;
#21509=CARTESIAN_POINT ( 'NONE',  ( -30.31940284292427634, 1523.382868172864164, 195.7503880523418616 ) ) ;
#21518=CARTESIAN_POINT ( 'NONE',  ( 21.28825147355426495, 1525.253972588462830, 234.3567090158657891 ) ) ;
#21535=DIRECTION ( 'NONE',  ( 0.000000000000000000, 1.000000000000000000, 0.000000000000000000 ) ) ;
#21547=EDGE_CURVE ( 'NONE', #105727, #15990, #92603, .T. ) ;
#21555=CARTESIAN_POINT ( 'NONE',  ( 28.49879435371743241, 1526.382868173645875, 198.4011524119004264 ) ) ;
#21556=CARTESIAN_POINT ( 'NONE',  ( -30.04668324475537844, 1524.739563915923100, 222.3144186811225609 ) ) ;
#21563=EDGE_LOOP ( 'NONE', ( #70873, #35824, #29953, #95496 ) ) ;
#21577=ORIENTED_EDGE ( 'NONE', *, *, #28927, .T. ) ;
#21581=ORIENTED_EDGE ( 'NONE', *, *, #58489, .T. ) ;
#21589=AXIS2_PLACEMENT_3D ( 'NONE', #28793, #86476, #43937 ) ;
#21605=CARTESIAN_POINT ( 'NONE',  ( -2.622430729443003816, 1523.621879633029039, 242.1535192357228254 ) ) ;
#21618=DIRECTION ( 'NONE',  ( -0.1070030146457234405, 0.000000000000000000, 0.9942586961433764747 ) ) ;
#21627=DIRECTION ( 'NONE',  ( 0.000000000000000000, 0.000000000000000000, -1.000000000000000000 ) ) ;
#21632=AXIS2_PLACEMENT_3D ( 'NONE', #110085, #42890, #42328 ) ;
#21653=EDGE_LOOP ( 'NONE', ( #18726, #24658, #109328, #45806 ) ) ;
#21663=VECTOR ( 'NONE', #77505, 1000.000000000000000 ) ;
#21665=CARTESIAN_POINT ( 'NONE',  ( -30.51231035492510557, 1524.382868172863937, 218.1578534183722979 ) ) ;
#21673=ORIENTED_EDGE ( 'NONE', *, *, #105511, .F. ) ;
#21699=CARTESIAN_POINT ( 'NONE',  ( 30.61115703707575264, 1523.542365884046148, 221.8239785241844686 ) ) ;
#21706=CARTESIAN_POINT ( 'NONE',  ( 34.18677586421181758, 1512.187213306747481, 198.4504086008745389 ) ) ;
#21718=ORIENTED_EDGE ( 'NONE', *, *, #74781, .T. ) ;
#21738=CARTESIAN_POINT ( 'NONE',  ( -31.54873523817366632, 1525.317349363549965, 216.6695393792268192 ) ) ;
#21756=ORIENTED_EDGE ( 'NONE', *, *, #60512, .T. ) ;
#21757=CARTESIAN_POINT ( 'NONE',  ( 17.44374831407513682, 1524.130440953581001, 237.5220222273273976 ) ) ;
#21759=VECTOR ( 'NONE', #36534, 1000.000000000000000 ) ;
#21777=VERTEX_POINT ( 'NONE', #59684 ) ;
#21792=B_SPLINE_CURVE_WITH_KNOTS ( 'NONE', 3,
 ( #68225, #32923, #102332, #40784 ),
 .UNSPECIFIED., .F., .F.,
 ( 4, 4 ),
 ( 0.000000000000000000, 0.0002220129587134773411 ),
 .UNSPECIFIED. ) ;
#21794=ORIENTED_EDGE ( 'NONE', *, *, #91290, .F. ) ;
#21802=CARTESIAN_POINT ( 'NONE',  ( 16.73628186595829703, 1526.382868172864164, 234.1845039693042452 ) ) ;
#21808=ORIENTED_EDGE ( 'NONE', *, *, #62503, .F. ) ;
#21814=CARTESIAN_POINT ( 'NONE',  ( 2.383407846123591689, 1522.906363951597314, 174.9517353176829602 ) ) ;
#21818=CARTESIAN_POINT ( 'NONE',  ( 20.12564951288285542, 1511.187213306747708, 237.5287294252014192 ) ) ;
#21824=CARTESIAN_POINT ( 'NONE',  ( 29.95987888842581981, 1525.317359687823455, 196.6841832611087284 ) ) ;
#21829=ORIENTED_EDGE ( 'NONE', *, *, #62533, .F. ) ;
#21831=CIRCLE ( 'NONE', #2234, 0.9999999999999981126 ) ;
#21844=CARTESIAN_POINT ( 'NONE',  ( -34.68852446352935459, 1501.977400791986611, 218.2490599186011764 ) ) ;
#21848=CARTESIAN_POINT ( 'NONE',  ( -20.71343476517491311, 1522.382868172863937, 238.3377464195766890 ) ) ;
#21850=DIRECTION ( 'NONE',  ( 0.000000000000000000, 1.000000000000000000, 0.000000000000000000 ) ) ;
#21856=LINE ( 'NONE', #54432, #45989 ) ;
#21861=CARTESIAN_POINT ( 'NONE',  ( 16.87900699709538799, 1524.382868172804365, 181.2327155136467809 ) ) ;
#21883=VERTEX_POINT ( 'NONE', #60233 ) ;
#21885=ADVANCED_FACE ( 'NONE', ( #92169 ), #8699, .T. ) ;
#21891=DIRECTION ( 'NONE',  ( 0.000000000000000000, 0.000000000000000000, 1.000000000000000000 ) ) ;
#21902=DIRECTION ( 'NONE',  ( 0.000000000000000000, 1.000000000000000000, 0.000000000000000000 ) ) ;
#21907=ORIENTED_EDGE ( 'NONE', *, *, #44061, .F. ) ;
#21914=ORIENTED_EDGE ( 'NONE', *, *, #35693, .T. ) ;
#21926=EDGE_CURVE ( 'NONE', #53780, #92019, #41314, .T. ) ;
#21961=CARTESIAN_POINT ( 'NONE',  ( -21.19880661589042248, 1524.382868172863937, 184.6948938244650833 ) ) ;
#21967=PRODUCT_DEFINITION ( 'UNKNOWN', '', #26123, #86055 ) ;
#21981=CARTESIAN_POINT ( 'NONE',  ( 17.12202622827918219, 1526.104292489127602, 182.3009725563080963 ) ) ;
#21994=DIRECTION ( 'NONE',  ( 0.000000000000000000, 1.000000000000000000, 0.000000000000000000 ) ) ;
#22015=CARTESIAN_POINT ( 'NONE',  ( 32.28368668151611587, 1524.972383263452684, 217.0406336501054341 ) ) ;
#22029=CARTESIAN_POINT ( 'NONE',  ( 17.17241001986483795, 1512.187213306747481, 180.6185504016043240 ) ) ;
#22060=CARTESIAN_POINT ( 'NONE',  ( -17.12202622829238052, 1526.104292489134423, 182.3009725563086931 ) ) ;
#22063=EDGE_LOOP ( 'NONE', ( #55861, #85699, #54004, #76029 ) ) ;
#22067=CARTESIAN_POINT ( 'NONE',  ( -28.44964981547095917, 1526.382868172864164, 198.3640452512632351 ) ) ;
#22069=DIRECTION ( 'NONE',  ( 0.000000000000000000, 0.000000000000000000, 1.000000000000000000 ) ) ;
#22072=ORIENTED_EDGE ( 'NONE', *, *, #89939, .F. ) ;
#22083=CARTESIAN_POINT ( 'NONE',  ( 2.356903266504112082, 1525.394057003702756, 176.3139131587520012 ) ) ;
#22099=CARTESIAN_POINT ( 'NONE',  ( 17.22845748920278197, 1525.848198008145346, 181.7617192448029186 ) ) ;
#22122=DIRECTION ( 'NONE',  ( 0.9786619618251657382, 0.000000000000000000, 0.2054769195713179730 ) ) ;
#22127=EDGE_CURVE ( 'NONE', #99467, #73683, #99791, .T. ) ;
#22133=FACE_OUTER_BOUND ( 'NONE', #61537, .T. ) ;
#22146=CIRCLE ( 'NONE', #11483, 33.13701971169416538 ) ;
#22147=DIRECTION ( 'NONE',  ( 0.3090169943749582204, -0.000000000000000000, 0.9510565162951499785 ) ) ;
#22164=EDGE_CURVE ( 'NONE', #13345, #40573, #18294, .T. ) ;
#22172=CARTESIAN_POINT ( 'NONE',  ( -2.383407846123591689, 1522.906363951597314, 243.2919566057130396 ) ) ;
#22183=LINE ( 'NONE', #97261, #49779 ) ;
#22254=FACE_OUTER_BOUND ( 'NONE', #1963, .T. ) ;
#22256=CARTESIAN_POINT ( 'NONE',  ( -21.38516915558008336, 1524.726013923371283, 180.3939891059723664 ) ) ;
#22259=CARTESIAN_POINT ( 'NONE',  ( -21.53981368633656857, 1523.542365884045694, 183.9340804168635088 ) ) ;
#22265=CIRCLE ( 'NONE', #29407, 0.9999999999999991118 ) ;
#22267=CARTESIAN_POINT ( 'NONE',  ( 0.000000000000000000, 1511.187213306747708, 209.1218459616979999 ) ) ;
#22286=CARTESIAN_POINT ( 'NONE',  ( -31.56779946216799360, 1525.408327360765952, 216.2063941007895380 ) ) ;
#22289=VERTEX_POINT ( 'NONE', #5411 ) ;
#22297=CARTESIAN_POINT ( 'NONE',  ( 3.348647037815445149, 1523.530870145311383, 242.0864809827354520 ) ) ;
#22302=CARTESIAN_POINT ( 'NONE',  ( 19.59884465730837277, 1526.382868172864164, 237.0995590530538948 ) ) ;
#22303=EDGE_CURVE ( 'NONE', #58921, #94817, #22183, .T. ) ;
#22328=DIRECTION ( 'NONE',  ( 0.5877852522924709167, 0.000000000000000000, 0.8090169943749491166 ) ) ;
#22340=VERTEX_POINT ( 'NONE', #67546 ) ;
#22342=CARTESIAN_POINT ( 'NONE',  ( -2.372478608332516892, 1501.977400791986611, 174.8996806668726549 ) ) ;
#22344=EDGE_LOOP ( 'NONE', ( #34277, #14674, #28041, #48305, #87760 ) ) ;
#22348=ORIENTED_EDGE ( 'NONE', *, *, #65817, .T. ) ;
#22352=CARTESIAN_POINT ( 'NONE',  ( 16.81611548245470189, 1526.382868172864164, 234.5451076435186053 ) ) ;
#22356=CIRCLE ( 'NONE', #38530, 2.000000000000001776 ) ;
#22360=ORIENTED_EDGE ( 'NONE', *, *, #100694, .F. ) ;
#22365=CARTESIAN_POINT ( 'NONE',  ( -29.00779973304124937, 1526.382868172863937, 217.2942086403127178 ) ) ;
#22379=ORIENTED_EDGE ( 'NONE', *, *, #76306, .F. ) ;
#22404=CARTESIAN_POINT ( 'NONE',  ( 21.80961351509229473, 1523.919943579690425, 183.3321359269316986 ) ) ;
#22416=VERTEX_POINT ( 'NONE', #41764 ) ;
#22417=CARTESIAN_POINT ( 'NONE',  ( -16.88555899346171785, 1525.556089352344770, 181.6768889465036523 ) ) ;
#22422=DIRECTION ( 'NONE',  ( 0.4090087482554189968, 0.000000000000000000, 0.9125304618754023211 ) ) ;
#22423=DIRECTION ( 'NONE',  ( 0.000000000000000000, 0.000000000000000000, -1.000000000000000000 ) ) ;
#22426=CARTESIAN_POINT ( 'NONE',  ( 2.372478608332516892, 1522.382868172863937, 243.3440112565233449 ) ) ;
#22429=CARTESIAN_POINT ( 'NONE',  ( -3.246772394788719929, 1511.187213306747708, 241.0944358625217774 ) ) ;
#22453=DIRECTION ( 'NONE',  ( -0.000000000000000000, -1.000000000000000000, -0.000000000000000000 ) ) ;
#22459=CARTESIAN_POINT ( 'NONE',  ( -32.36513277069977335, 1523.847248782568386, 216.1093201122535561 ) ) ;
#22465=ORIENTED_EDGE ( 'NONE', *, *, #71459, .T. ) ;
#22484=CARTESIAN_POINT ( 'NONE',  ( 31.55060375016905638, 1525.712835404586031, 217.0331836276179160 ) ) ;
#22488=CARTESIAN_POINT ( 'NONE',  ( -2.620401159549917480, 1523.382868172864164, 242.1631858340802239 ) ) ;
#22500=ORIENTED_EDGE ( 'NONE', *, *, #65274, .F. ) ;
#22509=CARTESIAN_POINT ( 'NONE',  ( -21.71247731328945108, 1523.982201850120191, 183.5488543797130490 ) ) ;
#22524=CARTESIAN_POINT ( 'NONE',  ( -1.961418762358051238, 1526.143142182166912, 177.8224660300539313 ) ) ;
#22526=ADVANCED_FACE ( 'NONE', ( #104434 ), #64096, .T. ) ;
#22540=CARTESIAN_POINT ( 'NONE',  ( 0.000000000000000000, 1523.051704408389696, 209.1218459616979999 ) ) ;
#22564=CARTESIAN_POINT ( 'NONE',  ( 32.09351624765461253, 1524.374142163904480, 216.7021085575802317 ) ) ;
#22574=CARTESIAN_POINT ( 'NONE',  ( 3.448830483803564828, 1518.913060387330006, 175.1594891075192209 ) ) ;
#22576=CARTESIAN_POINT ( 'NONE',  ( 17.78112617924024264, 1523.954924407802764, 237.8273222678101035 ) ) ;
#22607=CARTESIAN_POINT ( 'NONE',  ( -16.75454338844485846, 1526.382868172571079, 183.6974516591949396 ) ) ;
#22609=ORIENTED_EDGE ( 'NONE', *, *, #93180, .T. ) ;
#22612=CARTESIAN_POINT ( 'NONE',  ( 0.000000000000000000, 1523.382868172864164, 209.1218459616979999 ) ) ;
#22613=CARTESIAN_POINT ( 'NONE',  ( -34.18677586421195258, 1512.187213306747481, 198.4504086008750505 ) ) ;
#22615=CARTESIAN_POINT ( 'NONE',  ( -29.16136750932367150, 1526.143142182265592, 197.5843855542967731 ) ) ;
#22635=B_SPLINE_CURVE_WITH_KNOTS ( 'NONE', 3,
 ( #29480, #89940, #47405, #64779, #99429, #80456 ),
 .UNSPECIFIED., .F., .F.,
 ( 4, 2, 4 ),
 ( -1.131363979617846934E-05, 0.001067788114095997044, 0.002146889867988172572 ),
 .UNSPECIFIED. ) ;
#22663=ADVANCED_FACE ( 'NONE', ( #27598 ), #17315, .F. ) ;
#22667=DIRECTION ( 'NONE',  ( 0.000000000000000000, 0.000000000000000000, 1.000000000000000000 ) ) ;
#22668=CARTESIAN_POINT ( 'NONE',  ( 33.14208818188833305, 1524.841055067849538, 220.4153344904927678 ) ) ;
#22672=ORIENTED_EDGE ( 'NONE', *, *, #74187, .F. ) ;
#22701=CARTESIAN_POINT ( 'NONE',  ( -18.19590854888185305, 1501.977400791986611, 180.0410247165186490 ) ) ;
#22705=ORIENTED_EDGE ( 'NONE', *, *, #75722, .T. ) ;
#22731=EDGE_CURVE ( 'NONE', #6988, #98270, #33034, .T. ) ;
#22745=ORIENTED_EDGE ( 'NONE', *, *, #74314, .F. ) ;
#22749=EDGE_CURVE ( 'NONE', #65751, #103878, #4452, .T. ) ;
#22759=EDGE_CURVE ( 'NONE', #106841, #21883, #69489, .T. ) ;
#22763=CARTESIAN_POINT ( 'NONE',  ( -17.30126322281408235, 1523.382868172864164, 180.8506073313487548 ) ) ;
#22770=CARTESIAN_POINT ( 'NONE',  ( -28.54794148642016793, 1526.382868172864164, 219.8054320333061185 ) ) ;
#22788=CARTESIAN_POINT ( 'NONE',  ( -28.27139721233055170, 1526.382868172863937, 198.6830693683576214 ) ) ;
#22799=AXIS2_PLACEMENT_3D ( 'NONE', #54704, #65301, #88281 ) ;
#22807=ADVANCED_FACE ( 'NONE', ( #53231 ), #26336, .T. ) ;
#22815=DIRECTION ( 'NONE',  ( 0.000000000000000000, 0.000000000000000000, 1.000000000000000000 ) ) ;
#22830=EDGE_CURVE ( 'NONE', #55613, #13824, #77863, .T. ) ;
#22833=CARTESIAN_POINT ( 'NONE',  ( -30.31940284289361998, 1523.456924617336654, 222.4933038711236577 ) ) ;
#22842=CARTESIAN_POINT ( 'NONE',  ( 34.09113935471038559, 1523.429859730330918, 219.7507174562238390 ) ) ;
#22863=( BOUNDED_SURFACE ( )  B_SPLINE_SURFACE ( 3, 2, ( 
 ( #80172, #36516, #54450 ),
 ( #70709, #62300, #88043 ),
 ( #96986, #96427, #19705 ),
 ( #3489, #11327, #37064 ),
 ( #53908, #105381, #28669 ),
 ( #20249, #107017, #82375 ) ),
 .UNSPECIFIED., .F., .F., .F. ) 
 B_SPLINE_SURFACE_WITH_KNOTS ( ( 4, 2, 4 ),
 ( 3, 3 ),
 ( -2.493664996716660198E-17, 0.001312027981647334932, 0.002624055963294695017 ),
 ( 0.000000000000000000, 1.000000000000000000 ),
 .UNSPECIFIED. ) 
 GEOMETRIC_REPRESENTATION_ITEM ( )  RATIONAL_B_SPLINE_SURFACE ( (
 ( 1.000000000000000000, 0.9376006582765856745, 1.000000000000000000),
 ( 1.000000000000000000, 0.9569320108032824956, 1.000000000000000000),
 ( 1.000000000000000000, 0.9725743441605260164, 1.000000000000000000),
 ( 1.000000000000000000, 0.9942095667149332128, 1.000000000000000000),
 ( 1.000000000000000000, 1.000043666449679236, 1.000000000000000000),
 ( 1.000000000000000000, 1.000000000000000000, 1.000000000000000000) ) ) 
 REPRESENTATION_ITEM ( '' )  SURFACE ( )  );
#22864=CARTESIAN_POINT ( 'NONE',  ( 16.68062049856738938, 1526.382868172863937, 236.8314524626094055 ) ) ;
#22868=CARTESIAN_POINT ( 'NONE',  ( -33.42844755915814403, 1522.861859112239472, 222.1271778627171329 ) ) ;
#22874=CARTESIAN_POINT ( 'NONE',  ( 3.448830483803564828, 1512.187213306747481, 175.1594891075192209 ) ) ;
#22877=AXIS2_PLACEMENT_3D ( 'NONE', #50171, #58563, #101080 ) ;
#22882=EDGE_LOOP ( 'NONE', ( #61541, #99537, #105849, #56378, #25799 ) ) ;
#22893=ORIENTED_EDGE ( 'NONE', *, *, #53430, .T. ) ;
#22895=CARTESIAN_POINT ( 'NONE',  ( 16.66231036550724909, 1523.604703353109699, 237.7554842931445762 ) ) ;
#22899=VERTEX_POINT ( 'NONE', #95215 ) ;
#22922=CARTESIAN_POINT ( 'NONE',  ( 2.372478608332517336, 1522.382868172863937, 174.8996806668726549 ) ) ;
#22937=EDGE_CURVE ( 'NONE', #77302, #49611, #89431, .T. ) ;
#22961=DIRECTION ( 'NONE',  ( -1.000000000000000000, 0.000000000000000000, 0.000000000000000000 ) ) ;
#22977=DIRECTION ( 'NONE',  ( 0.000000000000000000, 0.000000000000000000, 1.000000000000000000 ) ) ;
#22982=EDGE_LOOP ( 'NONE', ( #59294, #99332, #54033, #80998, #96099 ) ) ;
#22983=CARTESIAN_POINT ( 'NONE',  ( -16.66231036550740541, 1523.604703353109699, 180.4882076302515372 ) ) ;
#22987=LINE ( 'NONE', #82912, #67887 ) ;
#22990=AXIS2_PLACEMENT_3D ( 'NONE', #7204, #73864, #31289 ) ;
#22997=ORIENTED_EDGE ( 'NONE', *, *, #57868, .T. ) ;
#22999=CARTESIAN_POINT ( 'NONE',  ( 16.65010197087796939, 1526.345556099435726, 183.3431577551421299 ) ) ;
#23045=DIRECTION ( 'NONE',  ( 0.000000000000000000, 1.000000000000000000, 0.000000000000000000 ) ) ;
#23046=VERTEX_POINT ( 'NONE', #32288 ) ;
#23049=CARTESIAN_POINT ( 'NONE',  ( -20.71343476517554905, 1522.382868172863937, 179.9059455038197086 ) ) ;
#23068=VECTOR ( 'NONE', #101011, 1000.000000000000114 ) ;
#23070=EDGE_CURVE ( 'NONE', #35843, #98270, #47249, .T. ) ;
#23078=CARTESIAN_POINT ( 'NONE',  ( -22.69876404239752077, 1522.861859112239017, 181.3483716558110359 ) ) ;
#23126=DIRECTION ( 'NONE',  ( -0.4090087482554316534, 0.000000000000000000, -0.9125304618753966590 ) ) ;
#23133=CARTESIAN_POINT ( 'NONE',  ( -31.32995031131182628, 1523.678648413191695, 221.9013357025048947 ) ) ;
#23138=CARTESIAN_POINT ( 'NONE',  ( -20.07149347155869634, 1526.186458717540972, 185.1794229323607794 ) ) ;
#23142=CIRCLE ( 'NONE', #48195, 0.9999999999999988898 ) ;
#23143=CARTESIAN_POINT ( 'NONE',  ( -21.38516915558007270, 1522.382868172863937, 180.3939891059723664 ) ) ;
#23152=CARTESIAN_POINT ( 'NONE',  ( 17.19754479272649661, 1524.059663615500085, 237.3738432385773365 ) ) ;
#23161=DIRECTION ( 'NONE',  ( -0.2054769195713296304, 0.000000000000000000, 0.9786619618251631847 ) ) ;
#23164=B_SPLINE_CURVE_WITH_KNOTS ( 'NONE', 3,
 ( #23133, #65171, #5247, #75226, #73580, #109378, #57338, #56765, #5814, #39953 ),
 .UNSPECIFIED., .F., .F.,
 ( 4, 2, 2, 2, 4 ),
 ( 0.000000000000000000, 0.0007403986298595417693, 0.001480797259719083539, 0.002221195889578625200, 0.002961594519438167077 ),
 .UNSPECIFIED. ) ;
#23184=ORIENTED_EDGE ( 'NONE', *, *, #41579, .T. ) ;
#23191=AXIS2_PLACEMENT_3D ( 'NONE', #76319, #109921, #110468 ) ;
#23226=ORIENTED_EDGE ( 'NONE', *, *, #41906, .T. ) ;
#23230=DIRECTION ( 'NONE',  ( 0.000000000000000000, 1.000000000000000000, 0.000000000000000000 ) ) ;
#23239=DIRECTION ( 'NONE',  ( 0.000000000000000000, 0.000000000000000000, 1.000000000000000000 ) ) ;
#23244=AXIS2_PLACEMENT_3D ( 'NONE', #11623, #104015, #87223 ) ;
#23262=CARTESIAN_POINT ( 'NONE',  ( -17.37723644544100310, 1525.394081235439444, 237.0493492034528913 ) ) ;
#23269=CARTESIAN_POINT ( 'NONE',  ( 16.55108609117709406, 1524.760046179776054, 180.7894123379967368 ) ) ;
#23280=VERTEX_POINT ( 'NONE', #93821 ) ;
#23299=EDGE_CURVE ( 'NONE', #42516, #31391, #85109, .T. ) ;
#23307=CARTESIAN_POINT ( 'NONE',  ( 1.590879946458802596, 1526.333389947941896, 239.8456008596616016 ) ) ;
#23311=CARTESIAN_POINT ( 'NONE',  ( -2.472529913803023227, 1523.678648413191695, 175.3762130535718597 ) ) ;
#23326=AXIS2_PLACEMENT_3D ( 'NONE', #55307, #88889, #80499 ) ;
#23328=VERTEX_POINT ( 'NONE', #22613 ) ;
#23330=ADVANCED_FACE ( 'NONE', ( #64131 ), #90269, .T. ) ;
#23338=CARTESIAN_POINT ( 'NONE',  ( 30.98826378581297192, 1524.599984580802357, 196.4397214278006345 ) ) ;
#23347=CYLINDRICAL_SURFACE ( 'NONE', #77628, 1.000000000000000444 ) ;
#23360=CARTESIAN_POINT ( 'NONE',  ( -28.81652261710059548, 1526.349684470114653, 198.1982547273859154 ) ) ;
#23382=CIRCLE ( 'NONE', #34100, 1.000000000000000888 ) ;
#23383=CARTESIAN_POINT ( 'NONE',  ( 0.000000000000000000, 1526.382868172863937, 238.6369021217711577 ) ) ;
#23389=DIRECTION ( 'NONE',  ( -4.857225732735055447E-14, 0.000000000000000000, 1.000000000000000000 ) ) ;
#23410=CARTESIAN_POINT ( 'NONE',  ( 30.51231035492520149, 1526.382868172863937, 218.1578534183718432 ) ) ;
#23416=AXIS2_PLACEMENT_3D ( 'NONE', #62578, #96696, #19967 ) ;
#23420=CARTESIAN_POINT ( 'NONE',  ( 2.470168521978398424, 1523.382868172864164, 175.3649660270905315 ) ) ;
#23434=EDGE_CURVE ( 'NONE', #82045, #84088, #8958, .T. ) ;
#23450=CARTESIAN_POINT ( 'NONE',  ( 29.35747451428488830, 1526.382868172571079, 201.0438982057034423 ) ) ;
#23454=EDGE_CURVE ( 'NONE', #39930, #34471, #13733, .T. ) ;
#23455=ORIENTED_EDGE ( 'NONE', *, *, #110441, .F. ) ;
#23469=CARTESIAN_POINT ( 'NONE',  ( 0.000000000000000000, 1511.187213306747708, 209.1218459616979999 ) ) ;
#23470=ORIENTED_EDGE ( 'NONE', *, *, #65180, .F. ) ;
#23486=AXIS2_PLACEMENT_3D ( 'NONE', #6438, #99369, #49557 ) ;
#23518=DIRECTION ( 'NONE',  ( -0.7414773880254760252, 0.000000000000000000, -0.6709778558543624261 ) ) ;
#23520=FACE_OUTER_BOUND ( 'NONE', #22982, .T. ) ;
#23524=EDGE_CURVE ( 'NONE', #63875, #43726, #105333, .T. ) ;
#23533=FACE_OUTER_BOUND ( 'NONE', #30196, .T. ) ;
#23547=CARTESIAN_POINT ( 'NONE',  ( -16.94364159994526986, 1525.231887713386186, 181.3784724611917625 ) ) ;
#23548=DIRECTION ( 'NONE',  ( 0.000000000000000000, 1.000000000000000000, 0.000000000000000000 ) ) ;
#23556=CARTESIAN_POINT ( 'NONE',  ( 32.38601544705583990, 1523.530935881284904, 202.1199691060085968 ) ) ;
#23563=CARTESIAN_POINT ( 'NONE',  ( -2.385013337802742495, 1526.073434386619510, 240.5311849226266645 ) ) ;
#23579=CARTESIAN_POINT ( 'NONE',  ( -30.68434753588525155, 1526.000688113616661, 216.8500914423166819 ) ) ;
#23589=EDGE_CURVE ( 'NONE', #43187, #50508, #63546, .T. ) ;
#23590=ORIENTED_EDGE ( 'NONE', *, *, #32289, .T. ) ;
#23599=TOROIDAL_SURFACE ( 'NONE', #62988, 30.13701971169416538, 3.000000000000000000 ) ;
#23604=DIRECTION ( 'NONE',  ( -0.000000000000000000, -1.000000000000000000, -0.000000000000000000 ) ) ;
#23605=EDGE_LOOP ( 'NONE', ( #46849, #101853, #77887 ) ) ;
#23619=CARTESIAN_POINT ( 'NONE',  ( -30.31940284292426924, 1523.382868172864164, 195.7503880523418616 ) ) ;
#23624=EDGE_CURVE ( 'NONE', #82581, #66323, #108178, .T. ) ;
#23627=VERTEX_POINT ( 'NONE', #102387 ) ;
#23628=TOROIDAL_SURFACE ( 'NONE', #12834, 1.000000000000000000, 1.000000000000000000 ) ;
#23647=DIRECTION ( 'NONE',  ( -0.000000000000000000, -1.000000000000000000, -0.000000000000000000 ) ) ;
#23656=VERTEX_POINT ( 'NONE', #43605 ) ;
#23680=LINE ( 'NONE', #102030, #8961 ) ;
#23688=CARTESIAN_POINT ( 'NONE',  ( 1.770994272916319279, 1526.211528530236592, 240.5584569913896189 ) ) ;
#23694=CARTESIAN_POINT ( 'NONE',  ( 31.75409331310657990, 1525.055402519452173, 216.6568980277143908 ) ) ;
#23695=DIRECTION ( 'NONE',  ( -0.3090169943749403458, 0.000000000000000000, 0.9510565162951560847 ) ) ;
#23711=DIRECTION ( 'NONE',  ( 0.3090169943749582204, 0.000000000000000000, 0.9510565162951499785 ) ) ;
#23718=ORIENTED_EDGE ( 'NONE', *, *, #48220, .F. ) ;
#23737=VERTEX_POINT ( 'NONE', #27341 ) ;
#23769=CYLINDRICAL_SURFACE ( 'NONE', #23486, 1.999999999999991562 ) ;
#23770=CARTESIAN_POINT ( 'NONE',  ( 21.77174004986088462, 1524.860077346005028, 184.6554692728756777 ) ) ;
#23776=EDGE_LOOP ( 'NONE', ( #86067, #83605, #102523, #100752, #19125 ) ) ;
#23787=CARTESIAN_POINT ( 'NONE',  ( -3.348648543330357885, 1523.530935881284904, 176.1572159930114196 ) ) ;
#23788=VERTEX_POINT ( 'NONE', #91107 ) ;
#23814=CARTESIAN_POINT ( 'NONE',  ( 16.48487877296681248, 1525.795403383247276, 181.7735843130006685 ) ) ;
#23834=CARTESIAN_POINT ( 'NONE',  ( -2.682480990172567470, 1524.330813522192102, 241.8675070349543716 ) ) ;
#23854=FACE_OUTER_BOUND ( 'NONE', #90396, .T. ) ;
#23863=CARTESIAN_POINT ( 'NONE',  ( -21.54905603439506478, 1524.816548299036867, 183.6628006193895430 ) ) ;
#23870=( BOUNDED_SURFACE ( )  B_SPLINE_SURFACE ( 3, 2, ( 
 ( #49618, #48520, #5950 ),
 ( #83751, #101085, #99990 ),
 ( #91603, #41205, #65323 ),
 ( #99433, #24383, #6495 ),
 ( #13768, #33334, #75375 ),
 ( #109514, #32790, #83206 ) ),
 .UNSPECIFIED., .F., .F., .F. ) 
 B_SPLINE_SURFACE_WITH_KNOTS ( ( 4, 2, 4 ),
 ( 3, 3 ),
 ( -6.288372600415925717E-17, 0.001312027981647218922, 0.002624055963294500728 ),
 ( 0.000000000000000000, 1.000000000000000000 ),
 .UNSPECIFIED. ) 
 GEOMETRIC_REPRESENTATION_ITEM ( )  RATIONAL_B_SPLINE_SURFACE ( (
 ( 1.000000000000000000, 0.9376006582765932240, 1.000000000000000000),
 ( 1.000000000000000000, 0.9569320108025204386, 1.000000000000000000),
 ( 1.000000000000000000, 0.9725743441615498641, 1.000000000000000000),
 ( 1.000000000000000000, 0.9942095667139038140, 1.000000000000000000),
 ( 1.000000000000000000, 1.000043666450451063, 1.000000000000000000),
 ( 1.000000000000000000, 1.000000000000000000, 1.000000000000000000) ) ) 
 REPRESENTATION_ITEM ( '' )  SURFACE ( )  );
#23875=DIRECTION ( 'NONE',  ( 0.9977304882603014180, 0.06733403890946067227, 0.000000000000000000 ) ) ;
#23877=CARTESIAN_POINT ( 'NONE',  ( -3.448830483803564828, 1512.187213306747481, 175.1594891075192209 ) ) ;
#23879=VERTEX_POINT ( 'NONE', #6555 ) ;
#23888=CIRCLE ( 'NONE', #13261, 2.000000000000001776 ) ;
#23891=CARTESIAN_POINT ( 'NONE',  ( -19.59884465730793579, 1526.382868172863937, 237.0995590530540937 ) ) ;
#23898=DIRECTION ( 'NONE',  ( -0.7414773880254701410, -2.572516463827778023E-15, -0.6709778558543689764 ) ) ;
#23920=DIRECTION ( 'NONE',  ( 0.000000000000000000, -1.000000000000000000, 0.000000000000000000 ) ) ;
#23922=ADVANCED_FACE ( 'NONE', ( #49127 ), #55123, .F. ) ;
#23926=EDGE_CURVE ( 'NONE', #61077, #94335, #97477, .T. ) ;
#23932=DIRECTION ( 'NONE',  ( 0.000000000000000000, 0.000000000000000000, 1.000000000000000000 ) ) ;
#23935=CARTESIAN_POINT ( 'NONE',  ( 20.70484064406403846, 1525.907212628473644, 233.2025904124105580 ) ) ;
#23938=CARTESIAN_POINT ( 'NONE',  ( 17.43739734485520998, 1526.178928173328131, 180.7274168163513082 ) ) ;
#23946=CARTESIAN_POINT ( 'NONE',  ( 34.68852446352672558, 1522.861859112239927, 218.2490599185861697 ) ) ;
#23951=EDGE_CURVE ( 'NONE', #40664, #24247, #39034, .T. ) ;
#23960=CARTESIAN_POINT ( 'NONE',  ( -30.44526109729619989, 1526.211528530236592, 201.0917145515471987 ) ) ;
#23962=CARTESIAN_POINT ( 'NONE',  ( 3.347801439296145709, 1523.456872492435195, 176.1543725841967500 ) ) ;
#23970=CARTESIAN_POINT ( 'NONE',  ( -22.04556278850142093, 1524.082582765195411, 184.4798054120614665 ) ) ;
#23975=EDGE_CURVE ( 'NONE', #38998, #17148, #58164, .T. ) ;
#23997=DIRECTION ( 'NONE',  ( 0.8672669759446726134, -7.800054970605876826E-15, 0.4978433412588572637 ) ) ;
#24012=ORIENTED_EDGE ( 'NONE', *, *, #63496, .T. ) ;
#24037=AXIS2_PLACEMENT_3D ( 'NONE', #96814, #105210, #20085 ) ;
#24039=VERTEX_POINT ( 'NONE', #73518 ) ;
#24060=CARTESIAN_POINT ( 'NONE',  ( 0.000000000000000000, 1512.187213306747481, 209.1218459616979999 ) ) ;
#24070=CARTESIAN_POINT ( 'NONE',  ( -2.686147501205827570, 1526.329757971589515, 176.3936480404082374 ) ) ;
#24113=AXIS2_PLACEMENT_3D ( 'NONE', #69939, #52568, #36853 ) ;
#24139=DIRECTION ( 'NONE',  ( 0.000000000000000000, 0.000000000000000000, -1.000000000000000000 ) ) ;
#24140=ORIENTED_EDGE ( 'NONE', *, *, #67197, .T. ) ;
#24143=ORIENTED_EDGE ( 'NONE', *, *, #78062, .F. ) ;
#24158=ORIENTED_EDGE ( 'NONE', *, *, #83473, .F. ) ;
#24185=CYLINDRICAL_SURFACE ( 'NONE', #58942, 33.13701971169416538 ) ;
#24190=( BOUNDED_SURFACE ( )  B_SPLINE_SURFACE ( 3, 2, ( 
 ( #106107, #29384, #4204 ),
 ( #20424, #63049, #22060 ),
 ( #46228, #80361, #90385 ),
 ( #13664, #47853, #81987 ),
 ( #37805, #22607, #3677 ),
 ( #71451, #107756, #31039 ) ),
 .UNSPECIFIED., .F., .F., .F. ) 
 B_SPLINE_SURFACE_WITH_KNOTS ( ( 4, 2, 4 ),
 ( 3, 3 ),
 ( -2.168404344971008868E-17, 0.001312027981647318452, 0.002624055963294658587 ),
 ( 0.000000000000000000, 1.000000000000000000 ),
 .UNSPECIFIED. ) 
 GEOMETRIC_REPRESENTATION_ITEM ( )  RATIONAL_B_SPLINE_SURFACE ( (
 ( 1.000000000000000000, 0.9376006582765917807, 1.000000000000000000),
 ( 1.000000000000000000, 0.9569320108023516847, 1.000000000000000000),
 ( 1.000000000000000000, 0.9725743441617671348, 1.000000000000000000),
 ( 1.000000000000000000, 0.9942095667136823245, 1.000000000000000000),
 ( 1.000000000000000000, 1.000043666450618485, 1.000000000000000000),
 ( 1.000000000000000000, 1.000000000000000000, 1.000000000000000000) ) ) 
 REPRESENTATION_ITEM ( '' )  SURFACE ( )  );
#24210=CARTESIAN_POINT ( 'NONE',  ( -32.38845792001066570, 1523.456924617338927, 216.1254071227721170 ) ) ;
#24212=EDGE_CURVE ( 'NONE', #25949, #108859, #25989, .T. ) ;
#24225=EDGE_CURVE ( 'NONE', #69831, #20553, #110245, .T. ) ;
#24227=CARTESIAN_POINT ( 'NONE',  ( 34.18677586421187442, 1524.726013923371283, 219.7932833225211482 ) ) ;
#24238=CARTESIAN_POINT ( 'NONE',  ( -18.66420869458074705, 1526.382868172864164, 185.4599087859683095 ) ) ;
#24240=AXIS2_PLACEMENT_3D ( 'NONE', #39423, #96585, #46201 ) ;
#24247=VERTEX_POINT ( 'NONE', #52717 ) ;
#24255=CARTESIAN_POINT ( 'NONE',  ( 17.19739463999655982, 1525.960063244516959, 236.2603809477409698 ) ) ;
#24261=CARTESIAN_POINT ( 'NONE',  ( -18.51436573157398513, 1512.187213306747481, 181.1015051776554969 ) ) ;
#24268=ORIENTED_EDGE ( 'NONE', *, *, #80073, .F. ) ;
#24269=VERTEX_POINT ( 'NONE', #9584 ) ;
#24310=CARTESIAN_POINT ( 'NONE',  ( -0.8350686643532178044, 1524.382868172863937, 240.9330574173806951 ) ) ;
#24316=DIRECTION ( 'NONE',  ( 0.000000000000000000, 1.000000000000000000, 0.000000000000000000 ) ) ;
#24321=DIRECTION ( 'NONE',  ( -0.7414773880254761362, 0.000000000000000000, -0.6709778558543624261 ) ) ;
#24326=CARTESIAN_POINT ( 'NONE',  ( 17.55396644409023210, 1524.816548299036867, 180.7601981288415800 ) ) ;
#24335=( BOUNDED_SURFACE ( )  B_SPLINE_SURFACE ( 3, 2, ( 
 ( #3857, #81614, #29569 ),
 ( #38518, #30675, #39634 ),
 ( #97867, #46409, #72697 ),
 ( #98426, #3303, #13852 ) ),
 .UNSPECIFIED., .F., .F., .F. ) 
 B_SPLINE_SURFACE_WITH_KNOTS ( ( 4, 4 ),
 ( 3, 3 ),
 ( 0.000000000000000000, 0.0002960034161023843515 ),
 ( 0.000000000000000000, 1.000000000000000000 ),
 .UNSPECIFIED. ) 
 GEOMETRIC_REPRESENTATION_ITEM ( )  RATIONAL_B_SPLINE_SURFACE ( (
 ( 1.000000000000000000, 0.8072480644198151145, 1.000000000000000000),
 ( 1.000000000000000000, 0.8072480346917711991, 1.000000000000000000),
 ( 1.000000000000000000, 0.8071723757218373096, 1.000000000000000000),
 ( 1.000000000000000000, 0.8070209408749986491, 1.000000000000000000) ) ) 
 REPRESENTATION_ITEM ( '' )  SURFACE ( )  );
#24360=ORIENTED_EDGE ( 'NONE', *, *, #41288, .F. ) ;
#24383=CARTESIAN_POINT ( 'NONE',  ( -19.34601893677120898, 1526.333389948038530, 233.0427900344768091 ) ) ;
#24421=CARTESIAN_POINT ( 'NONE',  ( 31.23437356469435144, 1512.187213306747481, 197.3468678195113739 ) ) ;
#24444=LINE ( 'NONE', #58632, #77145 ) ;
#24446=ORIENTED_EDGE ( 'NONE', *, *, #89048, .F. ) ;
#24451=CARTESIAN_POINT ( 'NONE',  ( -29.86461515634926656, 1525.960063244517187, 197.2746849027940925 ) ) ;
#24471=UNCERTAINTY_MEASURE_WITH_UNIT (LENGTH_MEASURE( 1.000000000000000082E-05 ), #64675, 'distance_accuracy_value', 'NONE');
#24484=VERTEX_POINT ( 'NONE', #13873 ) ;
#24485=ORIENTED_EDGE ( 'NONE', *, *, #61170, .T. ) ;
#24486=DIRECTION ( 'NONE',  ( -0.1070030146457386366, 0.000000000000000000, -0.9942586961433749204 ) ) ;
#24499=VERTEX_POINT ( 'NONE', #46428 ) ;
#24500=CARTESIAN_POINT ( 'NONE',  ( 33.45065857237933216, 1524.841055067848629, 219.4656524796220367 ) ) ;
#24503=ORIENTED_EDGE ( 'NONE', *, *, #87963, .F. ) ;
#24544=CARTESIAN_POINT ( 'NONE',  ( -2.273033093151270556, 1525.821544997590308, 177.3097463090896326 ) ) ;
#24573=ORIENTED_EDGE ( 'NONE', *, *, #33659, .F. ) ;
#24582=CARTESIAN_POINT ( 'NONE',  ( 30.60461244942475645, 1523.621879633029039, 196.4204177336139878 ) ) ;
#24607=AXIS2_PLACEMENT_3D ( 'NONE', #55384, #12807, #30149 ) ;
#24610=DIRECTION ( 'NONE',  ( -0.9948834766775035421, -0.000000000000000000, -0.1010290445074252669 ) ) ;
#24623=CARTESIAN_POINT ( 'NONE',  ( -17.62867182259884302, 1524.547873515804895, 180.6301120142637728 ) ) ;
#24629=AXIS2_PLACEMENT_3D ( 'NONE', #95063, #27859, #18330 ) ;
#24637=ORIENTED_EDGE ( 'NONE', *, *, #110571, .F. ) ;
#24654=CARTESIAN_POINT ( 'NONE',  ( -30.79916350761092048, 1526.104292489148747, 217.1177548920758795 ) ) ;
#24656=CIRCLE ( 'NONE', #94449, 33.13701971169416538 ) ;
#24658=ORIENTED_EDGE ( 'NONE', *, *, #102990, .F. ) ;
#24671=EDGE_CURVE ( 'NONE', #39549, #22340, #106294, .T. ) ;
#24680=ADVANCED_FACE ( 'NONE', ( #41310 ), #14978, .T. ) ;
#24694=DIRECTION ( 'NONE',  ( 0.000000000000000000, 0.000000000000000000, 1.000000000000000000 ) ) ;
#24707=ORIENTED_EDGE ( 'NONE', *, *, #21296, .T. ) ;
#24710=CARTESIAN_POINT ( 'NONE',  ( 22.08327125186944428, 1523.604703353109699, 233.8169256665487694 ) ) ;
#24716=EDGE_CURVE ( 'NONE', #68013, #24247, #47454, .T. ) ;
#24724=ORIENTED_EDGE ( 'NONE', *, *, #97273, .T. ) ;
#24726=CARTESIAN_POINT ( 'NONE',  ( 32.37018134260406299, 1512.187213306747481, 218.0712926453362002 ) ) ;
#24744=ORIENTED_EDGE ( 'NONE', *, *, #54202, .T. ) ;
#24747=CARTESIAN_POINT ( 'NONE',  ( -32.86470156657983210, 1523.580204110581917, 217.2021180770848616 ) ) ;
#24748=AXIS2_PLACEMENT_3D ( 'NONE', #70060, #71153, #94663 ) ;
#24766=CARTESIAN_POINT ( 'NONE',  ( -30.12442103005642124, 1524.524650307258753, 195.8615354049555322 ) ) ;
#24769=DIRECTION ( 'NONE',  ( 0.4035202328300511176, 0.000000000000000000, 0.9149707217702551798 ) ) ;
#24777=B_SPLINE_CURVE_WITH_KNOTS ( 'NONE', 3,
 ( #18045, #83597, #84153, #75770, #16375, #50573, #34860, #32658, #93104, #85814 ),
 .UNSPECIFIED., .F., .F.,
 ( 4, 2, 2, 2, 4 ),
 ( 0.000000000000000000, 0.0007189769279726063861, 0.001437953855945212772, 0.002156930783917819158, 0.002875907711890425544 ),
 .UNSPECIFIED. ) ;
#24789=CARTESIAN_POINT ( 'NONE',  ( 17.05900707844048014, 1524.678872986498845, 237.1958236346374633 ) ) ;
#24791=LINE ( 'NONE', #76333, #62461 ) ;
#24800=CIRCLE ( 'NONE', #82049, 1.000000000000015099 ) ;
#24802=ORIENTED_EDGE ( 'NONE', *, *, #68911, .F. ) ;
#24819=CARTESIAN_POINT ( 'NONE',  ( -17.17241001986523941, 1523.382868172864164, 179.6185504016046082 ) ) ;
#24852=EDGE_CURVE ( 'NONE', #53780, #73756, #15284, .T. ) ;
#24858=CARTESIAN_POINT ( 'NONE',  ( 1.491506560153233352, 1511.187213306747708, 242.6732489767341576 ) ) ;
#24859=CYLINDRICAL_SURFACE ( 'NONE', #82101, 1.999999999999981348 ) ;
#24862=CARTESIAN_POINT ( 'NONE',  ( -20.91563430996852091, 1525.795403621571268, 233.2509748519915718 ) ) ;
#24882=CARTESIAN_POINT ( 'NONE',  ( -33.52308185467848034, 1525.402221411349728, 217.5800527287189539 ) ) ;
#24883=LINE ( 'NONE', #66942, #91375 ) ;
#24887=CIRCLE ( 'NONE', #33863, 1.000000000000000888 ) ;
#24892=CARTESIAN_POINT ( 'NONE',  ( 19.38211899476434041, 1526.344110814219221, 185.3185741806024112 ) ) ;
#24893=DIRECTION ( 'NONE',  ( -0.000000000000000000, -1.000000000000000000, -0.000000000000000000 ) ) ;
#24904=CARTESIAN_POINT ( 'NONE',  ( 16.66231036550703593, 1523.604703353109699, 180.4882076302513099 ) ) ;
#24938=DIRECTION ( 'NONE',  ( 0.2113515706023409990, -1.466546124833963756E-15, 0.9774101051267701790 ) ) ;
#24956=ADVANCED_FACE ( 'NONE', ( #77669 ), #83100, .T. ) ;
#24970=CARTESIAN_POINT ( 'NONE',  ( -0.4151546846821903003, 1512.187213306747481, 173.3106345060153046 ) ) ;
#24974=CARTESIAN_POINT ( 'NONE',  ( -33.28034951413921760, 1512.187213306747481, 217.4407153818824838 ) ) ;
#24981=CARTESIAN_POINT ( 'NONE',  ( 1.491506560153238015, 1511.187213306747708, 175.5704429466618421 ) ) ;
#24984=ADVANCED_FACE ( 'NONE', ( #12669 ), #13192, .T. ) ;
#24998=CARTESIAN_POINT ( 'NONE',  ( -3.059311260596259352, 1525.343710797494396, 241.3958505225228066 ) ) ;
#25013=ORIENTED_EDGE ( 'NONE', *, *, #47009, .F. ) ;
#25019=CARTESIAN_POINT ( 'NONE',  ( 3.355802132529028370, 1523.843271061949054, 176.1812215589180539 ) ) ;
#25031=CARTESIAN_POINT ( 'NONE',  ( 33.42844755917195698, 1501.977400791986611, 222.1271778627166213 ) ) ;
#25033=ORIENTED_EDGE ( 'NONE', *, *, #94906, .F. ) ;
#25040=DIRECTION ( 'NONE',  ( -0.7414773880254689198, 0.000000000000000000, 0.6709778558543705307 ) ) ;
#25058=FACE_OUTER_BOUND ( 'NONE', #67611, .T. ) ;
#25062=CARTESIAN_POINT ( 'NONE',  ( -22.08523867432794674, 1523.530870145311610, 233.8225105631221084 ) ) ;
#25069=VECTOR ( 'NONE', #105572, 1000.000000000000114 ) ;
#25076=DIRECTION ( 'NONE',  ( -0.000000000000000000, -1.000000000000000000, -0.000000000000000000 ) ) ;
#25094=DIRECTION ( 'NONE',  ( 0.000000000000000000, 0.000000000000000000, 1.000000000000000000 ) ) ;
#25098=EDGE_CURVE ( 'NONE', #5750, #64661, #93940, .T. ) ;
#25100=CARTESIAN_POINT ( 'NONE',  ( -2.340423001224519517, 1525.425686270222059, 176.3541592074136872 ) ) ;
#25103=VECTOR ( 'NONE', #67057, 1000.000000000000000 ) ;
#25114=ORIENTED_EDGE ( 'NONE', *, *, #39849, .F. ) ;
#25118=CARTESIAN_POINT ( 'NONE',  ( 29.30029655192931770, 1525.907212628473872, 221.3719603026171114 ) ) ;
#25141=CARTESIAN_POINT ( 'NONE',  ( 30.31052258194585036, 1523.604703353109926, 195.7506062427367794 ) ) ;
#25142=CARTESIAN_POINT ( 'NONE',  ( 28.54400548274967520, 1526.382868172863482, 219.8019517411713082 ) ) ;
#25143=CARTESIAN_POINT ( 'NONE',  ( -16.55212241054000089, 1524.756004293092019, 180.7964624130805191 ) ) ;
#25145=CARTESIAN_POINT ( 'NONE',  ( 2.389876875773846887, 1525.253972588464876, 242.0501992864865883 ) ) ;
#25152=( BOUNDED_SURFACE ( )  B_SPLINE_SURFACE ( 3, 2, ( 
 ( #39187, #3422, #22922 ),
 ( #48169, #31343, #47067 ),
 ( #47609, #29692, #21814 ),
 ( #63337, #55470, #89597 ),
 ( #20725, #4508, #80102 ),
 ( #71753, #81191, #63876 ),
 ( #3974, #56013, #38098 ),
 ( #13420, #12889, #72275 ),
 ( #11799, #73918, #29150 ),
 ( #38641, #72817, #54921 ) ),
 .UNSPECIFIED., .F., .F., .F. ) 
 B_SPLINE_SURFACE_WITH_KNOTS ( ( 4, 2, 2, 2, 4 ),
 ( 3, 3 ),
 ( 0.000000000000000000, 0.3926990816987241395, 0.7853981633974482790, 1.178097245096172418, 1.570796326794896558 ),
 ( 0.000000000000000000, 1.000000000000000000 ),
 .UNSPECIFIED. ) 
 GEOMETRIC_REPRESENTATION_ITEM ( )  RATIONAL_B_SPLINE_SURFACE ( (
 ( 1.000000000000000000, 0.7763623250684303922, 1.000000000000000000),
 ( 1.000000000000000000, 0.7763684247035209651, 1.000000000000000000),
 ( 1.000000000000000000, 0.7746454561797311289, 1.000000000000000000),
 ( 1.000000000000000000, 0.7679730451973156846, 1.000000000000000000),
 ( 1.000000000000000000, 0.7630177051950561840, 1.000000000000000000),
 ( 1.000000000000000000, 0.7504512394524429642, 1.000000000000000000),
 ( 1.000000000000000000, 0.7428408967926065642, 1.000000000000000000),
 ( 1.000000000000000000, 0.7259222650911398844, 1.000000000000000000),
 ( 1.000000000000000000, 0.7166207884818885931, 1.000000000000000000),
 ( 1.000000000000000000, 0.7071067811865857644, 1.000000000000000000) ) ) 
 REPRESENTATION_ITEM ( '' )  SURFACE ( )  );
#25178=DIRECTION ( 'NONE',  ( -0.000000000000000000, -1.000000000000000000, -0.000000000000000000 ) ) ;
#25179=ORIENTED_EDGE ( 'NONE', *, *, #37977, .T. ) ;
#25181=AXIS2_PLACEMENT_3D ( 'NONE', #2910, #37028, #62839 ) ;
#25182=CARTESIAN_POINT ( 'NONE',  ( 33.23571934791666393, 1512.187213306747481, 198.7594255952494677 ) ) ;
#25188=DIRECTION ( 'NONE',  ( 0.000000000000000000, 0.000000000000000000, 1.000000000000000000 ) ) ;
#25208=CARTESIAN_POINT ( 'NONE',  ( 32.86802468386292730, 1512.187213306747481, 217.2040256693915410 ) ) ;
#25209=FACE_OUTER_BOUND ( 'NONE', #56483, .T. ) ;
#25225=EDGE_CURVE ( 'NONE', #88502, #39623, #61785, .T. ) ;
#25240=ORIENTED_EDGE ( 'NONE', *, *, #30975, .T. ) ;
#25263=VECTOR ( 'NONE', #76389, 1000.000000000000000 ) ;
#25284=CARTESIAN_POINT ( 'NONE',  ( -21.66432897272838431, 1525.042412244734578, 233.5340606467491966 ) ) ;
#25307=ADVANCED_FACE ( 'NONE', ( #85364 ), #94891, .T. ) ;
#25308=DIRECTION ( 'NONE',  ( 0.000000000000000000, 1.000000000000000000, 0.000000000000000000 ) ) ;
#25315=EDGE_CURVE ( 'NONE', #54321, #73940, #93225, .T. ) ;
#25325=CARTESIAN_POINT ( 'NONE',  ( -30.04653961080366287, 1524.739915903616748, 195.9294070843147892 ) ) ;
#25355=CARTESIAN_POINT ( 'NONE',  ( 31.34137657934019927, 1512.187213306747481, 221.9025654077410081 ) ) ;
#25365=ORIENTED_EDGE ( 'NONE', *, *, #45891, .F. ) ;
#25376=ADVANCED_FACE ( 'NONE', ( #61328 ), #50681, .F. ) ;
#25377=CARTESIAN_POINT ( 'NONE',  ( 0.4151546846821903003, 1511.187213306747708, 174.3106345060153046 ) ) ;
#25381=ORIENTED_EDGE ( 'NONE', *, *, #46840, .F. ) ;
#25396=EDGE_LOOP ( 'NONE', ( #10828, #80506, #11636, #28296 ) ) ;
#25402=ORIENTED_EDGE ( 'NONE', *, *, #84660, .T. ) ;
#25407=CARTESIAN_POINT ( 'NONE',  ( 21.71247731329033215, 1523.982201850120191, 183.5488543797099226 ) ) ;
#25414=CARTESIAN_POINT ( 'NONE',  ( -20.70484064406366187, 1525.907212628473644, 233.2025904124108706 ) ) ;
#25416=CARTESIAN_POINT ( 'NONE',  ( 30.31052258194597471, 1523.604703353109699, 222.4930856806589929 ) ) ;
#25434=EDGE_CURVE ( 'NONE', #87976, #12155, #8177, .T. ) ;
#25436=AXIS2_PLACEMENT_3D ( 'NONE', #13719, #82612, #14284 ) ;
#25451=CARTESIAN_POINT ( 'NONE',  ( -20.53760542139810852, 1525.821544997590308, 184.7213720461156470 ) ) ;
#25461=CARTESIAN_POINT ( 'NONE',  ( 33.42844755916640764, 1522.861859112239927, 196.1165140606936745 ) ) ;
#25464=CARTESIAN_POINT ( 'NONE',  ( 16.51111913633373263, 1525.159196711359755, 181.0518213589280947 ) ) ;
#25528=CARTESIAN_POINT ( 'NONE',  ( -19.53786426059057746, 1511.187213306747708, 181.5239794925695946 ) ) ;
#25543=CARTESIAN_POINT ( 'NONE',  ( -29.41653895341162439, 1525.790286462514587, 221.5659762852381505 ) ) ;
#25550=CARTESIAN_POINT ( 'NONE',  ( 21.54116136303161966, 1523.462669333490112, 234.3126182784851039 ) ) ;
#25556=CARTESIAN_POINT ( 'NONE',  ( -17.44952998132148281, 1525.163457223743990, 237.2403228777125150 ) ) ;
#25557=EDGE_CURVE ( 'NONE', #12956, #58921, #88443, .T. ) ;
#25560=DIRECTION ( 'NONE',  ( -0.000000000000000000, -1.000000000000000000, -0.000000000000000000 ) ) ;
#25565=ORIENTED_EDGE ( 'NONE', *, *, #46890, .T. ) ;
#25568=ORIENTED_EDGE ( 'NONE', *, *, #82556, .F. ) ;
#25570=CARTESIAN_POINT ( 'NONE',  ( -31.32995031131182628, 1523.678648413191695, 221.9013357025048947 ) ) ;
#25571=CARTESIAN_POINT ( 'NONE',  ( 2.485125933802709852, 1524.547873515805350, 175.7096756841900458 ) ) ;
#25584=CARTESIAN_POINT ( 'NONE',  ( 2.582675909241441747, 1526.178928173327677, 242.3428666835334298 ) ) ;
#25608=ORIENTED_EDGE ( 'NONE', *, *, #41875, .T. ) ;
#25609=DIRECTION ( 'NONE',  ( 0.000000000000000000, 1.000000000000000000, 0.000000000000000000 ) ) ;
#25693=CARTESIAN_POINT ( 'NONE',  ( 30.57065064345538374, 1523.844782250838307, 196.3873375281003177 ) ) ;
#25698=ORIENTED_EDGE ( 'NONE', *, *, #65850, .T. ) ;
#25699=CARTESIAN_POINT ( 'NONE',  ( -1.484142863822457858, 1526.349689584397083, 178.3401621312602572 ) ) ;
#25721=VECTOR ( 'NONE', #39896, 1000.000000000000227 ) ;
#25743=CARTESIAN_POINT ( 'NONE',  ( -16.65100080374379843, 1526.335487865669393, 183.3462803417096723 ) ) ;
#25748=DIRECTION ( 'NONE',  ( 0.000000000000000000, 1.000000000000000000, 0.000000000000000000 ) ) ;
#25753=CARTESIAN_POINT ( 'NONE',  ( -20.71343476517490600, 1522.382868172863937, 238.3377464195766606 ) ) ;
#25772=CARTESIAN_POINT ( 'NONE',  ( -29.00779973304124582, 1526.382868172864164, 217.2942086403127178 ) ) ;
#25788=DIRECTION ( 'NONE',  ( 0.000000000000000000, 0.000000000000000000, -1.000000000000000000 ) ) ;
#25798=ORIENTED_EDGE ( 'NONE', *, *, #63819, .F. ) ;
#25799=ORIENTED_EDGE ( 'NONE', *, *, #78172, .F. ) ;
#25803=CARTESIAN_POINT ( 'NONE',  ( 18.69816095120771493, 1526.382868172863937, 234.8576566410002897 ) ) ;
#25806=DIRECTION ( 'NONE',  ( 0.000000000000000000, 1.000000000000000000, 0.000000000000000000 ) ) ;
#25836=DIRECTION ( 'NONE',  ( 0.8672669759446665072, 0.000000000000000000, 0.4978433412588676998 ) ) ;
#25839=CARTESIAN_POINT ( 'NONE',  ( -20.79738390328697406, 1511.187213306747708, 237.0406858230491025 ) ) ;
#25854=DIRECTION ( 'NONE',  ( -0.000000000000000000, -1.000000000000000000, -0.000000000000000000 ) ) ;
#25862=CARTESIAN_POINT ( 'NONE',  ( 17.19739463999647100, 1525.960063244516959, 236.2603809477409982 ) ) ;
#25885=CIRCLE ( 'NONE', #7996, 1.000000000000000888 ) ;
#25896=CARTESIAN_POINT ( 'NONE',  ( 22.75273496409596774, 1523.382868172864164, 234.5707981297186109 ) ) ;
#25898=CARTESIAN_POINT ( 'NONE',  ( 16.52275697107005570, 1525.042337199239910, 180.9739969239476522 ) ) ;
#25903=FACE_OUTER_BOUND ( 'NONE', #94931, .T. ) ;
#25918=CARTESIAN_POINT ( 'NONE',  ( 21.55808852498703843, 1523.844789899191710, 183.9826104398626967 ) ) ;
#25922=CARTESIAN_POINT ( 'NONE',  ( 21.12212911287011963, 1512.187213306747481, 182.4210318429774134 ) ) ;
#25929=CARTESIAN_POINT ( 'NONE',  ( -32.86802468386279941, 1523.382868172864164, 217.2040256693919957 ) ) ;
#25949=VERTEX_POINT ( 'NONE', #108815 ) ;
#25967=CARTESIAN_POINT ( 'NONE',  ( 22.07680818022633318, 1523.847248782568613, 184.4451128950378518 ) ) ;
#25971=CARTESIAN_POINT ( 'NONE',  ( 30.30249668296529464, 1524.678872986498618, 221.8071382193505201 ) ) ;
#25988=CARTESIAN_POINT ( 'NONE',  ( 29.30029655192942073, 1525.907212628473644, 196.8717316207784620 ) ) ;
#25989=CIRCLE ( 'NONE', #13439, 30.10786454236638576 ) ;
#25999=DIRECTION ( 'NONE',  ( -0.9510565162951566398, 0.000000000000000000, -0.3090169943749382919 ) ) ;
#26000=DIRECTION ( 'NONE',  ( 0.7414773880254711402, 0.000000000000000000, 0.6709778558543678662 ) ) ;
#26001=CIRCLE ( 'NONE', #29615, 1.000000000000000444 ) ;
#26004=CARTESIAN_POINT ( 'NONE',  ( 19.54391504031716664, 1526.306647125542895, 185.2858915736553911 ) ) ;
#26006=CARTESIAN_POINT ( 'NONE',  ( -21.84020450222019250, 1512.187213306747481, 234.9798068779743403 ) ) ;
#26022=CARTESIAN_POINT ( 'NONE',  ( 30.31643683089982844, 1523.530935881284904, 195.7504610701754189 ) ) ;
#26026=CYLINDRICAL_SURFACE ( 'NONE', #5183, 0.9999999999999906741 ) ;
#26040=DIRECTION ( 'NONE',  ( 0.9510565162951518658, 0.000000000000000000, -0.3090169943749528914 ) ) ;
#26047=CARTESIAN_POINT ( 'NONE',  ( 17.17241001986483795, 1512.187213306747481, 181.6185504016043240 ) ) ;
#26049=CARTESIAN_POINT ( 'NONE',  ( -32.18358323225091766, 1524.059547553519224, 201.4963293957178792 ) ) ;
#26051=CARTESIAN_POINT ( 'NONE',  ( -21.41971086555067316, 1512.187213306747481, 233.0798096144383749 ) ) ;
#26062=VERTEX_POINT ( 'NONE', #37626 ) ;
#26074=DIRECTION ( 'NONE',  ( 0.000000000000000000, -0.8286769424886414326, -0.5597271880011518430 ) ) ;
#26080=EDGE_CURVE ( 'NONE', #18078, #8168, #44014, .T. ) ;
#26107=EDGE_CURVE ( 'NONE', #109511, #40850, #74151, .T. ) ;
#26123=PRODUCT_DEFINITION_FORMATION_WITH_SPECIFIED_SOURCE ( 'ANY', '', #82225, .NOT_KNOWN. ) ;
#26125=CARTESIAN_POINT ( 'NONE',  ( 2.596261494520262225, 1525.907212628473644, 177.4701144822247727 ) ) ;
#26132=DIRECTION ( 'NONE',  ( 0.9125304618753908859, 0.000000000000000000, -0.4090087482554448095 ) ) ;
#26165=CARTESIAN_POINT ( 'NONE',  ( -31.32995031131208918, 1523.678648413191695, 196.3423562208917872 ) ) ;
#26210=CARTESIAN_POINT ( 'NONE',  ( -3.317974621678423830, 1524.412455883367784, 176.3320022186326241 ) ) ;
#26217=CYLINDRICAL_SURFACE ( 'NONE', #7825, 2.000000000000000000 ) ;
#26227=EDGE_CURVE ( 'NONE', #26062, #36172, #29360, .T. ) ;
#26231=EDGE_CURVE ( 'NONE', #81018, #4524, #90423, .T. ) ;
#26237=CARTESIAN_POINT ( 'NONE',  ( 20.71343476517513338, 1522.382868172863937, 179.9059455038194528 ) ) ;
#26239=ORIENTED_EDGE ( 'NONE', *, *, #55441, .F. ) ;
#26255=DIRECTION ( 'NONE',  ( 0.9942586961433745874, 0.000000000000000000, -0.1070030146457423004 ) ) ;
#26272=AXIS2_PLACEMENT_3D ( 'NONE', #99388, #5905, #93202 ) ;
#26282=VECTOR ( 'NONE', #49750, 1000.000000000000000 ) ;
#26292=ORIENTED_EDGE ( 'NONE', *, *, #89173, .F. ) ;
#26296=CARTESIAN_POINT ( 'NONE',  ( -31.80535162409287864, 1525.137906803776332, 216.1511969346493345 ) ) ;
#26306=DIRECTION ( 'NONE',  ( 0.000000000000000000, 0.000000000000000000, 1.000000000000000000 ) ) ;
#26321=CARTESIAN_POINT ( 'NONE',  ( -2.038847259689231084, 1501.977400791986611, 173.3106345060153046 ) ) ;
#26328=CARTESIAN_POINT ( 'NONE',  ( -29.41145195048104455, 1525.795403383247276, 221.5574857735277874 ) ) ;
#26335=ORIENTED_EDGE ( 'NONE', *, *, #70675, .F. ) ;
#26336=PLANE ( 'NONE',  #34891 ) ;
#26361=DIRECTION ( 'NONE',  ( 0.6709778558543747495, 0.000000000000000000, 0.7414773880254650340 ) ) ;
#26365=LINE ( 'NONE', #25803, #102813 ) ;
#26398=ADVANCED_FACE ( 'NONE', ( #749 ), #101703, .F. ) ;
#26402=CARTESIAN_POINT ( 'NONE',  ( -20.64339891394635629, 1523.429859730330236, 179.9837476533126335 ) ) ;
#26404=EDGE_CURVE ( 'NONE', #36172, #42124, #101869, .T. ) ;
#26418=CIRCLE ( 'NONE', #22799, 1.000000000000000888 ) ;
#26434=ORIENTED_EDGE ( 'NONE', *, *, #88708, .T. ) ;
#26437=AXIS2_PLACEMENT_3D ( 'NONE', #44370, #46030, #80158 ) ;
#26448=AXIS2_PLACEMENT_3D ( 'NONE', #21352, #62321, #55559 ) ;
#26459=CARTESIAN_POINT ( 'NONE',  ( 17.83486663330484845, 1523.678648413191922, 180.3677388339000061 ) ) ;
#26480=CARTESIAN_POINT ( 'NONE',  ( 20.49599333844850335, 1525.960063244516959, 184.3798832129034793 ) ) ;
#26481=ORIENTED_EDGE ( 'NONE', *, *, #16455, .F. ) ;
#26484=DIRECTION ( 'NONE',  ( 0.3090169943749447867, 0.000000000000000000, -0.9510565162951545304 ) ) ;
#26485=( BOUNDED_SURFACE ( )  B_SPLINE_SURFACE ( 3, 2, ( 
 ( #4848, #57491, #80473 ),
 ( #38453, #46891, #12707 ),
 ( #106218, #14892, #81547 ),
 ( #74289, #3791, #29500 ),
 ( #55839, #39566, #65886 ),
 ( #37922, #107316, #4322 ),
 ( #72625, #63694, #73739 ),
 ( #47424, #30611, #89417 ),
 ( #38995, #106757, #30047 ),
 ( #64239, #13235, #73172 ) ),
 .UNSPECIFIED., .F., .F., .F. ) 
 B_SPLINE_SURFACE_WITH_KNOTS ( ( 4, 2, 2, 2, 4 ),
 ( 3, 3 ),
 ( 0.000000000000000000, 0.3926990816987241395, 0.7853981633974482790, 1.178097245096172418, 1.570796326794896558 ),
 ( 0.000000000000000000, 1.000000000000000000 ),
 .UNSPECIFIED. ) 
 GEOMETRIC_REPRESENTATION_ITEM ( )  RATIONAL_B_SPLINE_SURFACE ( (
 ( 1.000000000000000000, 0.7763623250684333899, 1.000000000000000000),
 ( 1.000000000000000000, 0.7763684247036575226, 1.000000000000000000),
 ( 1.000000000000000000, 0.7746454561795425020, 1.000000000000000000),
 ( 1.000000000000000000, 0.7679730451975060879, 1.000000000000000000),
 ( 1.000000000000000000, 0.7630177051941748889, 1.000000000000000000),
 ( 1.000000000000000000, 0.7504512394533247033, 1.000000000000000000),
 ( 1.000000000000000000, 0.7428408967923679773, 1.000000000000000000),
 ( 1.000000000000000000, 0.7259222650913751407, 1.000000000000000000),
 ( 1.000000000000000000, 0.7166207884817078488, 1.000000000000000000),
 ( 1.000000000000000000, 0.7071067811865879849, 1.000000000000000000) ) ) 
 REPRESENTATION_ITEM ( '' )  SURFACE ( )  );
#26505=VECTOR ( 'NONE', #77432, 1000.000000000000114 ) ;
#26519=EDGE_LOOP ( 'NONE', ( #94952, #77603, #101815, #78457 ) ) ;
#26528=AXIS2_PLACEMENT_3D ( 'NONE', #3038, #43907, #53998 ) ;
#26537=DIRECTION ( 'NONE',  ( -0.7414773880254735827, -0.000000000000000000, -0.6709778558543652016 ) ) ;
#26539=CARTESIAN_POINT ( 'NONE',  ( 30.17514886432845955, 1525.712830164893376, 221.2664250985396848 ) ) ;
#26549=DIRECTION ( 'NONE',  ( -0.9510565162951561957, 0.000000000000000000, -0.3090169943749392911 ) ) ;
#26569=PLANE ( 'NONE',  #94824 ) ;
#26578=CARTESIAN_POINT ( 'NONE',  ( 31.81407709659792715, 1522.644714754857659, 196.2902540610638198 ) ) ;
#26600=AXIS2_PLACEMENT_3D ( 'NONE', #110757, #104010, #95617 ) ;
#26611=VECTOR ( 'NONE', #8910, 999.9999999999998863 ) ;
#26618=CARTESIAN_POINT ( 'NONE',  ( -31.31962774233543101, 1525.556090473913400, 201.5436825240319365 ) ) ;
#26632=CARTESIAN_POINT ( 'NONE',  ( 0.000000000000000000, 1522.051704408389924, 232.8211094035767985 ) ) ;
#26642=DIRECTION ( 'NONE',  ( -0.000000000000000000, -1.000000000000000000, -0.000000000000000000 ) ) ;
#26673=LINE ( 'NONE', #60301, #102339 ) ;
#26690=CARTESIAN_POINT ( 'NONE',  ( -32.59719044532482002, 1523.982201850120191, 201.1951351303495414 ) ) ;
#26699=DIRECTION ( 'NONE',  ( 0.000000000000000000, 0.000000000000000000, -1.000000000000000000 ) ) ;
#26706=DIRECTION ( 'NONE',  ( 0.000000000000000000, 0.000000000000000000, -1.000000000000000000 ) ) ;
#26721=ORIENTED_EDGE ( 'NONE', *, *, #107775, .T. ) ;
#26732=CYLINDRICAL_SURFACE ( 'NONE', #37261, 1.000000000000000888 ) ;
#26764=CIRCLE ( 'NONE', #53657, 1.000000000000003775 ) ;
#26773=CIRCLE ( 'NONE', #85758, 0.9999999999999987788 ) ;
#26777=CARTESIAN_POINT ( 'NONE',  ( -2.410659749415533071, 1525.163457223744217, 176.1169438982480244 ) ) ;
#26807=ORIENTED_EDGE ( 'NONE', *, *, #78822, .F. ) ;
#26818=CARTESIAN_POINT ( 'NONE',  ( 30.41976661596575937, 1524.374142163904025, 196.3903116790124841 ) ) ;
#26829=CARTESIAN_POINT ( 'NONE',  ( -22.74803453391424668, 1523.678648413191695, 234.5603111028700027 ) ) ;
#26874=EDGE_CURVE ( 'NONE', #67163, #44154, #20474, .T. ) ;
#26883=ORIENTED_EDGE ( 'NONE', *, *, #87069, .T. ) ;
#26884=EDGE_CURVE ( 'NONE', #58330, #104688, #97383, .T. ) ;
#26895=CARTESIAN_POINT ( 'NONE',  ( -33.14208818188965466, 1524.841055067850448, 220.4153344904860887 ) ) ;
#26912=CARTESIAN_POINT ( 'NONE',  ( 20.92767404034517753, 1511.187213306747708, 235.3888156262294444 ) ) ;
#26929=ORIENTED_EDGE ( 'NONE', *, *, #37738, .T. ) ;
#26937=DIRECTION ( 'NONE',  ( 0.000000000000000000, 0.000000000000000000, -1.000000000000000000 ) ) ;
#26939=CARTESIAN_POINT ( 'NONE',  ( 18.02257621027597523, 1524.382868172863937, 235.3484976865586589 ) ) ;
#26951=FACE_OUTER_BOUND ( 'NONE', #26519, .T. ) ;
#26954=CIRCLE ( 'NONE', #80829, 2.000000000000001776 ) ;
#26955=CARTESIAN_POINT ( 'NONE',  ( -31.81407709660760830, 1522.382868172863937, 221.9534378623334590 ) ) ;
#26959=CARTESIAN_POINT ( 'NONE',  ( 0.4151546846821905223, 1524.726013923371283, 173.3106345060153330 ) ) ;
#26967=AXIS2_PLACEMENT_3D ( 'NONE', #47501, #64316, #72707 ) ;
#26971=CARTESIAN_POINT ( 'NONE',  ( 28.27139721233038827, 1526.382868172863937, 198.6830693683571667 ) ) ;
#26972=DIRECTION ( 'NONE',  ( 0.000000000000000000, 0.000000000000000000, 1.000000000000000000 ) ) ;
#26973=B_SPLINE_CURVE_WITH_KNOTS ( 'NONE', 3,
 ( #47806, #66830, #23688, #99840, #56763, #13618 ),
 .UNSPECIFIED., .F., .F.,
 ( 4, 2, 4 ),
 ( 2.841188977517477842E-17, 0.001087661325621714888, 0.002175322651243401587 ),
 .UNSPECIFIED. ) ;
#26997=CARTESIAN_POINT ( 'NONE',  ( 17.55387852034876772, 1524.816846803860926, 237.4833057087513168 ) ) ;
#27002=EDGE_CURVE ( 'NONE', #47989, #52269, #38458, .T. ) ;
#27036=CYLINDRICAL_SURFACE ( 'NONE', #94381, 1.000000000000000888 ) ;
#27045=CONICAL_SURFACE ( 'NONE', #48556, 23.69926344187880929, 1.195358426993359036 ) ;
#27051=EDGE_CURVE ( 'NONE', #83952, #89419, #54596, .T. ) ;
#27058=CARTESIAN_POINT ( 'NONE',  ( 21.60819468828557177, 1524.659802833171625, 183.5975935901099376 ) ) ;
#27062=CARTESIAN_POINT ( 'NONE',  ( -2.372478608332516892, 1512.187213306747481, 243.3440112565233449 ) ) ;
#27067=CIRCLE ( 'NONE', #86114, 1.000000000000001554 ) ;
#27074=AXIS2_PLACEMENT_3D ( 'NONE', #41455, #109752, #67220 ) ;
#27079=ORIENTED_EDGE ( 'NONE', *, *, #24852, .T. ) ;
#27080=ORIENTED_EDGE ( 'NONE', *, *, #76982, .F. ) ;
#27096=EDGE_LOOP ( 'NONE', ( #38338, #109305, #17682, #47306 ) ) ;
#27113=CIRCLE ( 'NONE', #84324, 2.000000000000001332 ) ;
#27130=CARTESIAN_POINT ( 'NONE',  ( -18.66420869458074350, 1526.382868172863937, 185.4599087859683095 ) ) ;
#27135=CIRCLE ( 'NONE', #43207, 1.000000000000011102 ) ;
#27138=FACE_OUTER_BOUND ( 'NONE', #80085, .T. ) ;
#27141=CARTESIAN_POINT ( 'NONE',  ( -32.02808312589930040, 1501.977400791986611, 198.2787714533499752 ) ) ;
#27165=DIRECTION ( 'NONE',  ( -0.8672669759446667292, 0.000000000000000000, -0.4978433412588673113 ) ) ;
#27179=ORIENTED_EDGE ( 'NONE', *, *, #6907, .F. ) ;
#27185=ADVANCED_FACE ( 'NONE', ( #106509 ), #74572, .T. ) ;
#27211=CARTESIAN_POINT ( 'NONE',  ( 31.12456774391177206, 1525.960063244516959, 217.0912716842394730 ) ) ;
#27218=DIRECTION ( 'NONE',  ( -0.000000000000000000, -1.000000000000000000, -0.000000000000000000 ) ) ;
#27233=ORIENTED_EDGE ( 'NONE', *, *, #68470, .T. ) ;
#27246=ORIENTED_EDGE ( 'NONE', *, *, #5587, .F. ) ;
#27254=CARTESIAN_POINT ( 'NONE',  ( -30.31052258194604576, 1523.604703353109699, 195.7506062427372058 ) ) ;
#27263=CARTESIAN_POINT ( 'NONE',  ( 0.8350686643532179154, 1526.382868172863937, 240.9330574173806951 ) ) ;
#27284=ORIENTED_EDGE ( 'NONE', *, *, #14136, .F. ) ;
#27290=DIRECTION ( 'NONE',  ( 0.6665120492724535550, 0.000000000000000000, -0.7454942576402816545 ) ) ;
#27303=ORIENTED_EDGE ( 'NONE', *, *, #65857, .F. ) ;
#27320=ORIENTED_EDGE ( 'NONE', *, *, #11684, .F. ) ;
#27327=CARTESIAN_POINT ( 'NONE',  ( -2.472529913803048984, 1523.678648413191922, 175.3762130535718597 ) ) ;
#27339=ORIENTED_EDGE ( 'NONE', *, *, #77699, .T. ) ;
#27341=CARTESIAN_POINT ( 'NONE',  ( -32.02808312589930040, 1512.187213306747481, 196.2787714533499752 ) ) ;
#27349=EDGE_CURVE ( 'NONE', #98891, #42640, #621, .T. ) ;
#27353=ORIENTED_EDGE ( 'NONE', *, *, #105647, .T. ) ;
#27374=DIRECTION ( 'NONE',  ( 0.5117323852941357831, -0.8591449038673127925, 0.000000000000000000 ) ) ;
#27378=CARTESIAN_POINT ( 'NONE',  ( 21.19880661589024839, 1524.382868172863937, 233.5487980989310302 ) ) ;
#27395=CARTESIAN_POINT ( 'NONE',  ( 29.99620953741496976, 1526.382868172863937, 219.7462484079458704 ) ) ;
#27411=ORIENTED_EDGE ( 'NONE', *, *, #63941, .F. ) ;
#27414=DIRECTION ( 'NONE',  ( 0.000000000000000000, 1.000000000000000000, 0.000000000000000000 ) ) ;
#27432=B_SPLINE_CURVE_WITH_KNOTS ( 'NONE', 3,
 ( #31764, #109588, #32858, #58639, #16048, #67598, #91674, #101706, #24998, #57551, #50778, #8203 ),
 .UNSPECIFIED., .F., .F.,
 ( 4, 2, 2, 2, 2, 4 ),
 ( 0.000000000000000000, 0.0007194225121803534111, 0.001079133768270215590, 0.001438845024360077551, 0.002158267536539286695, 0.002877690048718496273 ),
 .UNSPECIFIED. ) ;
#27434=CARTESIAN_POINT ( 'NONE',  ( -32.09235212274860771, 1525.402221411349046, 221.9833860708173461 ) ) ;
#27436=CARTESIAN_POINT ( 'NONE',  ( 32.79520046278974377, 1523.954924407802309, 201.0814700520839438 ) ) ;
#27442=EDGE_CURVE ( 'NONE', #40850, #19317, #88548, .T. ) ;
#27444=CARTESIAN_POINT ( 'NONE',  ( -32.02808312589908013, 1512.187213306747481, 219.9649204700466782 ) ) ;
#27462=VERTEX_POINT ( 'NONE', #26912 ) ;
#27514=CARTESIAN_POINT ( 'NONE',  ( -18.72690275719048714, 1526.278758871496620, 182.1127646906402333 ) ) ;
#27516=CYLINDRICAL_SURFACE ( 'NONE', #40209, 2.000000000000006661 ) ;
#27517=EDGE_CURVE ( 'NONE', #100321, #53518, #60963, .T. ) ;
#27527=DIRECTION ( 'NONE',  ( -0.000000000000000000, -1.000000000000000000, -0.000000000000000000 ) ) ;
#27537=CARTESIAN_POINT ( 'NONE',  ( -31.47409394596284571, 1526.278758871496848, 218.5859237437391869 ) ) ;
#27538=LINE ( 'NONE', #102019, #66127 ) ;
#27545=CARTESIAN_POINT ( 'NONE',  ( 17.61555691395466638, 1524.600389084707103, 237.5961665349170744 ) ) ;
#27556=CYLINDRICAL_SURFACE ( 'NONE', #67019, 0.9999999999999967804 ) ;
#27558=CARTESIAN_POINT ( 'NONE',  ( -29.86281881105125180, 1525.137906803777014, 196.1139937296260598 ) ) ;
#27584=AXIS2_PLACEMENT_3D ( 'NONE', #18937, #86161, #62661 ) ;
#27588=DIRECTION ( 'NONE',  ( -0.000000000000000000, -1.000000000000000000, -0.000000000000000000 ) ) ;
#27596=EDGE_LOOP ( 'NONE', ( #69968, #36185, #11384, #106528 ) ) ;
#27598=FACE_OUTER_BOUND ( 'NONE', #101937, .T. ) ;
#27615=ORIENTED_EDGE ( 'NONE', *, *, #11999, .F. ) ;
#27636=ADVANCED_FACE ( 'NONE', ( #84754 ), #101062, .T. ) ;
#27652=EDGE_CURVE ( 'NONE', #79695, #42097, #61711, .T. ) ;
#27655=CARTESIAN_POINT ( 'NONE',  ( 30.47387511496750179, 1525.394057003703438, 221.5016029580054635 ) ) ;
#27658=CARTESIAN_POINT ( 'NONE',  ( 30.16747994869233196, 1524.964230758883104, 221.7255045378688862 ) ) ;
#27660=ORIENTED_EDGE ( 'NONE', *, *, #37977, .F. ) ;
#27661=CARTESIAN_POINT ( 'NONE',  ( -17.36692104388747637, 1525.425686270210235, 237.0071275365210681 ) ) ;
#27663=CARTESIAN_POINT ( 'NONE',  ( 29.00779973304128134, 1526.382868172864164, 217.2942086403122630 ) ) ;
#27664=CARTESIAN_POINT ( 'NONE',  ( 20.39147186912994769, 1526.073429442291854, 233.1306614363087419 ) ) ;
#27673=ORIENTED_EDGE ( 'NONE', *, *, #29514, .T. ) ;
#27697=CARTESIAN_POINT ( 'NONE',  ( -33.43367350703748997, 1524.397344074318653, 197.7663411554295578 ) ) ;
#27703=VECTOR ( 'NONE', #77320, 1000.000000000000000 ) ;
#27707=ORIENTED_EDGE ( 'NONE', *, *, #107775, .F. ) ;
#27719=LINE ( 'NONE', #8694, #110566 ) ;
#27732=CARTESIAN_POINT ( 'NONE',  ( 0.4151546846821903003, 1522.382868172863937, 173.3106345060153046 ) ) ;
#27744=DIRECTION ( 'NONE',  ( 0.000000000000000000, -1.000000000000000000, 0.000000000000000000 ) ) ;
#27748=ORIENTED_EDGE ( 'NONE', *, *, #75838, .F. ) ;
#27751=AXIS2_PLACEMENT_3D ( 'NONE', #39813, #80160, #47121 ) ;
#27774=AXIS2_PLACEMENT_3D ( 'NONE', #59233, #40750, #23389 ) ;
#27803=( BOUNDED_SURFACE ( )  B_SPLINE_SURFACE ( 3, 2, ( 
 ( #90628, #3906, #29623 ),
 ( #22297, #47002, #62731 ),
 ( #97381, #4970, #106875 ),
 ( #39115, #71688, #45901 ) ),
 .UNSPECIFIED., .F., .F., .F. ) 
 B_SPLINE_SURFACE_WITH_KNOTS ( ( 4, 4 ),
 ( 3, 3 ),
 ( 0.000000000000000000, 0.0002960034161023844057 ),
 ( 0.000000000000000000, 1.000000000000000000 ),
 .UNSPECIFIED. ) 
 GEOMETRIC_REPRESENTATION_ITEM ( )  RATIONAL_B_SPLINE_SURFACE ( (
 ( 1.000000000000000000, 0.8070209408750013136, 1.000000000000000000),
 ( 1.000000000000000000, 0.8071723757218328688, 1.000000000000000000),
 ( 1.000000000000000000, 0.8072480346917663141, 1.000000000000000000),
 ( 1.000000000000000000, 0.8072480644198083422, 1.000000000000000000) ) ) 
 REPRESENTATION_ITEM ( '' )  SURFACE ( )  );
#27810=CARTESIAN_POINT ( 'NONE',  ( -33.28034951413935261, 1522.382868172863937, 200.8029765415142549 ) ) ;
#27826=CARTESIAN_POINT ( 'NONE',  ( -31.44837959398599736, 1511.187213306747708, 197.3353852117985525 ) ) ;
#27828=CARTESIAN_POINT ( 'NONE',  ( 28.82451532742497946, 1526.348417187215318, 220.0525736641851609 ) ) ;
#27838=ORIENTED_EDGE ( 'NONE', *, *, #39743, .F. ) ;
#27842=ORIENTED_EDGE ( 'NONE', *, *, #103228, .F. ) ;
#27846=DIRECTION ( 'NONE',  ( -0.5369043659964716220, -0.4884709562386453929, -0.6878443331781037839 ) ) ;
#27859=DIRECTION ( 'NONE',  ( -0.2054769195713187224, 0.000000000000000000, 0.9786619618251655162 ) ) ;
#27888=CARTESIAN_POINT ( 'NONE',  ( -28.97303002314149367, 1526.186458717542109, 197.4313369063832511 ) ) ;
#27900=ORIENTED_EDGE ( 'NONE', *, *, #23589, .F. ) ;
#27917=ORIENTED_EDGE ( 'NONE', *, *, #106740, .T. ) ;
#27927=LINE ( 'NONE', #4249, #5632 ) ;
#27939=CYLINDRICAL_SURFACE ( 'NONE', #81548, 1.999999999999996669 ) ;
#27940=EDGE_CURVE ( 'NONE', #39550, #89436, #83183, .T. ) ;
#27950=CARTESIAN_POINT ( 'NONE',  ( -34.18677586421195258, 1522.382868172863937, 198.4504086008750505 ) ) ;
#27953=CARTESIAN_POINT ( 'NONE',  ( -1.775988990185336736, 1526.208281990536079, 240.5699127611742938 ) ) ;
#27968=ORIENTED_EDGE ( 'NONE', *, *, #109619, .T. ) ;
#27972=DIRECTION ( 'NONE',  ( -0.4090087482554183862, 0.000000000000000000, 0.9125304618754027652 ) ) ;
#27982=EDGE_LOOP ( 'NONE', ( #107628, #58428, #21238 ) ) ;
#27994=CARTESIAN_POINT ( 'NONE',  ( 31.11295512653393303, 1525.790287071783951, 201.8987506415136295 ) ) ;
#28000=DIRECTION ( 'NONE',  ( -0.8090169943749465631, -0.000000000000000000, 0.5877852522924742473 ) ) ;
#28004=VERTEX_POINT ( 'NONE', #16836 ) ;
#28018=DIRECTION ( 'NONE',  ( 0.4978433412588781914, 0.000000000000000000, 0.8672669759446606230 ) ) ;
#28019=DIRECTION ( 'NONE',  ( 0.000000000000000000, 0.000000000000000000, -1.000000000000000000 ) ) ;
#28029=DIRECTION ( 'NONE',  ( 0.7414773880254614813, 0.000000000000000000, -0.6709778558543786353 ) ) ;
#28041=ORIENTED_EDGE ( 'NONE', *, *, #39710, .T. ) ;
#28061=CARTESIAN_POINT ( 'NONE',  ( -156.6846457583342840, 1526.382868172863937, 340.9912860285748479 ) ) ;
#28064=CARTESIAN_POINT ( 'NONE',  ( -19.33418355719859960, 1523.342713519622748, 179.0109766843198997 ) ) ;
#28066=CARTESIAN_POINT ( 'NONE',  ( 2.902322711624676882E-15, 1523.051704408389696, 232.8211094035767985 ) ) ;
#28077=CARTESIAN_POINT ( 'NONE',  ( 18.19590854888166476, 1512.187213306747481, 238.2026672068774360 ) ) ;
#28078=DIRECTION ( 'NONE',  ( -0.000000000000000000, -1.000000000000000000, -0.000000000000000000 ) ) ;
#28086=CARTESIAN_POINT ( 'NONE',  ( -31.74003925669971338, 1524.382868172804365, 216.5565202880893878 ) ) ;
#28104=LINE ( 'NONE', #1265, #79556 ) ;
#28108=CARTESIAN_POINT ( 'NONE',  ( 32.86802468386284914, 1523.382868172864164, 201.0396662540042030 ) ) ;
#28127=EDGE_CURVE ( 'NONE', #10257, #89438, #26365, .T. ) ;
#28133=DIRECTION ( 'NONE',  ( -0.3090169943749515591, 0.000000000000000000, -0.9510565162951521989 ) ) ;
#28147=CARTESIAN_POINT ( 'NONE',  ( 21.51496489921850852, 1524.872178180563878, 183.6916733868881124 ) ) ;
#28155=( BOUNDED_SURFACE ( )  B_SPLINE_SURFACE ( 3, 2, ( 
 ( #99209, #22488, #56689 ),
 ( #90825, #48298, #5737 ),
 ( #39879, #34226, #85175 ),
 ( #101402, #103, #33661 ) ),
 .UNSPECIFIED., .F., .F., .T. ) 
 B_SPLINE_SURFACE_WITH_KNOTS ( ( 4, 4 ),
 ( 3, 3 ),
 ( 0.000000000000000000, 0.0002960034161023843515 ),
 ( 0.000000000000000000, 1.000000000000000000 ),
 .UNSPECIFIED. ) 
 GEOMETRIC_REPRESENTATION_ITEM ( )  RATIONAL_B_SPLINE_SURFACE ( (
 ( 1.000000000000000000, 0.8072480644198086752, 1.000000000000000000),
 ( 1.000000000000000000, 0.8072480346917653149, 1.000000000000000000),
 ( 1.000000000000000000, 0.8071723757218337569, 1.000000000000000000),
 ( 1.000000000000000000, 0.8070209408750013136, 1.000000000000000000) ) ) 
 REPRESENTATION_ITEM ( '' )  SURFACE ( )  );
#28165=ORIENTED_EDGE ( 'NONE', *, *, #107488, .T. ) ;
#28175=VECTOR ( 'NONE', #63236, 999.9999999999998863 ) ;
#28202=CARTESIAN_POINT ( 'NONE',  ( -31.12456774391156600, 1525.960063244517187, 217.0912716842400698 ) ) ;
#28210=CARTESIAN_POINT ( 'NONE',  ( -16.57702445344840569, 1524.523992613103246, 237.5566323917545901 ) ) ;
#28212=CARTESIAN_POINT ( 'NONE',  ( 30.31118248176371210, 1526.186458717542109, 216.6939452248806504 ) ) ;
#28263=CARTESIAN_POINT ( 'NONE',  ( -29.86461515634926656, 1525.960063244517187, 197.2746849027940925 ) ) ;
#28266=VECTOR ( 'NONE', #3505, 1000.000000000000000 ) ;
#28285=DIRECTION ( 'NONE',  ( -0.5877852522924785772, 0.000000000000000000, 0.8090169943749434545 ) ) ;
#28288=DIRECTION ( 'NONE',  ( 0.7414773880254630356, 0.000000000000000000, -0.6709778558543769700 ) ) ;
#28296=ORIENTED_EDGE ( 'NONE', *, *, #48004, .F. ) ;
#28298=VECTOR ( 'NONE', #20068, 1000.000000000000114 ) ;
#28300=DIRECTION ( 'NONE',  ( 0.000000000000000000, 0.000000000000000000, -1.000000000000000000 ) ) ;
#28307=TOROIDAL_SURFACE ( 'NONE', #89123, 1.000000000000000000, 1.000000000000000000 ) ;
#28325=AXIS2_PLACEMENT_3D ( 'NONE', #86518, #43977, #78677 ) ;
#28330=CARTESIAN_POINT ( 'NONE',  ( -30.30264253605756508, 1524.678541297860875, 221.8072158554251416 ) ) ;
#28341=CARTESIAN_POINT ( 'NONE',  ( 16.73628186595824019, 1526.382868172863937, 184.0591879540915272 ) ) ;
#28344=CARTESIAN_POINT ( 'NONE',  ( -17.84338787571901364, 1512.187213306747481, 237.8836641337663309 ) ) ;
#28356=DIRECTION ( 'NONE',  ( -0.7414773880254614813, 0.000000000000000000, 0.6709778558543786353 ) ) ;
#28358=CARTESIAN_POINT ( 'NONE',  ( -30.29107669316903539, 1523.847248782568613, 195.7510835661477984 ) ) ;
#28367=CARTESIAN_POINT ( 'NONE',  ( 2.180465155517623099, 1524.667648926078527, 244.2585483383492999 ) ) ;
#28377=LINE ( 'NONE', #64770, #96741 ) ;
#28383=CIRCLE ( 'NONE', #42694, 1.000000000000015099 ) ;
#28391=EDGE_CURVE ( 'NONE', #20574, #73846, #104599, .T. ) ;
#28401=CARTESIAN_POINT ( 'NONE',  ( -19.39983987835443457, 1501.977400791986611, 178.9515629539737631 ) ) ;
#28406=AXIS2_PLACEMENT_3D ( 'NONE', #25528, #26642, #67026 ) ;
#28412=ADVANCED_FACE ( 'NONE', ( #102928 ), #74328, .T. ) ;
#28414=CARTESIAN_POINT ( 'NONE',  ( 0.000000000000000000, 1512.187213306747481, 209.1218459616979999 ) ) ;
#28415=ORIENTED_EDGE ( 'NONE', *, *, #41949, .T. ) ;
#28441=EDGE_CURVE ( 'NONE', #11785, #15037, #4928, .T. ) ;
#28447=ORIENTED_EDGE ( 'NONE', *, *, #61317, .T. ) ;
#28462=AXIS2_PLACEMENT_3D ( 'NONE', #8270, #59266, #102874 ) ;
#28518=VECTOR ( 'NONE', #74961, 1000.000000000000000 ) ;
#28520=ADVANCED_FACE ( 'NONE', ( #11120, #2182 ), #96773, .F. ) ;
#28522=FACE_OUTER_BOUND ( 'NONE', #56317, .T. ) ;
#28538=CIRCLE ( 'NONE', #91111, 32.13701971169416538 ) ;
#28543=ORIENTED_EDGE ( 'NONE', *, *, #52472, .F. ) ;
#28546=EDGE_CURVE ( 'NONE', #77058, #82322, #65376, .T. ) ;
#28550=CARTESIAN_POINT ( 'NONE',  ( 32.38114538885250226, 1523.604703353109699, 202.1233279672528624 ) ) ;
#28556=DIRECTION ( 'NONE',  ( 0.000000000000000000, 1.000000000000000000, 0.000000000000000000 ) ) ;
#28560=CARTESIAN_POINT ( 'NONE',  ( -0.4151546846821903003, 1522.382868172863937, 175.3106345060153046 ) ) ;
#28562=ORIENTED_EDGE ( 'NONE', *, *, #7034, .F. ) ;
#28578=ORIENTED_EDGE ( 'NONE', *, *, #63930, .T. ) ;
#28581=ORIENTED_EDGE ( 'NONE', *, *, #49662, .T. ) ;
#28589=LINE ( 'NONE', #43744, #7432 ) ;
#28599=CARTESIAN_POINT ( 'NONE',  ( 30.79107737087824148, 1526.107876515966382, 201.1252789359793383 ) ) ;
#28608=CARTESIAN_POINT ( 'NONE',  ( -31.23437356469425907, 1512.187213306747481, 222.8968241038848248 ) ) ;
#28613=CARTESIAN_POINT ( 'NONE',  ( -30.51231035492526900, 1526.382868172863937, 200.0858385050243555 ) ) ;
#28622=CARTESIAN_POINT ( 'NONE',  ( -21.08704007906051459, 1525.317349363567700, 233.7719395062865146 ) ) ;
#28623=CARTESIAN_POINT ( 'NONE',  ( 0.000000000000000000, 1512.187213306747481, 209.1218459616979999 ) ) ;
#28654=AXIS2_PLACEMENT_3D ( 'NONE', #3926, #19588, #62752 ) ;
#28660=ORIENTED_EDGE ( 'NONE', *, *, #31801, .T. ) ;
#28663=CARTESIAN_POINT ( 'NONE',  ( 33.93019615848945847, 1522.382868172863937, 197.6607374645996060 ) ) ;
#28669=CARTESIAN_POINT ( 'NONE',  ( 19.02270174365980893, 1526.382868172864164, 232.8547275633986828 ) ) ;
#28675=DIRECTION ( 'NONE',  ( -0.07713599384728245245, -0.9969860201949397593, -0.008301444997533467124 ) ) ;
#28685=EDGE_CURVE ( 'NONE', #5040, #10960, #65935, .T. ) ;
#28694=AXIS2_PLACEMENT_3D ( 'NONE', #23469, #41393, #75558 ) ;
#28700=AXIS2_PLACEMENT_3D ( 'NONE', #107703, #14734, #23126 ) ;
#28728=VECTOR ( 'NONE', #99929, 1000.000000000000114 ) ;
#28736=LINE ( 'NONE', #21401, #32456 ) ;
#28757=CARTESIAN_POINT ( 'NONE',  ( -2.225547318884174786, 1525.712830164893376, 241.5729992621096756 ) ) ;
#28766=CIRCLE ( 'NONE', #37716, 2.000000000000001776 ) ;
#28767=CARTESIAN_POINT ( 'NONE',  ( -17.10350668511973993, 1524.477587234265911, 237.2713348840137542 ) ) ;
#28783=AXIS2_PLACEMENT_3D ( 'NONE', #15838, #110484, #7470 ) ;
#28793=CARTESIAN_POINT ( 'NONE',  ( -31.23437356469455040, 1512.187213306747481, 195.3468678195118287 ) ) ;
#28806=CARTESIAN_POINT ( 'NONE',  ( -30.79697748855988593, 1526.178928173328131, 196.3997152352021942 ) ) ;
#28819=CARTESIAN_POINT ( 'NONE',  ( 16.66936639845652834, 1512.187213306747481, 237.7608804993219280 ) ) ;
#28874=CARTESIAN_POINT ( 'NONE',  ( 2.038646110889678287, 1525.960063244516959, 177.0579350083066004 ) ) ;
#28878=CARTESIAN_POINT ( 'NONE',  ( 18.97665094185096990, 1526.382868172863937, 232.9676995165609412 ) ) ;
#28885=CARTESIAN_POINT ( 'NONE',  ( -30.57065064348379835, 1523.844782250847175, 221.8563543952624855 ) ) ;
#28912=DIRECTION ( 'NONE',  ( -0.9948834766775040972, 0.000000000000000000, 0.1010290445074212007 ) ) ;
#28913=EDGE_CURVE ( 'NONE', #13345, #58330, #26001, .T. ) ;
#28916=ADVANCED_FACE ( 'NONE', ( #76499 ), #67571, .T. ) ;
#28927=EDGE_CURVE ( 'NONE', #14943, #40151, #68134, .T. ) ;
#28931=CARTESIAN_POINT ( 'NONE',  ( 3.347801439296143933, 1523.382868172864164, 242.0893193391992497 ) ) ;
#28936=CARTESIAN_POINT ( 'NONE',  ( -2.385609062339151709, 1525.697947650495507, 241.0978138787441480 ) ) ;
#28974=EDGE_CURVE ( 'NONE', #95247, #20553, #79688, .T. ) ;
#28980=AXIS2_PLACEMENT_3D ( 'NONE', #93486, #10046, #16756 ) ;
#28991=CARTESIAN_POINT ( 'NONE',  ( -0.4151546846821905223, 1524.726013923371283, 244.9330574173806383 ) ) ;
#29030=LINE ( 'NONE', #10011, #11459 ) ;
#29041=CARTESIAN_POINT ( 'NONE',  ( 2.622430729443033126, 1523.621879633029039, 242.1535192357228823 ) ) ;
#29042=ORIENTED_EDGE ( 'NONE', *, *, #53428, .F. ) ;
#29061=DIRECTION ( 'NONE',  ( 0.6709778558543786353, 0.000000000000000000, 0.7414773880254614813 ) ) ;
#29069=CARTESIAN_POINT ( 'NONE',  ( 29.00779973304130266, 1526.382868172863937, 200.9494832830834810 ) ) ;
#29091=CARTESIAN_POINT ( 'NONE',  ( -17.17241001986462123, 1518.913060387330006, 238.6251415217917895 ) ) ;
#29101=CARTESIAN_POINT ( 'NONE',  ( 31.12456774391176850, 1525.960063244516959, 201.1524202391561857 ) ) ;
#29107=CARTESIAN_POINT ( 'NONE',  ( 31.12456774391179692, 1525.960063244516959, 201.1524202391561573 ) ) ;
#29127=EDGE_LOOP ( 'NONE', ( #8512, #72686, #104754, #91428 ) ) ;
#29129=CARTESIAN_POINT ( 'NONE',  ( 29.00779973304137371, 1526.382868172863937, 217.2942086403122914 ) ) ;
#29148=ORIENTED_EDGE ( 'NONE', *, *, #74314, .T. ) ;
#29150=CARTESIAN_POINT ( 'NONE',  ( 2.737416067801661690, 1524.382868172804365, 176.6378340846514448 ) ) ;
#29170=B_SPLINE_CURVE_WITH_KNOTS ( 'NONE', 3,
 ( #58269, #66681, #93495, #67775, #75628, #76708, #49868, #94052 ),
 .UNSPECIFIED., .F., .F.,
 ( 4, 2, 2, 4 ),
 ( 0.000000000000000000, 0.001073044933456180836, 0.001609567400184301177, 0.002146089866912421519 ),
 .UNSPECIFIED. ) ;
#29173=CARTESIAN_POINT ( 'NONE',  ( 0.4151546846821903003, 1511.187213306747708, 175.3106345060153046 ) ) ;
#29216=CARTESIAN_POINT ( 'NONE',  ( -29.91204167771525135, 1525.042412244735488, 196.0616339290309611 ) ) ;
#29234=DIRECTION ( 'NONE',  ( 0.000000000000000000, 1.000000000000000000, 0.000000000000000000 ) ) ;
#29240=DIRECTION ( 'NONE',  ( 0.000000000000000000, -1.000000000000000000, -0.000000000000000000 ) ) ;
#29241=CARTESIAN_POINT ( 'NONE',  ( -20.71343476517491311, 1512.187213306747481, 238.3377464195766890 ) ) ;
#29269=VERTEX_POINT ( 'NONE', #67856 ) ;
#29271=ORIENTED_EDGE ( 'NONE', *, *, #31692, .T. ) ;
#29284=VERTEX_POINT ( 'NONE', #42636 ) ;
#29308=ORIENTED_EDGE ( 'NONE', *, *, #5258, .F. ) ;
#29309=FACE_OUTER_BOUND ( 'NONE', #86252, .T. ) ;
#29317=FACE_OUTER_BOUND ( 'NONE', #13957, .T. ) ;
#29326=DIRECTION ( 'NONE',  ( 0.9149707217702551798, 0.000000000000000000, -0.4035202328300510621 ) ) ;
#29335=VECTOR ( 'NONE', #100184, 1000.000000000000000 ) ;
#29360=LINE ( 'NONE', #12021, #94024 ) ;
#29384=CARTESIAN_POINT ( 'NONE',  ( -16.85976061912594304, 1525.821544997590763, 182.0492613858613709 ) ) ;
#29385=CARTESIAN_POINT ( 'NONE',  ( 21.08703188481580071, 1525.317359687823455, 233.7719348611598775 ) ) ;
#29392=ORIENTED_EDGE ( 'NONE', *, *, #74301, .F. ) ;
#29407=AXIS2_PLACEMENT_3D ( 'NONE', #31213, #73227, #40167 ) ;
#29410=CARTESIAN_POINT ( 'NONE',  ( 21.84020450222037724, 1523.382868172864164, 183.2638850454218016 ) ) ;
#29418=CARTESIAN_POINT ( 'NONE',  ( -30.83422926911917727, 1524.871836253796118, 221.7255529736243602 ) ) ;
#29422=ORIENTED_EDGE ( 'NONE', *, *, #22749, .F. ) ;
#29468=CARTESIAN_POINT ( 'NONE',  ( -2.693001348318031063, 1524.059663615500085, 242.0866550885344282 ) ) ;
#29480=CARTESIAN_POINT ( 'NONE',  ( -16.73628186595804479, 1526.382868172863937, 234.1845039693045862 ) ) ;
#29484=PLANE ( 'NONE',  #92173 ) ;
#29485=DIRECTION ( 'NONE',  ( -0.7454942576402588950, 0.000000000000000000, 0.6665120492724789791 ) ) ;
#29496=CIRCLE ( 'NONE', #90234, 2.000000000000001776 ) ;
#29500=CARTESIAN_POINT ( 'NONE',  ( 33.05665451062059645, 1523.390106123591067, 200.9313857523606544 ) ) ;
#29503=ORIENTED_EDGE ( 'NONE', *, *, #75415, .T. ) ;
#29514=EDGE_CURVE ( 'NONE', #16271, #97990, #650, .T. ) ;
#29517=CARTESIAN_POINT ( 'NONE',  ( -30.12521068615179942, 1524.538969332612623, 222.3851261604999365 ) ) ;
#29525=ORIENTED_EDGE ( 'NONE', *, *, #82409, .F. ) ;
#29531=VERTEX_POINT ( 'NONE', #39741 ) ;
#29558=ORIENTED_EDGE ( 'NONE', *, *, #82503, .T. ) ;
#29560=DIRECTION ( 'NONE',  ( 0.000000000000000000, 1.000000000000000000, 0.000000000000000000 ) ) ;
#29569=CARTESIAN_POINT ( 'NONE',  ( 32.86802468386284914, 1523.382868172864164, 201.0396662540042030 ) ) ;
#29573=ORIENTED_EDGE ( 'NONE', *, *, #61279, .F. ) ;
#29590=ORIENTED_EDGE ( 'NONE', *, *, #24225, .T. ) ;
#29594=CARTESIAN_POINT ( 'NONE',  ( -1.439851189671583542, 1526.382868172864164, 239.5034140466476060 ) ) ;
#29605=B_SPLINE_CURVE_WITH_KNOTS ( 'NONE', 3,
 ( #1677, #88963, #39672, #90054, #55935, #80575, #96836, #107414, #63256, #4955 ),
 .UNSPECIFIED., .F., .F.,
 ( 4, 2, 2, 2, 4 ),
 ( 0.000000000000000000, 0.0007189769279725886052, 0.001437953855945177210, 0.002156930783917765816, 0.002875907711890354421 ),
 .UNSPECIFIED. ) ;
#29608=ADVANCED_FACE ( 'NONE', ( #54909 ), #52381, .F. ) ;
#29614=ORIENTED_EDGE ( 'NONE', *, *, #83701, .F. ) ;
#29615=AXIS2_PLACEMENT_3D ( 'NONE', #8176, #17663, #69221 ) ;
#29623=CARTESIAN_POINT ( 'NONE',  ( 2.472529913803013901, 1523.678648413191695, 242.8674788698241684 ) ) ;
#29633=CARTESIAN_POINT ( 'NONE',  ( 20.64339891394584114, 1523.429859730330236, 238.2599442700835937 ) ) ;
#29636=EDGE_CURVE ( 'NONE', #21131, #5947, #100847, .T. ) ;
#29659=AXIS2_PLACEMENT_3D ( 'NONE', #31631, #84241, #6444 ) ;
#29680=VECTOR ( 'NONE', #66232, 1000.000000000000227 ) ;
#29687=ORIENTED_EDGE ( 'NONE', *, *, #95300, .T. ) ;
#29692=CARTESIAN_POINT ( 'NONE',  ( 2.057041824809119568, 1523.342713519622521, 173.3972930408587558 ) ) ;
#29693=DIRECTION ( 'NONE',  ( 0.000000000000000000, 0.000000000000000000, 1.000000000000000000 ) ) ;
#29719=CARTESIAN_POINT ( 'NONE',  ( 32.02808312589922224, 1512.187213306747481, 219.9649204700462235 ) ) ;
#29728=FACE_OUTER_BOUND ( 'NONE', #37904, .T. ) ;
#29736=CARTESIAN_POINT ( 'NONE',  ( 0.000000000000000000, 1518.913060387330006, 209.1218459616979999 ) ) ;
#29743=LINE ( 'NONE', #40346, #44386 ) ;
#29762=DIRECTION ( 'NONE',  ( 0.3090169943749383474, 0.000000000000000000, -0.9510565162951566398 ) ) ;
#29764=CARTESIAN_POINT ( 'NONE',  ( -2.472529913803013901, 1523.678648413191695, 175.3762130535718313 ) ) ;
#29769=( BOUNDED_SURFACE ( )  B_SPLINE_SURFACE ( 3, 2, ( 
 ( #23410, #91722, #101760 ),
 ( #68213, #42421, #84961 ),
 ( #58690, #8255, #109096 ),
 ( #32378, #33451, #76579 ),
 ( #41332, #66558, #108526 ),
 ( #24500, #31818, #67652 ),
 ( #100126, #110731, #34020 ),
 ( #22842, #92823, #14453 ),
 ( #49194, #23946, #58142 ),
 ( #48646, #16094, #92274 ) ),
 .UNSPECIFIED., .F., .F., .F. ) 
 B_SPLINE_SURFACE_WITH_KNOTS ( ( 4, 2, 2, 2, 4 ),
 ( 3, 3 ),
 ( 1.570796326794896558, 1.963495408493620697, 2.356194490192344837, 2.748893571891068976, 3.141592653589793116 ),
 ( 0.000000000000000000, 1.000000000000000000 ),
 .UNSPECIFIED. ) 
 GEOMETRIC_REPRESENTATION_ITEM ( )  RATIONAL_B_SPLINE_SURFACE ( (
 ( 1.000000000000000000, 0.7071067811865813235, 1.000000000000000000),
 ( 1.000000000000000000, 0.7166207884823980745, 1.000000000000000000),
 ( 1.000000000000000000, 0.7259222650904582075, 1.000000000000000000),
 ( 1.000000000000000000, 0.7428408967932866869, 1.000000000000000000),
 ( 1.000000000000000000, 0.7504512394528688457, 1.000000000000000000),
 ( 1.000000000000000000, 0.7630177051946271938, 1.000000000000000000),
 ( 1.000000000000000000, 0.7679730451969652982, 1.000000000000000000),
 ( 1.000000000000000000, 0.7746454561800797389, 1.000000000000000000),
 ( 1.000000000000000000, 0.7763684247032546226, 1.000000000000000000),
 ( 1.000000000000000000, 0.7763623250684360544, 1.000000000000000000) ) ) 
 REPRESENTATION_ITEM ( '' )  SURFACE ( )  );
#29770=CARTESIAN_POINT ( 'NONE',  ( 32.28466283162151029, 1511.187213306747708, 199.0684425896244250 ) ) ;
#29772=DIRECTION ( 'NONE',  ( -0.000000000000000000, 1.000000000000000000, -0.000000000000000000 ) ) ;
#29784=CYLINDRICAL_SURFACE ( 'NONE', #74126, 0.9999999999999976685 ) ;
#29787=ADVANCED_FACE ( 'NONE', ( #108470 ), #67210, .T. ) ;
#29795=ADVANCED_FACE ( 'NONE', ( #31754 ), #18893, .T. ) ;
#29847=AXIS2_PLACEMENT_3D ( 'NONE', #102550, #51630, #52194 ) ;
#29862=CARTESIAN_POINT ( 'NONE',  ( 16.73628186595820111, 1526.382868172864164, 184.0591879540915841 ) ) ;
#29889=DIRECTION ( 'NONE',  ( 0.000000000000000000, 0.000000000000000000, -1.000000000000000000 ) ) ;
#29898=CARTESIAN_POINT ( 'NONE',  ( -18.97796697799288879, 1526.382868172864164, 232.9684741896490721 ) ) ;
#29934=EDGE_LOOP ( 'NONE', ( #61677, #65918, #100995, #78271 ) ) ;
#29935=FACE_OUTER_BOUND ( 'NONE', #89439, .T. ) ;
#29937=VERTEX_POINT ( 'NONE', #63494 ) ;
#29942=CARTESIAN_POINT ( 'NONE',  ( 29.78220350812341266, 1524.382868172863937, 196.5089261231631212 ) ) ;
#29953=ORIENTED_EDGE ( 'NONE', *, *, #84660, .F. ) ;
#29954=CARTESIAN_POINT ( 'NONE',  ( -29.86461515634900010, 1525.960063244516959, 220.9690070206027031 ) ) ;
#29969=CARTESIAN_POINT ( 'NONE',  ( 29.13898522074257258, 1526.069472839378022, 197.1409705599812128 ) ) ;
#29985=CARTESIAN_POINT ( 'NONE',  ( 22.08622291482331690, 1523.382868172864164, 184.4183880513174927 ) ) ;
#29988=CIRCLE ( 'NONE', #53197, 1.000000000000000888 ) ;
#29992=VERTEX_POINT ( 'NONE', #9736 ) ;
#30005=CARTESIAN_POINT ( 'NONE',  ( 2.456601303385837820, 1523.611961620354123, 242.9433449337720958 ) ) ;
#30009=CARTESIAN_POINT ( 'NONE',  ( -30.31643683090000962, 1523.530935881284904, 195.7504610701758168 ) ) ;
#30010=AXIS2_PLACEMENT_3D ( 'NONE', #1568, #86652, #52521 ) ;
#30014=CARTESIAN_POINT ( 'NONE',  ( -2.487422374635116284, 1523.954924407802764, 242.7965478622698754 ) ) ;
#30017=CARTESIAN_POINT ( 'NONE',  ( 3.246772394788718596, 1512.187213306747481, 177.1492560608742508 ) ) ;
#30026=VERTEX_POINT ( 'NONE', #95408 ) ;
#30040=CIRCLE ( 'NONE', #6863, 0.9999999999999980016 ) ;
#30041=CARTESIAN_POINT ( 'NONE',  ( -0.4260839224734093711, 1523.429859730329781, 244.8289481157578393 ) ) ;
#30045=AXIS2_PLACEMENT_3D ( 'NONE', #46027, #61192, #19693 ) ;
#30047=CARTESIAN_POINT ( 'NONE',  ( 31.74003925669979154, 1524.382868172804365, 201.6871716353068109 ) ) ;
#30049=ORIENTED_EDGE ( 'NONE', *, *, #39779, .F. ) ;
#30056=CARTESIAN_POINT ( 'NONE',  ( -204.2714532754874881, 1524.382868172863937, 194.5341519463070767 ) ) ;
#30075=VERTEX_POINT ( 'NONE', #97070 ) ;
#30077=( BOUNDED_CURVE ( )  B_SPLINE_CURVE ( 3, ( #77951, #78513, #86901, #12392 ),
 .UNSPECIFIED., .F., .F. ) 
 B_SPLINE_CURVE_WITH_KNOTS ( ( 4, 4 ),
 ( 2.436781329611980240, 3.141592653589793116 ),
 .UNSPECIFIED. ) 
 CURVE ( )  GEOMETRIC_REPRESENTATION_ITEM ( )  RATIONAL_B_SPLINE_CURVE ( ( 1.000000000000000000, 0.9590300661663084814, 0.9590300661663084814, 1.000000000000000000 ) ) 
 REPRESENTATION_ITEM ( '' )  );
#30083=DIRECTION ( 'NONE',  ( 0.000000000000000000, 0.000000000000000000, -1.000000000000000000 ) ) ;
#30098=EDGE_LOOP ( 'NONE', ( #77196, #78416, #40895, #5462 ) ) ;
#30100=ORIENTED_EDGE ( 'NONE', *, *, #104370, .T. ) ;
#30109=DIRECTION ( 'NONE',  ( 0.000000000000000000, 0.000000000000000000, 1.000000000000000000 ) ) ;
#30112=CARTESIAN_POINT ( 'NONE',  ( 30.31644210119978311, 1523.530870145309564, 222.4932309826555183 ) ) ;
#30115=VECTOR ( 'NONE', #49090, 1000.000000000000000 ) ;
#30121=AXIS2_PLACEMENT_3D ( 'NONE', #30732, #57068, #72754 ) ;
#30130=DIRECTION ( 'NONE',  ( -1.000000000000000000, 0.000000000000000000, 0.000000000000000000 ) ) ;
#30149=DIRECTION ( 'NONE',  ( 0.000000000000000000, 0.000000000000000000, 1.000000000000000000 ) ) ;
#30158=ORIENTED_EDGE ( 'NONE', *, *, #53746, .F. ) ;
#30161=CARTESIAN_POINT ( 'NONE',  ( 76.99707197884903564, 1526.382868172863937, 19.35599459046138193 ) ) ;
#30166=CARTESIAN_POINT ( 'NONE',  ( 34.18677586421188863, 1512.187213306747481, 219.7932833225211766 ) ) ;
#30178=CARTESIAN_POINT ( 'NONE',  ( 19.39983987835401535, 1501.977400791986611, 178.9515629539735073 ) ) ;
#30196=EDGE_LOOP ( 'NONE', ( #62930, #100008, #21829, #76379, #20491 ) ) ;
#30213=VERTEX_POINT ( 'NONE', #80814 ) ;
#30223=CARTESIAN_POINT ( 'NONE',  ( 16.73628186595829703, 1526.382868172864164, 234.1845039693042452 ) ) ;
#30271=CYLINDRICAL_SURFACE ( 'NONE', #21506, 1.000000000000000888 ) ;
#30274=CARTESIAN_POINT ( 'NONE',  ( -21.41029105011321576, 1526.329757971584741, 234.0206363885986320 ) ) ;
#30276=DIRECTION ( 'NONE',  ( 0.5877852522924709167, 0.000000000000000000, 0.8090169943749491166 ) ) ;
#30289=CARTESIAN_POINT ( 'NONE',  ( 18.15646965371242771, 1522.906363951597314, 180.0767137688687001 ) ) ;
#30295=FACE_OUTER_BOUND ( 'NONE', #38093, .T. ) ;
#30300=DIRECTION ( 'NONE',  ( 0.000000000000000000, 0.000000000000000000, -1.000000000000000000 ) ) ;
#30313=CARTESIAN_POINT ( 'NONE',  ( -2.621078202466434082, 1523.542365884045466, 176.0837307636415972 ) ) ;
#30315=ORIENTED_EDGE ( 'NONE', *, *, #61170, .F. ) ;
#30320=CARTESIAN_POINT ( 'NONE',  ( 0.000000000000000000, 1524.090675761330203, 209.1218459616979999 ) ) ;
#30321=CIRCLE ( 'NONE', #57213, 0.9999999999999935607 ) ;
#30329=DIRECTION ( 'NONE',  ( 0.000000000000000000, 0.000000000000000000, -1.000000000000000000 ) ) ;
#30358=VECTOR ( 'NONE', #45402, 1000.000000000000114 ) ;
#30392=CARTESIAN_POINT ( 'NONE',  ( -21.98490254033148972, 1525.713797967456912, 182.9410524212120777 ) ) ;
#30404=VERTEX_POINT ( 'NONE', #28613 ) ;
#30405=CARTESIAN_POINT ( 'NONE',  ( -17.78112816951914610, 1523.954914175594695, 237.8273240688543524 ) ) ;
#30407=CARTESIAN_POINT ( 'NONE',  ( -22.75273496409559826, 1511.187213306747708, 234.5707981297189235 ) ) ;
#30427=( BOUNDED_SURFACE ( )  B_SPLINE_SURFACE ( 3, 2, ( 
 ( #7165, #39090, #32898 ),
 ( #48637, #65438, #91714 ),
 ( #22833, #92264, #83863 ),
 ( #6059, #4948, #13886 ) ),
 .UNSPECIFIED., .F., .F., .T. ) 
 B_SPLINE_SURFACE_WITH_KNOTS ( ( 4, 4 ),
 ( 3, 3 ),
 ( 0.000000000000000000, 0.0002960034161023845684 ),
 ( 0.000000000000000000, 1.000000000000000000 ),
 .UNSPECIFIED. ) 
 GEOMETRIC_REPRESENTATION_ITEM ( )  RATIONAL_B_SPLINE_SURFACE ( (
 ( 1.000000000000000000, 0.8070209408750042002, 1.000000000000000000),
 ( 1.000000000000000000, 0.8071723757218286499, 1.000000000000000000),
 ( 1.000000000000000000, 0.8072480346917807470, 1.000000000000000000),
 ( 1.000000000000000000, 0.8072480644198112287, 1.000000000000000000) ) ) 
 REPRESENTATION_ITEM ( '' )  SURFACE ( )  );
#30447=AXIS2_PLACEMENT_3D ( 'NONE', #104452, #27744, #28300 ) ;
#30450=CARTESIAN_POINT ( 'NONE',  ( 31.88715249297890253, 1525.425686270225242, 217.0217434889228798 ) ) ;
#30456=ORIENTED_EDGE ( 'NONE', *, *, #103879, .F. ) ;
#30457=CARTESIAN_POINT ( 'NONE',  ( 31.34137657934018506, 1523.481610426287716, 221.9025654077410081 ) ) ;
#30459=CARTESIAN_POINT ( 'NONE',  ( -17.17241001986463189, 1523.382868172864164, 238.6251415217917895 ) ) ;
#30486=SURFACE_STYLE_FILL_AREA ( #83643 ) ;
#30492=DIRECTION ( 'NONE',  ( 0.000000000000000000, 1.000000000000000000, 0.000000000000000000 ) ) ;
#30493=CARTESIAN_POINT ( 'NONE',  ( 22.08327125186946915, 1523.604703353109926, 233.8169256665487410 ) ) ;
#30502=VERTEX_POINT ( 'NONE', #100747 ) ;
#30510=AXIS2_PLACEMENT_3D ( 'NONE', #29091, #47007, #38575 ) ;
#30516=VERTEX_POINT ( 'NONE', #66095 ) ;
#30526=CARTESIAN_POINT ( 'NONE',  ( 29.16136750931930166, 1526.143142182216479, 197.5843855542958352 ) ) ;
#30554=CARTESIAN_POINT ( 'NONE',  ( 0.000000000000000000, 1511.187213306747708, 209.1218459616979999 ) ) ;
#30577=CARTESIAN_POINT ( 'NONE',  ( -2.494575337237918689, 1524.201816949777367, 242.7026873301162482 ) ) ;
#30588=ORIENTED_EDGE ( 'NONE', *, *, #45659, .T. ) ;
#30605=CARTESIAN_POINT ( 'NONE',  ( -0.4151546846839010985, 1522.906561336852974, 244.9330574173806951 ) ) ;
#30611=CARTESIAN_POINT ( 'NONE',  ( 32.39315898239293290, 1526.178928173327449, 201.3122567411275838 ) ) ;
#30614=ORIENTED_EDGE ( 'NONE', *, *, #91290, .T. ) ;
#30621=DIRECTION ( 'NONE',  ( 0.5369043659964899406, -0.4884709562386497228, 0.6878443331780863534 ) ) ;
#30637=DIRECTION ( 'NONE',  ( 0.000000000000000000, 1.000000000000000000, 0.000000000000000000 ) ) ;
#30645=LINE ( 'NONE', #98938, #82019 ) ;
#30656=DIRECTION ( 'NONE',  ( 0.8672669759446630655, 0.000000000000000000, -0.4978433412588735285 ) ) ;
#30668=EDGE_LOOP ( 'NONE', ( #12361, #14559, #64801, #77748, #67992, #50545, #109011, #91725 ) ) ;
#30675=CARTESIAN_POINT ( 'NONE',  ( 32.23393008293232498, 1523.462669333491704, 201.4036600224296478 ) ) ;
#30676=DIRECTION ( 'NONE',  ( 0.9510565162951566398, 0.000000000000000000, 0.3090169943749382919 ) ) ;
#30691=EDGE_CURVE ( 'NONE', #69179, #81290, #3367, .T. ) ;
#30692=CARTESIAN_POINT ( 'NONE',  ( -21.54116136312547880, 1523.382868172864391, 183.9310736446958856 ) ) ;
#30695=CARTESIAN_POINT ( 'NONE',  ( -31.10385014139604820, 1525.795403383247276, 201.8948722003923990 ) ) ;
#30713=AXIS2_PLACEMENT_3D ( 'NONE', #35100, #110705, #93343 ) ;
#30716=CARTESIAN_POINT ( 'NONE',  ( -30.95751052620443033, 1525.821544997589854, 216.7905424461075654 ) ) ;
#30719=EDGE_LOOP ( 'NONE', ( #75797, #4638, #28578, #11147, #84317 ) ) ;
#30732=CARTESIAN_POINT ( 'NONE',  ( 0.000000000000000000, 1512.187213306747481, 209.1218459616979999 ) ) ;
#30733=ORIENTED_EDGE ( 'NONE', *, *, #91619, .F. ) ;
#30736=CARTESIAN_POINT ( 'NONE',  ( 18.37487226820591246, 1526.382868172863937, 235.7398599686385694 ) ) ;
#30747=CARTESIAN_POINT ( 'NONE',  ( 3.258294392304168507, 1524.756004293092474, 176.4770358516228725 ) ) ;
#30772=ORIENTED_EDGE ( 'NONE', *, *, #86300, .T. ) ;
#30781=ORIENTED_EDGE ( 'NONE', *, *, #61862, .F. ) ;
#30793=CARTESIAN_POINT ( 'NONE',  ( 16.73628186595838940, 1526.382868172863937, 234.1845039693043589 ) ) ;
#30820=EDGE_CURVE ( 'NONE', #46121, #13274, #33540, .T. ) ;
#30823=PLANE ( 'NONE',  #58057 ) ;
#30827=CARTESIAN_POINT ( 'NONE',  ( -22.69876404240055479, 1522.382868172864391, 236.8953202675780858 ) ) ;
#30831=FACE_OUTER_BOUND ( 'NONE', #93494, .T. ) ;
#30833=CARTESIAN_POINT ( 'NONE',  ( 21.19079385647347991, 1525.394057003703438, 183.9650237549345491 ) ) ;
#30845=ORIENTED_EDGE ( 'NONE', *, *, #87069, .F. ) ;
#30846=CARTESIAN_POINT ( 'NONE',  ( -17.29393938232497518, 1523.621879633028584, 180.8572348224460882 ) ) ;
#30850=EDGE_CURVE ( 'NONE', #5224, #41836, #108356, .T. ) ;
#30852=CYLINDRICAL_SURFACE ( 'NONE', #59899, 2.000000000000001776 ) ;
#30878=CARTESIAN_POINT ( 'NONE',  ( 14.22993178683297266, 1512.187213306747481, 236.2420368605362455 ) ) ;
#30883=ORIENTED_EDGE ( 'NONE', *, *, #42012, .T. ) ;
#30890=ORIENTED_EDGE ( 'NONE', *, *, #47763, .T. ) ;
#30901=ADVANCED_FACE ( 'NONE', ( #4917 ), #24335, .F. ) ;
#30910=ORIENTED_EDGE ( 'NONE', *, *, #32415, .T. ) ;
#30924=ADVANCED_FACE ( 'NONE', ( #12778 ), #46955, .F. ) ;
#30935=CARTESIAN_POINT ( 'NONE',  ( 19.53786426059019021, 1511.187213306747708, 180.5239794925693388 ) ) ;
#30945=CARTESIAN_POINT ( 'NONE',  ( -21.61625474793611446, 1526.178928173327449, 183.7635344381546361 ) ) ;
#30950=EDGE_CURVE ( 'NONE', #18078, #13119, #95543, .T. ) ;
#30959=CARTESIAN_POINT ( 'NONE',  ( -16.66231036550680500, 1523.604703353109926, 237.7554842931448036 ) ) ;
#30975=EDGE_CURVE ( 'NONE', #32282, #108592, #77103, .T. ) ;
#30992=CARTESIAN_POINT ( 'NONE',  ( -20.20959865099510111, 1522.382868172863937, 182.0120230947222524 ) ) ;
#30998=FACE_OUTER_BOUND ( 'NONE', #91249, .T. ) ;
#31039=CARTESIAN_POINT ( 'NONE',  ( -16.73628186595857059, 1526.382868172864164, 184.0591879540917546 ) ) ;
#31040=CARTESIAN_POINT ( 'NONE',  ( 22.07691437628581710, 1523.843263703803586, 233.7988804623609269 ) ) ;
#31050=EDGE_CURVE ( 'NONE', #21147, #43726, #88802, .T. ) ;
#31063=CARTESIAN_POINT ( 'NONE',  ( -31.26701299884003404, 1523.919943579690425, 196.3491295910356769 ) ) ;
#31065=EDGE_CURVE ( 'NONE', #40736, #59940, #1975, .T. ) ;
#31075=CARTESIAN_POINT ( 'NONE',  ( 28.82451532742483735, 1526.348417187219184, 198.1911182592214402 ) ) ;
#31080=CARTESIAN_POINT ( 'NONE',  ( 19.37374569213945463, 1526.382868172863937, 234.3668155954418637 ) ) ;
#31084=ORIENTED_EDGE ( 'NONE', *, *, #57599, .F. ) ;
#31103=CIRCLE ( 'NONE', #91927, 1.000000000000000888 ) ;
#31120=CARTESIAN_POINT ( 'NONE',  ( 32.52419458002820107, 1524.600389084707103, 201.1675047309180968 ) ) ;
#31132=VERTEX_POINT ( 'NONE', #38386 ) ;
#31136=ORIENTED_EDGE ( 'NONE', *, *, #28127, .T. ) ;
#31153=VERTEX_POINT ( 'NONE', #106690 ) ;
#31181=EDGE_CURVE ( 'NONE', #41312, #58330, #99939, .T. ) ;
#31213=CARTESIAN_POINT ( 'NONE',  ( -29.40443212115400939, 1512.187213306747481, 196.1539082851718661 ) ) ;
#31223=CARTESIAN_POINT ( 'NONE',  ( 29.99620953741488449, 1526.382868172863937, 198.4974435154498735 ) ) ;
#31238=CARTESIAN_POINT ( 'NONE',  ( -0.4151546846821904668, 1524.726013923371283, 173.3106345060153330 ) ) ;
#31246=EDGE_LOOP ( 'NONE', ( #65772, #27707, #36471, #2664 ) ) ;
#31247=ORIENTED_EDGE ( 'NONE', *, *, #109623, .T. ) ;
#31250=FACE_OUTER_BOUND ( 'NONE', #44309, .T. ) ;
#31269=LINE ( 'NONE', #4433, #7216 ) ;
#31278=CYLINDRICAL_SURFACE ( 'NONE', #91094, 4.000000000000000000 ) ;
#31282=CARTESIAN_POINT ( 'NONE',  ( 156.6846457583332892, 1524.382868172863937, 77.25240589481998654 ) ) ;
#31287=AXIS2_PLACEMENT_3D ( 'NONE', #67, #8433, #10101 ) ;
#31288=CARTESIAN_POINT ( 'NONE',  ( 20.71343476517798621, 1522.906561336852974, 238.3377464195744722 ) ) ;
#31289=DIRECTION ( 'NONE',  ( 0.000000000000000000, 0.000000000000000000, 1.000000000000000000 ) ) ;
#31298=CYLINDRICAL_SURFACE ( 'NONE', #15808, 1.000000000000000888 ) ;
#31299=CARTESIAN_POINT ( 'NONE',  ( 3.316380893998936763, 1524.425415513988810, 176.3365459558180817 ) ) ;
#31322=EDGE_LOOP ( 'NONE', ( #31997, #72376, #27320, #11649, #96887 ) ) ;
#31331=AXIS2_PLACEMENT_3D ( 'NONE', #84302, #82659, #108964 ) ;
#31343=CARTESIAN_POINT ( 'NONE',  ( 2.038847259681869861, 1522.861859112239244, 173.3106345060298565 ) ) ;
#31344=DIRECTION ( 'NONE',  ( 0.000000000000000000, 1.000000000000000000, 0.000000000000000000 ) ) ;
#31353=CARTESIAN_POINT ( 'NONE',  ( 30.57821243133773947, 1525.253972588462602, 196.6735172117064110 ) ) ;
#31358=ORIENTED_EDGE ( 'NONE', *, *, #65951, .T. ) ;
#31368=CARTESIAN_POINT ( 'NONE',  ( 16.62350534370850141, 1524.082740465118604, 237.7032228575765771 ) ) ;
#31377=CARTESIAN_POINT ( 'NONE',  ( -21.86721050905262587, 1523.611961620354123, 235.0400593884483840 ) ) ;
#31380=CARTESIAN_POINT ( 'NONE',  ( 28.35863496383795379, 1526.382868172863937, 219.7167431890427451 ) ) ;
#31389=DIRECTION ( 'NONE',  ( 0.000000000000000000, 0.000000000000000000, -1.000000000000000000 ) ) ;
#31391=VERTEX_POINT ( 'NONE', #98106 ) ;
#31393=B_SPLINE_CURVE_WITH_KNOTS ( 'NONE', 3,
 ( #94696, #45427, #69533, #35908, #28599, #62800 ),
 .UNSPECIFIED., .F., .F.,
 ( 4, 2, 4 ),
 ( -1.285435071100343021E-05, 0.001079388306740753593, 0.002171630964192510903 ),
 .UNSPECIFIED. ) ;
#31399=CARTESIAN_POINT ( 'NONE',  ( -17.59770716511913591, 1524.659802833170716, 180.6838038464929639 ) ) ;
#31439=ORIENTED_EDGE ( 'NONE', *, *, #9351, .F. ) ;
#31441=DIRECTION ( 'NONE',  ( 0.03173147633655607619, -0.9969860201949453105, -0.07079540200709832920 ) ) ;
#31442=ORIENTED_EDGE ( 'NONE', *, *, #105511, .T. ) ;
#31444=AXIS2_PLACEMENT_3D ( 'NONE', #53347, #38172, #106484 ) ;
#31470=CARTESIAN_POINT ( 'NONE',  ( 30.15585515321759758, 1524.425415513990174, 222.4071264889503254 ) ) ;
#31471=DIRECTION ( 'NONE',  ( 0.2054769195713296581, 0.000000000000000000, -0.9786619618251632957 ) ) ;
#31489=EDGE_CURVE ( 'NONE', #42444, #63875, #38751, .T. ) ;
#31520=B_SPLINE_CURVE_WITH_KNOTS ( 'NONE', 3,
 ( #5082, #56605, #39233, #30833, #82893, #99125, #100252, #99675, #22404, #90741 ),
 .UNSPECIFIED., .F., .F.,
 ( 4, 2, 2, 2, 4 ),
 ( 1.734723475976807094E-17, 0.0007406479101619456874, 0.001481295820323874027, 0.002221943730485802584, 0.002962591640647730708 ),
 .UNSPECIFIED. ) ;
#31527=EDGE_CURVE ( 'NONE', #82581, #37235, #52685, .T. ) ;
#31547=CARTESIAN_POINT ( 'NONE',  ( 32.21030510514599143, 1524.412455883367329, 216.0988835363537817 ) ) ;
#31553=ORIENTED_EDGE ( 'NONE', *, *, #37734, .T. ) ;
#31560=CARTESIAN_POINT ( 'NONE',  ( 16.55384015339962289, 1524.739915903632209, 237.4556660764005471 ) ) ;
#31562=B_SPLINE_CURVE_WITH_KNOTS ( 'NONE', 3,
 ( #42709, #100931, #109371, #77413, #17464, #32649, #58413, #75761, #66826, #94758 ),
 .UNSPECIFIED., .F., .F.,
 ( 4, 2, 2, 2, 4 ),
 ( 3.469446951953614189E-18, 0.0007403986298595326620, 0.001480797259719061855, 0.002221195889578590939, 0.002961594519438120240 ),
 .UNSPECIFIED. ) ;
#31577=ORIENTED_EDGE ( 'NONE', *, *, #28913, .T. ) ;
#31586=( LENGTH_UNIT ( ) NAMED_UNIT ( * ) SI_UNIT ( .MILLI., .METRE. ) );
#31591=VERTEX_POINT ( 'NONE', #5197 ) ;
#31615=VERTEX_POINT ( 'NONE', #5763 ) ;
#31625=LINE ( 'NONE', #40583, #69686 ) ;
#31631=CARTESIAN_POINT ( 'NONE',  ( -2.640434834157888933, 1526.748660780343471, 176.9315852594522482 ) ) ;
#31636=CARTESIAN_POINT ( 'NONE',  ( 31.34137657907978891, 1523.481610118013123, 196.3411265156827596 ) ) ;
#31646=CARTESIAN_POINT ( 'NONE',  ( 30.51126001304326252, 1526.382868172863937, 219.8557927178086970 ) ) ;
#31647=ORIENTED_EDGE ( 'NONE', *, *, #3941, .F. ) ;
#31652=EDGE_CURVE ( 'NONE', #76248, #40736, #106348, .T. ) ;
#31653=CARTESIAN_POINT ( 'NONE',  ( -17.17241001986523941, 1512.187213306747481, 179.6185504016045797 ) ) ;
#31674=CARTESIAN_POINT ( 'NONE',  ( -16.66936639845670598, 1523.382868172864164, 180.4828114240741854 ) ) ;
#31681=CARTESIAN_POINT ( 'NONE',  ( 31.44837959398592986, 1511.187213306747708, 220.9083067115976462 ) ) ;
#31686=ORIENTED_EDGE ( 'NONE', *, *, #67288, .T. ) ;
#31692=EDGE_CURVE ( 'NONE', #49707, #29992, #33690, .T. ) ;
#31722=AXIS2_PLACEMENT_3D ( 'NONE', #109887, #25854, #102015 ) ;
#31731=B_SPLINE_CURVE_WITH_KNOTS ( 'NONE', 3,
 ( #94865, #36075, #77521, #821, #27664, #51208 ),
 .UNSPECIFIED., .F., .F.,
 ( 4, 2, 4 ),
 ( -1.131363979550832737E-05, 0.001067788114096722158, 0.002146889867988952330 ),
 .UNSPECIFIED. ) ;
#31754=FACE_OUTER_BOUND ( 'NONE', #88575, .T. ) ;
#31764=CARTESIAN_POINT ( 'NONE',  ( -3.350338079455601026, 1523.604703353109699, 242.0808062845893289 ) ) ;
#31775=TOROIDAL_SURFACE ( 'NONE', #53225, 1.000000000000000000, 1.000000000000000000 ) ;
#31777=FACE_OUTER_BOUND ( 'NONE', #72978, .T. ) ;
#31801=EDGE_CURVE ( 'NONE', #79144, #11721, #55425, .T. ) ;
#31805=CARTESIAN_POINT ( 'NONE',  ( -17.83486663330464950, 1523.678648413191695, 237.8759530894961074 ) ) ;
#31808=CARTESIAN_POINT ( 'NONE',  ( -16.69297358003335674, 1526.382868172864164, 234.5473741529612255 ) ) ;
#31817=ORIENTED_EDGE ( 'NONE', *, *, #100654, .T. ) ;
#31818=CARTESIAN_POINT ( 'NONE',  ( 34.09079054514135976, 1524.667648926078527, 217.9059385276705143 ) ) ;
#31825=CARTESIAN_POINT ( 'NONE',  ( -17.17241001986523941, 1512.187213306747481, 179.6185504016045797 ) ) ;
#31827=DIRECTION ( 'NONE',  ( -0.000000000000000000, -1.000000000000000000, -0.000000000000000000 ) ) ;
#31829=FACE_OUTER_BOUND ( 'NONE', #12975, .T. ) ;
#31834=DIRECTION ( 'NONE',  ( 0.7414773880254614813, 0.000000000000000000, -0.6709778558543786353 ) ) ;
#31844=DIRECTION ( 'NONE',  ( -1.040834085586083310E-14, 0.000000000000000000, 1.000000000000000000 ) ) ;
#31861=CARTESIAN_POINT ( 'NONE',  ( 22.08622291482350519, 1523.382868172864164, 233.8253038720783366 ) ) ;
#31875=ORIENTED_EDGE ( 'NONE', *, *, #102104, .T. ) ;
#31879=ORIENTED_EDGE ( 'NONE', *, *, #56752, .F. ) ;
#31882=CIRCLE ( 'NONE', #35492, 2.000000000000001776 ) ;
#31883=AXIS2_PLACEMENT_3D ( 'NONE', #91460, #5242, #66828 ) ;
#31886=CIRCLE ( 'NONE', #17561, 33.13701971169416538 ) ;
#31896=ORIENTED_EDGE ( 'NONE', *, *, #4958, .T. ) ;
#31920=CARTESIAN_POINT ( 'NONE',  ( 16.49514911236786219, 1525.343710797494396, 237.0302821690905546 ) ) ;
#31936=EDGE_CURVE ( 'NONE', #21237, #57810, #48742, .T. ) ;
#31952=FACE_OUTER_BOUND ( 'NONE', #18348, .T. ) ;
#31953=CARTESIAN_POINT ( 'NONE',  ( 2.620401159549908598, 1523.382868172863937, 176.0805060893157190 ) ) ;
#31959=AXIS2_PLACEMENT_3D ( 'NONE', #84322, #24938, #68106 ) ;
#31971=ORIENTED_EDGE ( 'NONE', *, *, #44604, .T. ) ;
#31997=ORIENTED_EDGE ( 'NONE', *, *, #11077, .F. ) ;
#32007=LINE ( 'NONE', #66741, #5338 ) ;
#32038=TOROIDAL_SURFACE ( 'NONE', #99959, 1.000000000000000000, 1.000000000000000000 ) ;
#32057=CARTESIAN_POINT ( 'NONE',  ( -21.83164632205553346, 1524.739915903632664, 233.6211154403027024 ) ) ;
#32060=( BOUNDED_SURFACE ( )  B_SPLINE_SURFACE ( 3, 2, ( 
 ( #54869, #52657, #105821 ),
 ( #97399, #70036, #1159 ),
 ( #96304, #87923, #70580 ),
 ( #69475, #11744, #78401 ),
 ( #104148, #27434, #11210 ),
 ( #26895, #61084, #20134 ),
 ( #88457, #61617, #95749 ),
 ( #87355, #10651, #78973 ),
 ( #14482, #22868, #56515 ),
 ( #107445, #82798, #66031 ) ),
 .UNSPECIFIED., .F., .F., .F. ) 
 B_SPLINE_SURFACE_WITH_KNOTS ( ( 4, 2, 2, 2, 4 ),
 ( 3, 3 ),
 ( 1.570796326794896558, 1.963495408493620697, 2.356194490192344837, 2.748893571891068976, 3.141592653589793116 ),
 ( 0.000000000000000000, 1.000000000000000000 ),
 .UNSPECIFIED. ) 
 GEOMETRIC_REPRESENTATION_ITEM ( )  RATIONAL_B_SPLINE_SURFACE ( (
 ( 1.000000000000000000, 0.7071067811865870967, 1.000000000000000000),
 ( 1.000000000000000000, 0.7166207884813499129, 1.000000000000000000),
 ( 1.000000000000000000, 0.7259222650918575326, 1.000000000000000000),
 ( 1.000000000000000000, 0.7428408967918733730, 1.000000000000000000),
 ( 1.000000000000000000, 0.7504512394537499187, 1.000000000000000000),
 ( 1.000000000000000000, 0.7630177051937450106, 1.000000000000000000),
 ( 1.000000000000000000, 0.7679730451964706939, 1.000000000000000000),
 ( 1.000000000000000000, 0.7746454561805765637, 1.000000000000000000),
 ( 1.000000000000000000, 0.7763684247028794783, 1.000000000000000000),
 ( 1.000000000000000000, 0.7763623250684325017, 1.000000000000000000) ) ) 
 REPRESENTATION_ITEM ( '' )  SURFACE ( )  );
#32061=DIRECTION ( 'NONE',  ( 0.000000000000000000, 1.000000000000000000, 0.000000000000000000 ) ) ;
#32063=EDGE_LOOP ( 'NONE', ( #88828, #48844, #58074, #46830 ) ) ;
#32064=CARTESIAN_POINT ( 'NONE',  ( -17.83486663330463173, 1523.678648413191922, 237.8759530894961358 ) ) ;
#32070=CARTESIAN_POINT ( 'NONE',  ( 16.73628186595820466, 1526.382868172864164, 184.0591879540915841 ) ) ;
#32108=CARTESIAN_POINT ( 'NONE',  ( 31.12456774391174008, 1525.960063244516959, 217.0912716842395582 ) ) ;
#32112=AXIS2_PLACEMENT_3D ( 'NONE', #107996, #74979, #40247 ) ;
#32116=LINE ( 'NONE', #14753, #7014 ) ;
#32121=CARTESIAN_POINT ( 'NONE',  ( 16.50400130224765149, 1525.907212628473644, 236.2546788475581252 ) ) ;
#32122=CIRCLE ( 'NONE', #91101, 1.000000000000085043 ) ;
#32164=EDGE_CURVE ( 'NONE', #106220, #3217, #105887, .T. ) ;
#32206=DIRECTION ( 'NONE',  ( 1.387778780781444413E-14, 0.000000000000000000, 1.000000000000000000 ) ) ;
#32208=CARTESIAN_POINT ( 'NONE',  ( 32.41382812665953139, 1525.581535527370988, 220.2604433702309734 ) ) ;
#32223=EDGE_CURVE ( 'NONE', #95777, #74589, #69264, .T. ) ;
#32226=CARTESIAN_POINT ( 'NONE',  ( 20.21716934225348439, 1526.104292489126465, 184.5497256588712105 ) ) ;
#32256=EDGE_CURVE ( 'NONE', #32684, #43726, #64825, .T. ) ;
#32274=AXIS2_PLACEMENT_3D ( 'NONE', #48119, #13932, #82258 ) ;
#32282=VERTEX_POINT ( 'NONE', #93874 ) ;
#32288=CARTESIAN_POINT ( 'NONE',  ( -2.470168521978398424, 1523.382868172864164, 175.3649660270905315 ) ) ;
#32289=EDGE_CURVE ( 'NONE', #108583, #82581, #98752, .T. ) ;
#32296=EDGE_CURVE ( 'NONE', #40624, #35166, #26673, .T. ) ;
#32303=AXIS2_PLACEMENT_3D ( 'NONE', #36536, #46619, #62324 ) ;
#32310=CARTESIAN_POINT ( 'NONE',  ( -28.72841836130151805, 1526.333389947941441, 220.1290250959031596 ) ) ;
#32323=EDGE_LOOP ( 'NONE', ( #9633, #80343, #101392 ) ) ;
#32343=ORIENTED_EDGE ( 'NONE', *, *, #52925, .T. ) ;
#32349=CARTESIAN_POINT ( 'NONE',  ( -17.15830831501837039, 1512.187213306747481, 209.3391145445735333 ) ) ;
#32355=CARTESIAN_POINT ( 'NONE',  ( -17.17241001986523941, 1512.187213306747481, 180.6185504016045797 ) ) ;
#32373=EDGE_CURVE ( 'NONE', #105990, #90799, #21831, .T. ) ;
#32374=LINE ( 'NONE', #17179, #19604 ) ;
#32377=VERTEX_POINT ( 'NONE', #28344 ) ;
#32378=CARTESIAN_POINT ( 'NONE',  ( 32.36284091029084209, 1525.878013734320120, 218.9814869512333075 ) ) ;
#32390=CARTESIAN_POINT ( 'NONE',  ( -21.53712143570537663, 1523.621879633028584, 234.3036048850999578 ) ) ;
#32400=CARTESIAN_POINT ( 'NONE',  ( -21.59396340175319651, 1525.159196711359755, 184.7447238809834857 ) ) ;
#32402=( BOUNDED_CURVE ( )  B_SPLINE_CURVE ( 3, ( #12009, #80870, #107719, #99294 ),
 .UNSPECIFIED., .F., .F. ) 
 B_SPLINE_CURVE_WITH_KNOTS ( ( 4, 4 ),
 ( 2.436781329611983793, 3.141592653589793116 ),
 .UNSPECIFIED. ) 
 CURVE ( )  GEOMETRIC_REPRESENTATION_ITEM ( )  RATIONAL_B_SPLINE_CURVE ( ( 1.000000000000000000, 0.9590300661663088144, 0.9590300661663088144, 1.000000000000000000 ) ) 
 REPRESENTATION_ITEM ( '' )  );
#32413=CARTESIAN_POINT ( 'NONE',  ( 32.02808312589922224, 1511.187213306747708, 220.9649204700462235 ) ) ;
#32415=EDGE_CURVE ( 'NONE', #100609, #17148, #79119, .T. ) ;
#32422=VECTOR ( 'NONE', #69170, 1000.000000000000000 ) ;
#32439=CARTESIAN_POINT ( 'NONE',  ( 2.038646110889678287, 1525.960063244516959, 177.0579350083066004 ) ) ;
#32456=VECTOR ( 'NONE', #20865, 1000.000000000000000 ) ;
#32478=EDGE_LOOP ( 'NONE', ( #87827, #39854, #33602, #69708 ) ) ;
#32489=CARTESIAN_POINT ( 'NONE',  ( 17.83486663330486621, 1523.678648413191695, 180.3677388339000061 ) ) ;
#32505=CARTESIAN_POINT ( 'NONE',  ( -0.4151546846839010985, 1522.906561336850928, 173.3106345060153046 ) ) ;
#32517=CARTESIAN_POINT ( 'NONE',  ( -17.50735355147196515, 1524.972613296805548, 180.8654324079905393 ) ) ;
#32525=DIRECTION ( 'NONE',  ( -0.000000000000000000, -1.000000000000000000, -0.000000000000000000 ) ) ;
#32527=CARTESIAN_POINT ( 'NONE',  ( -17.44374831407654725, 1524.130440953581001, 237.5220222273293302 ) ) ;
#32547=FACE_OUTER_BOUND ( 'NONE', #65637, .T. ) ;
#32555=VERTEX_POINT ( 'NONE', #56864 ) ;
#32557=ORIENTED_EDGE ( 'NONE', *, *, #51072, .T. ) ;
#32564=VECTOR ( 'NONE', #67221, 1000.000000000000000 ) ;
#32588=CARTESIAN_POINT ( 'NONE',  ( 29.74902317390491646, 1525.343710797494623, 222.0046397572924377 ) ) ;
#32615=CARTESIAN_POINT ( 'NONE',  ( -21.55808852496470962, 1523.844789899204443, 234.2610814835831547 ) ) ;
#32635=CARTESIAN_POINT ( 'NONE',  ( -32.86802468386279941, 1523.382868172864164, 217.2040256693919957 ) ) ;
#32649=CARTESIAN_POINT ( 'NONE',  ( 21.32683180188249139, 1525.211477436245787, 234.3841140920684722 ) ) ;
#32658=CARTESIAN_POINT ( 'NONE',  ( -16.62351968733423391, 1524.082582765195411, 237.7032314130105703 ) ) ;
#32669=DIRECTION ( 'NONE',  ( 0.000000000000000000, 0.000000000000000000, -1.000000000000000000 ) ) ;
#32671=CARTESIAN_POINT ( 'NONE',  ( 17.22627284987205698, 1525.856065479249082, 236.4663881609581892 ) ) ;
#32674=CARTESIAN_POINT ( 'NONE',  ( 32.38114538885250226, 1523.604703353109699, 202.1233279672528624 ) ) ;
#32684=VERTEX_POINT ( 'NONE', #49572 ) ;
#32697=( NAMED_UNIT ( * ) PLANE_ANGLE_UNIT ( ) SI_UNIT ( $, .RADIAN. ) );
#32713=DIRECTION ( 'NONE',  ( 0.000000000000000000, 1.000000000000000000, 0.000000000000000000 ) ) ;
#32726=ORIENTED_EDGE ( 'NONE', *, *, #21547, .F. ) ;
#32739=CARTESIAN_POINT ( 'NONE',  ( 17.61566626013499004, 1524.599984580802129, 180.6473472415456456 ) ) ;
#32745=CARTESIAN_POINT ( 'NONE',  ( 32.97913964219439720, 1511.187213306747708, 220.2739374644211807 ) ) ;
#32754=ORIENTED_EDGE ( 'NONE', *, *, #48262, .T. ) ;
#32759=FACE_OUTER_BOUND ( 'NONE', #18400, .T. ) ;
#32768=CARTESIAN_POINT ( 'NONE',  ( 18.66420869458043441, 1526.382868172864164, 185.4599087859680537 ) ) ;
#32790=CARTESIAN_POINT ( 'NONE',  ( -18.66420869458028520, 1526.382868172864164, 232.7837831374281166 ) ) ;
#32804=VERTEX_POINT ( 'NONE', #85341 ) ;
#32820=VERTEX_POINT ( 'NONE', #15383 ) ;
#32838=VERTEX_POINT ( 'NONE', #33847 ) ;
#32853=ORIENTED_EDGE ( 'NONE', *, *, #65808, .F. ) ;
#32858=CARTESIAN_POINT ( 'NONE',  ( -3.351013500467394213, 1524.082740465118604, 242.0157168755361852 ) ) ;
#32870=CARTESIAN_POINT ( 'NONE',  ( 0.000000000000000000, 1523.051704408389696, 185.4225825198192013 ) ) ;
#32880=CARTESIAN_POINT ( 'NONE',  ( 2.038646110889595242, 1525.960063244516959, 177.0579350083065435 ) ) ;
#32890=VERTEX_POINT ( 'NONE', #45461 ) ;
#32898=CARTESIAN_POINT ( 'NONE',  ( -31.32995031131184760, 1523.678648413191695, 221.9013357025048663 ) ) ;
#32908=ORIENTED_EDGE ( 'NONE', *, *, #66546, .F. ) ;
#32923=CARTESIAN_POINT ( 'NONE',  ( -32.38845791999490586, 1523.456872492435195, 216.1254071228449902 ) ) ;
#32925=CARTESIAN_POINT ( 'NONE',  ( -29.73374635647653008, 1526.349689584397083, 201.0212862843677613 ) ) ;
#32927=CARTESIAN_POINT ( 'NONE',  ( -33.36586802512168504, 1512.187213306747481, 216.3367586934473366 ) ) ;
#32938=CARTESIAN_POINT ( 'NONE',  ( 29.40443212115394189, 1512.187213306747481, 222.0897836382243042 ) ) ;
#32968=CARTESIAN_POINT ( 'NONE',  ( 33.28034951413924603, 1522.382868172863937, 200.8029765415137433 ) ) ;
#32982=CARTESIAN_POINT ( 'NONE',  ( 18.02257621027576917, 1526.382868172863937, 182.8951942368371988 ) ) ;
#32984=ORIENTED_EDGE ( 'NONE', *, *, #57111, .F. ) ;
#32997=AXIS2_PLACEMENT_3D ( 'NONE', #100071, #101153, #59738 ) ;
#32999=CARTESIAN_POINT ( 'NONE',  ( 30.95265250778348687, 1524.659148609483054, 196.4584948516175302 ) ) ;
#33033=CARTESIAN_POINT ( 'NONE',  ( -2.580915939757335131, 1524.130440953581001, 175.8924427158433161 ) ) ;
#33034=CIRCLE ( 'NONE', #52735, 0.9999999999999898970 ) ;
#33039=( BOUNDED_SURFACE ( )  B_SPLINE_SURFACE ( 3, 2, ( 
 ( #110702, #57571, #14970 ),
 ( #96675, #51914, #61992 ),
 ( #43516, #9896, #86057 ),
 ( #103957, #10451, #45182 ),
 ( #53026, #79323, #26690 ),
 ( #60886, #2634, #87733 ),
 ( #78204, #44065, #36760 ),
 ( #9354, #78765, #69838 ),
 ( #70954, #8780, #69278 ),
 ( #95013, #105069, #27810 ) ),
 .UNSPECIFIED., .F., .F., .F. ) 
 B_SPLINE_SURFACE_WITH_KNOTS ( ( 4, 2, 2, 2, 4 ),
 ( 3, 3 ),
 ( 1.570796326794896558, 1.963495408493620697, 2.356194490192344837, 2.748893571891068976, 3.141592653589793116 ),
 ( 0.000000000000000000, 1.000000000000000000 ),
 .UNSPECIFIED. ) 
 GEOMETRIC_REPRESENTATION_ITEM ( )  RATIONAL_B_SPLINE_SURFACE ( (
 ( 1.000000000000000000, 0.7071067811865867636, 1.000000000000000000),
 ( 1.000000000000000000, 0.7166207884820130491, 1.000000000000000000),
 ( 1.000000000000000000, 0.7259222650909733510, 1.000000000000000000),
 ( 1.000000000000000000, 0.7428408967927655482, 1.000000000000000000),
 ( 1.000000000000000000, 0.7504512394527111940, 1.000000000000000000),
 ( 1.000000000000000000, 0.7630177051947926170, 1.000000000000000000),
 ( 1.000000000000000000, 0.7679730451972418548, 1.000000000000000000),
 ( 1.000000000000000000, 0.7746454561798022942, 1.000000000000000000),
 ( 1.000000000000000000, 0.7763684247034656760, 1.000000000000000000),
 ( 1.000000000000000000, 0.7763623250684373867, 1.000000000000000000) ) ) 
 REPRESENTATION_ITEM ( '' )  SURFACE ( )  );
#33053=PLANE ( 'NONE',  #66023 ) ;
#33055=ADVANCED_FACE ( 'NONE', ( #92252 ), #57701, .T. ) ;
#33058=LINE ( 'NONE', #60498, #84338 ) ;
#33061=CARTESIAN_POINT ( 'NONE',  ( -19.07966196791873159, 1524.244163922424377, 239.0023935151694161 ) ) ;
#33081=ADVANCED_FACE ( 'NONE', ( #5493 ), #106006, .F. ) ;
#33086=AXIS2_PLACEMENT_3D ( 'NONE', #46572, #88566, #46023 ) ;
#33091=ORIENTED_EDGE ( 'NONE', *, *, #90698, .T. ) ;
#33094=CARTESIAN_POINT ( 'NONE',  ( -32.78250617288048829, 1511.187213306747708, 199.9357095655695389 ) ) ;
#33117=DIRECTION ( 'NONE',  ( 0.000000000000000000, 1.000000000000000000, 0.000000000000000000 ) ) ;
#33121=AXIS2_PLACEMENT_3D ( 'NONE', #36771, #55802, #97218 ) ;
#33153=CARTESIAN_POINT ( 'NONE',  ( -30.90487439922565116, 1525.907212628473644, 201.8101144455181952 ) ) ;
#33168=ORIENTED_EDGE ( 'NONE', *, *, #96685, .T. ) ;
#33174=CIRCLE ( 'NONE', #31331, 0.9999999999999873435 ) ;
#33191=CARTESIAN_POINT ( 'NONE',  ( -30.41961987998705297, 1524.374578187332872, 196.3903468980581977 ) ) ;
#33208=CARTESIAN_POINT ( 'NONE',  ( 17.10350668511487626, 1524.477587234284556, 180.9723570393801708 ) ) ;
#33214=CARTESIAN_POINT ( 'NONE',  ( 17.83486663330510424, 1523.678648413191695, 237.8759530894958516 ) ) ;
#33224=ADVANCED_FACE ( 'NONE', ( #8231 ), #85485, .T. ) ;
#33228=ORIENTED_EDGE ( 'NONE', *, *, #81444, .F. ) ;
#33240=CARTESIAN_POINT ( 'NONE',  ( 2.902322711624676882E-15, 1524.090675761330203, 185.4225825198192013 ) ) ;
#33252=DIRECTION ( 'NONE',  ( 0.000000000000000000, 0.000000000000000000, 1.000000000000000000 ) ) ;
#33297=DIRECTION ( 'NONE',  ( 0.000000000000000000, 0.000000000000000000, -1.000000000000000000 ) ) ;
#33299=CARTESIAN_POINT ( 'NONE',  ( -34.18677586421132730, 1522.906561336852519, 219.7932833225229388 ) ) ;
#33311=ORIENTED_EDGE ( 'NONE', *, *, #38519, .F. ) ;
#33334=CARTESIAN_POINT ( 'NONE',  ( -19.00259723423865665, 1526.382868172570852, 232.9129335399678098 ) ) ;
#33350=ORIENTED_EDGE ( 'NONE', *, *, #11102, .F. ) ;
#33367=DIRECTION ( 'NONE',  ( -0.4090087482554183862, -0.000000000000000000, 0.9125304618754026542 ) ) ;
#33368=ORIENTED_EDGE ( 'NONE', *, *, #108894, .T. ) ;
#33376=CARTESIAN_POINT ( 'NONE',  ( 22.74803453391460906, 1523.678648413191695, 234.5603111028696901 ) ) ;
#33382=DIRECTION ( 'NONE',  ( 0.000000000000000000, 0.000000000000000000, 1.000000000000000000 ) ) ;
#33402=ORIENTED_EDGE ( 'NONE', *, *, #74787, .T. ) ;
#33406=CARTESIAN_POINT ( 'NONE',  ( 17.83486663330506872, 1523.678648413191695, 237.8759530894958800 ) ) ;
#33420=CARTESIAN_POINT ( 'NONE',  ( 32.28466283162151029, 1512.187213306747481, 199.0684425896244250 ) ) ;
#33421=CARTESIAN_POINT ( 'NONE',  ( 2.311636021096358018, 1525.506916460682305, 176.4384780102049035 ) ) ;
#33423=FACE_OUTER_BOUND ( 'NONE', #66621, .T. ) ;
#33438=CARTESIAN_POINT ( 'NONE',  ( -1.191524307911311809, 1526.382868172863937, 179.0083900503167911 ) ) ;
#33442=B_SPLINE_CURVE_WITH_KNOTS ( 'NONE', 3,
 ( #44827, #26328, #77856, #80488, #72116, #106231, #29517, #63707, #4336, #97818 ),
 .UNSPECIFIED., .F., .F.,
 ( 4, 2, 2, 2, 4 ),
 ( 0.000000000000000000, 0.0007189769279725889304, 0.001437953855945177861, 0.002156930783917766683, 0.002875907711890355722 ),
 .UNSPECIFIED. ) ;
#33443=PLANE ( 'NONE',  #98735 ) ;
#33451=CARTESIAN_POINT ( 'NONE',  ( 33.17484411121481713, 1525.713797967457140, 217.3801513758794215 ) ) ;
#33454=VERTEX_POINT ( 'NONE', #45744 ) ;
#33458=CARTESIAN_POINT ( 'NONE',  ( 17.83486663330486621, 1523.678648413191695, 180.3677388339000061 ) ) ;
#33469=DIRECTION ( 'NONE',  ( 0.2054769195713296304, 0.000000000000000000, -0.9786619618251631847 ) ) ;
#33471=CIRCLE ( 'NONE', #105039, 1.000000000000000888 ) ;
#33473=EDGE_LOOP ( 'NONE', ( #49198, #657, #95671, #100733 ) ) ;
#33496=ORIENTED_EDGE ( 'NONE', *, *, #30950, .T. ) ;
#33498=CARTESIAN_POINT ( 'NONE',  ( -3.017174818680797177, 1525.408337840050081, 176.9098480759781182 ) ) ;
#33503=DIRECTION ( 'NONE',  ( 1.788933584601080738E-15, 0.000000000000000000, 1.000000000000000000 ) ) ;
#33509=ORIENTED_EDGE ( 'NONE', *, *, #75298, .F. ) ;
#33528=VERTEX_POINT ( 'NONE', #95566 ) ;
#33532=EDGE_CURVE ( 'NONE', #9564, #87392, #48507, .T. ) ;
#33539=CARTESIAN_POINT ( 'NONE',  ( 30.38288201977627878, 1524.477587234266139, 196.4016200325754369 ) ) ;
#33540=LINE ( 'NONE', #84516, #93775 ) ;
#33545=CARTESIAN_POINT ( 'NONE',  ( 2.340423001224530619, 1525.425686270222059, 241.8895327159822841 ) ) ;
#33564=CARTESIAN_POINT ( 'NONE',  ( 2.470168521978398868, 1501.977400791986611, 242.8787258963054683 ) ) ;
#33566=EDGE_CURVE ( 'NONE', #8681, #43690, #52098, .T. ) ;
#33581=FACE_OUTER_BOUND ( 'NONE', #7362, .T. ) ;
#33594=VECTOR ( 'NONE', #29772, 1000.000000000000000 ) ;
#33602=ORIENTED_EDGE ( 'NONE', *, *, #13996, .T. ) ;
#33616=DIRECTION ( 'NONE',  ( 0.000000000000000000, 0.000000000000000000, -1.000000000000000000 ) ) ;
#33629=EDGE_LOOP ( 'NONE', ( #18136, #54652, #104041, #21362 ) ) ;
#33638=CARTESIAN_POINT ( 'NONE',  ( -17.84054676580458221, 1523.580203803270933, 180.3625987673426607 ) ) ;
#33646=B_SPLINE_CURVE_WITH_KNOTS ( 'NONE', 3,
 ( #87163, #103385, #2635, #11012, #36761, #36211, #60887, #68729, #51915, #95014 ),
 .UNSPECIFIED., .F., .F.,
 ( 4, 2, 2, 2, 4 ),
 ( 3.469446951953614189E-18, 0.0007406479101618190525, 0.001481295820323634636, 0.002221943730485450436, 0.002962591640647265802 ),
 .UNSPECIFIED. ) ;
#33659=EDGE_CURVE ( 'NONE', #74525, #17686, #96775, .T. ) ;
#33661=CARTESIAN_POINT ( 'NONE',  ( -2.472529913803013013, 1523.678648413191695, 242.8674788698241684 ) ) ;
#33669=ORIENTED_EDGE ( 'NONE', *, *, #22303, .T. ) ;
#33687=EDGE_CURVE ( 'NONE', #45131, #82569, #68260, .T. ) ;
#33690=LINE ( 'NONE', #17985, #11172 ) ;
#33713=CARTESIAN_POINT ( 'NONE',  ( -19.53786426059057746, 1512.187213306747481, 180.5239794925695946 ) ) ;
#33716=AXIS2_PLACEMENT_3D ( 'NONE', #41089, #75266, #13109 ) ;
#33721=AXIS2_PLACEMENT_3D ( 'NONE', #26829, #72704, #21150 ) ;
#33737=AXIS2_PLACEMENT_3D ( 'NONE', #92746, #60269, #50752 ) ;
#33743=ADVANCED_FACE ( 'NONE', ( #48917 ), #98738, .F. ) ;
#33745=CARTESIAN_POINT ( 'NONE',  ( -18.66420869458074705, 1526.382868172864164, 185.4599087859683095 ) ) ;
#33759=LINE ( 'NONE', #61766, #9293 ) ;
#33767=CARTESIAN_POINT ( 'NONE',  ( -30.61611611309821157, 1526.069472839380751, 201.6871119896482867 ) ) ;
#33788=DIRECTION ( 'NONE',  ( 1.139346649588226023E-16, 0.3666799630584695047, -0.9303471420343265574 ) ) ;
#33797=ADVANCED_FACE ( 'NONE', ( #84422 ), #43202, .T. ) ;
#33798=ORIENTED_EDGE ( 'NONE', *, *, #47269, .F. ) ;
#33812=ORIENTED_EDGE ( 'NONE', *, *, #75677, .T. ) ;
#33827=CARTESIAN_POINT ( 'NONE',  ( 21.86721050905282482, 1523.611961620354123, 183.2036325349477579 ) ) ;
#33831=EDGE_CURVE ( 'NONE', #79801, #13899, #49059, .T. ) ;
#33847=CARTESIAN_POINT ( 'NONE',  ( -31.92108011125334954, 1511.187213306747708, 220.9591791661900686 ) ) ;
#33863=AXIS2_PLACEMENT_3D ( 'NONE', #30459, #3092, #64643 ) ;
#33867=CARTESIAN_POINT ( 'NONE',  ( -21.30909630337585270, 1524.964158026965606, 184.3255832943751784 ) ) ;
#33871=CARTESIAN_POINT ( 'NONE',  ( -32.78250617288048829, 1511.187213306747708, 199.9357095655695389 ) ) ;
#33880=CARTESIAN_POINT ( 'NONE',  ( 16.64685983873516761, 1523.847233649538339, 180.5000230624021640 ) ) ;
#33899=CARTESIAN_POINT ( 'NONE',  ( -0.5770119038902407071, 1525.581535527370761, 243.3912443123663820 ) ) ;
#33909=B_SPLINE_CURVE_WITH_KNOTS ( 'NONE', 3,
 ( #31674, #41190, #66416, #75361 ),
 .UNSPECIFIED., .F., .F.,
 ( 4, 4 ),
 ( 0.000000000000000000, 0.0002220129587134778018 ),
 .UNSPECIFIED. ) ;
#33924=CARTESIAN_POINT ( 'NONE',  ( 2.356894939219843721, 1525.394081235439444, 241.9297540029686786 ) ) ;
#33929=DIRECTION ( 'NONE',  ( 0.3090169943749582204, -0.000000000000000000, 0.9510565162951500895 ) ) ;
#33935=ORIENTED_EDGE ( 'NONE', *, *, #34595, .T. ) ;
#33948=AXIS2_PLACEMENT_3D ( 'NONE', #11505, #55177, #64126 ) ;
#33965=CARTESIAN_POINT ( 'NONE',  ( 2.472529913803023227, 1523.678648413191695, 242.8674788698241400 ) ) ;
#33973=CARTESIAN_POINT ( 'NONE',  ( -16.51370628721510769, 1525.137881624908914, 237.1983654728897477 ) ) ;
#33976=DIRECTION ( 'NONE',  ( -0.5877852522924820189, 0.000000000000000000, -0.8090169943749410120 ) ) ;
#33985=ADVANCED_FACE ( 'NONE', ( #48508 ), #38966, .T. ) ;
#33991=CARTESIAN_POINT ( 'NONE',  ( 2.340429037510286747, 1525.425665131969026, 176.3541395084411079 ) ) ;
#33992=DIRECTION ( 'NONE',  ( 0.4978433412588781914, 0.000000000000000000, 0.8672669759446606230 ) ) ;
#33997=FACE_OUTER_BOUND ( 'NONE', #16309, .T. ) ;
#34003=ORIENTED_EDGE ( 'NONE', *, *, #106857, .F. ) ;
#34017=DIRECTION ( 'NONE',  ( 0.000000000000000000, 0.000000000000000000, -1.000000000000000000 ) ) ;
#34020=CARTESIAN_POINT ( 'NONE',  ( 33.05665451062220228, 1523.390106123591067, 217.3123061710359423 ) ) ;
#34024=ORIENTED_EDGE ( 'NONE', *, *, #23975, .T. ) ;
#34025=ORIENTED_EDGE ( 'NONE', *, *, #99506, .F. ) ;
#34031=DIRECTION ( 'NONE',  ( -0.9510565162951518658, 0.000000000000000000, 0.3090169943749528914 ) ) ;
#34035=CARTESIAN_POINT ( 'NONE',  ( -21.54116136303244389, 1523.462669333492613, 234.3126182784949947 ) ) ;
#34047=CARTESIAN_POINT ( 'NONE',  ( -20.70484064406422320, 1525.907212628473644, 185.0411015109855839 ) ) ;
#34062=ORIENTED_EDGE ( 'NONE', *, *, #59929, .F. ) ;
#34064=AXIS2_PLACEMENT_3D ( 'NONE', #92973, #77299, #59406 ) ;
#34072=CARTESIAN_POINT ( 'NONE',  ( -3.177699364621945133, 1525.042337199240137, 176.6379248602500525 ) ) ;
#34100=AXIS2_PLACEMENT_3D ( 'NONE', #15458, #51285, #83785 ) ;
#34105=EDGE_CURVE ( 'NONE', #71856, #32890, #43408, .T. ) ;
#34119=CARTESIAN_POINT ( 'NONE',  ( -32.86802468386296994, 1523.382868172864164, 201.0396662540046577 ) ) ;
#34122=CARTESIAN_POINT ( 'NONE',  ( 31.99468309217332873, 1524.860077346004573, 202.1252391477154617 ) ) ;
#34129=DIRECTION ( 'NONE',  ( 0.1070030146457237041, 0.000000000000000000, -0.9942586961433764747 ) ) ;
#34141=CIRCLE ( 'NONE', #3724, 2.000000000000001776 ) ;
#34164=CARTESIAN_POINT ( 'NONE',  ( -22.03465957474533354, 1522.382868172863937, 235.4136513321633117 ) ) ;
#34179=ADVANCED_FACE ( 'NONE', ( #77012 ), #14496, .T. ) ;
#34191=CARTESIAN_POINT ( 'NONE',  ( -30.37359097063588109, 1526.143142182216252, 216.9284661788367998 ) ) ;
#34218=ORIENTED_EDGE ( 'NONE', *, *, #65041, .F. ) ;
#34226=CARTESIAN_POINT ( 'NONE',  ( -2.621078202464676821, 1523.542365884047513, 242.1599611597541752 ) ) ;
#34227=CARTESIAN_POINT ( 'NONE',  ( 21.38516915557986309, 1512.187213306747481, 237.8497028174237471 ) ) ;
#34267=DIRECTION ( 'NONE',  ( -0.4090087482554383147, 0.000000000000000000, -0.9125304618753937724 ) ) ;
#34269=DIRECTION ( 'NONE',  ( 0.000000000000000000, 0.000000000000000000, -1.000000000000000000 ) ) ;
#34277=ORIENTED_EDGE ( 'NONE', *, *, #67242, .T. ) ;
#34286=CARTESIAN_POINT ( 'NONE',  ( -33.93019615848938031, 1524.726013923371283, 220.5829544587965927 ) ) ;
#34290=CARTESIAN_POINT ( 'NONE',  ( 17.84338787571921614, 1512.187213306747481, 180.3600277896298110 ) ) ;
#34305=DIRECTION ( 'NONE',  ( 0.000000000000000000, 0.000000000000000000, -1.000000000000000000 ) ) ;
#34306=CARTESIAN_POINT ( 'NONE',  ( -17.19739463999666285, 1525.960063244516959, 181.9833109756550584 ) ) ;
#34320=CARTESIAN_POINT ( 'NONE',  ( 17.12670006681583246, 1524.374142163904253, 180.9415281674935443 ) ) ;
#34328=EDGE_CURVE ( 'NONE', #49199, #22340, #103952, .T. ) ;
#34338=ORIENTED_EDGE ( 'NONE', *, *, #56744, .F. ) ;
#34341=CARTESIAN_POINT ( 'NONE',  ( 20.88378052024278020, 1525.556089352344770, 184.5817669221027586 ) ) ;
#34346=( BOUNDED_CURVE ( )  B_SPLINE_CURVE ( 3, ( #6207, #4570, #14603, #22426 ),
 .UNSPECIFIED., .F., .F. ) 
 B_SPLINE_CURVE_WITH_KNOTS ( ( 4, 4 ),
 ( 2.436781329611989122, 3.141592653589793116 ),
 .UNSPECIFIED. ) 
 CURVE ( )  GEOMETRIC_REPRESENTATION_ITEM ( )  RATIONAL_B_SPLINE_CURVE ( ( 1.000000000000000000, 0.9590300661663093695, 0.9590300661663093695, 1.000000000000000000 ) ) 
 REPRESENTATION_ITEM ( '' )  );
#34369=DIRECTION ( 'NONE',  ( 0.000000000000000000, 0.000000000000000000, 1.000000000000000000 ) ) ;
#34387=CARTESIAN_POINT ( 'NONE',  ( -20.20959865099510111, 1511.187213306747708, 182.0120230947222524 ) ) ;
#34390=CARTESIAN_POINT ( 'NONE',  ( 21.61975802671112135, 1524.130440953581001, 183.7557183496562061 ) ) ;
#34401=EDGE_LOOP ( 'NONE', ( #35444, #84732, #32754, #11992 ) ) ;
#34417=DIRECTION ( 'NONE',  ( 0.000000000000000000, 0.000000000000000000, 1.000000000000000000 ) ) ;
#34429=CARTESIAN_POINT ( 'NONE',  ( -20.70484064406419122, 1525.907212628473644, 185.0411015109856692 ) ) ;
#34471=VERTEX_POINT ( 'NONE', #33406 ) ;
#34493=CARTESIAN_POINT ( 'NONE',  ( -21.63731731441981410, 1524.599984580802129, 183.5692477652812329 ) ) ;
#34507=EDGE_LOOP ( 'NONE', ( #48534, #45108, #3565 ) ) ;
#34522=ORIENTED_EDGE ( 'NONE', *, *, #100179, .T. ) ;
#34539=ORIENTED_EDGE ( 'NONE', *, *, #22731, .T. ) ;
#34542=CARTESIAN_POINT ( 'NONE',  ( 2.385609062334842712, 1525.697947650493916, 177.1458780446492653 ) ) ;
#34550=CARTESIAN_POINT ( 'NONE',  ( 17.29882006758224122, 1523.542365884046376, 180.8528181918412940 ) ) ;
#34587=EDGE_CURVE ( 'NONE', #40948, #83491, #287, .T. ) ;
#34589=DIRECTION ( 'NONE',  ( -0.000000000000000000, -1.000000000000000000, 0.000000000000000000 ) ) ;
#34595=EDGE_CURVE ( 'NONE', #7480, #73940, #45080, .T. ) ;
#34623=ORIENTED_EDGE ( 'NONE', *, *, #265, .T. ) ;
#34654=DIRECTION ( 'NONE',  ( 0.000000000000000000, 1.000000000000000000, 0.000000000000000000 ) ) ;
#34706=CARTESIAN_POINT ( 'NONE',  ( -31.81424859196000909, 1524.964230758882877, 216.6572717949418347 ) ) ;
#34707=DIRECTION ( 'NONE',  ( 0.6709778558543747495, 0.000000000000000000, 0.7414773880254650340 ) ) ;
#34723=EDGE_LOOP ( 'NONE', ( #78845, #66223, #21808 ) ) ;
#34728=CARTESIAN_POINT ( 'NONE',  ( -33.36586802512168504, 1518.913060387330006, 216.3367586934473366 ) ) ;
#34737=DIRECTION ( 'NONE',  ( -0.000000000000000000, -1.000000000000000000, -0.000000000000000000 ) ) ;
#34776=ORIENTED_EDGE ( 'NONE', *, *, #102955, .F. ) ;
#34788=ORIENTED_EDGE ( 'NONE', *, *, #62600, .T. ) ;
#34809=ORIENTED_EDGE ( 'NONE', *, *, #65082, .T. ) ;
#34848=LINE ( 'NONE', #43266, #108148 ) ;
#34851=CARTESIAN_POINT ( 'NONE',  ( 32.85805783624304155, 1523.678648413191695, 201.0453875934054508 ) ) ;
#34860=CARTESIAN_POINT ( 'NONE',  ( -16.57584690634401170, 1524.538969332612623, 237.5592196072092008 ) ) ;
#34861=CARTESIAN_POINT ( 'NONE',  ( 32.97913964219439720, 1512.187213306747481, 220.2739374644211807 ) ) ;
#34869=CARTESIAN_POINT ( 'NONE',  ( 17.50742245788203988, 1524.972383263452912, 180.8652753437762897 ) ) ;
#34886=ORIENTED_EDGE ( 'NONE', *, *, #79151, .F. ) ;
#34889=ORIENTED_EDGE ( 'NONE', *, *, #36788, .T. ) ;
#34891=AXIS2_PLACEMENT_3D ( 'NONE', #68382, #59978, #19029 ) ;
#34934=CARTESIAN_POINT ( 'NONE',  ( 30.60461244942486303, 1523.621879633029039, 221.8232741897817277 ) ) ;
#34943=CARTESIAN_POINT ( 'NONE',  ( 30.29139560038433743, 1523.843271061948371, 222.4926161930171418 ) ) ;
#34967=DIRECTION ( 'NONE',  ( 0.000000000000000000, 1.000000000000000000, 0.000000000000000000 ) ) ;
#34973=FACE_OUTER_BOUND ( 'NONE', #66159, .T. ) ;
#34976=DIRECTION ( 'NONE',  ( 0.000000000000000000, 0.000000000000000000, -1.000000000000000000 ) ) ;
#34985=CARTESIAN_POINT ( 'NONE',  ( 30.80549360313082374, 1524.130440953581001, 196.3987987232744956 ) ) ;
#34993=( BOUNDED_CURVE ( )  B_SPLINE_CURVE ( 3, ( #63116, #37877, #88824, #36217 ),
 .UNSPECIFIED., .F., .F. ) 
 B_SPLINE_CURVE_WITH_KNOTS ( ( 4, 4 ),
 ( 4.712388980384689674, 6.283185307179586232 ),
 .UNSPECIFIED. ) 
 CURVE ( )  GEOMETRIC_REPRESENTATION_ITEM ( )  RATIONAL_B_SPLINE_CURVE ( ( 1.000000000000000000, 0.8047378541243649375, 0.8047378541243649375, 1.000000000000000000 ) ) 
 REPRESENTATION_ITEM ( '' )  );
#34999=ORIENTED_EDGE ( 'NONE', *, *, #17890, .T. ) ;
#35012=CARTESIAN_POINT ( 'NONE',  ( -3.350338079455601026, 1523.604703353109699, 242.0808062845893289 ) ) ;
#35022=CARTESIAN_POINT ( 'NONE',  ( -31.87600794503257617, 1525.042337199240364, 202.1059339849676917 ) ) ;
#35065=FACE_OUTER_BOUND ( 'NONE', #36151, .T. ) ;
#35066=CARTESIAN_POINT ( 'NONE',  ( -29.30029655192924665, 1525.907212628473644, 221.3719603026177367 ) ) ;
#35083=EDGE_CURVE ( 'NONE', #57779, #90117, #16399, .T. ) ;
#35097=CARTESIAN_POINT ( 'NONE',  ( -29.52630424919052388, 1525.661275128775515, 196.5237685151092819 ) ) ;
#35100=CARTESIAN_POINT ( 'NONE',  ( 31.41104781486818354, 1512.187213306747481, 202.3296363711535264 ) ) ;
#35106=CARTESIAN_POINT ( 'NONE',  ( 2.682480990172567026, 1524.330813522192102, 241.8675070349544001 ) ) ;
#35110=EDGE_CURVE ( 'NONE', #40565, #50666, #37535, .T. ) ;
#35113=DIRECTION ( 'NONE',  ( -0.000000000000000000, -1.000000000000000000, -0.000000000000000000 ) ) ;
#35115=CARTESIAN_POINT ( 'NONE',  ( 28.62766089293167227, 1526.344110814219221, 220.1997210292020952 ) ) ;
#35123=DIRECTION ( 'NONE',  ( 0.4978433412588624818, 0.000000000000000000, -0.8672669759446693938 ) ) ;
#35129=CARTESIAN_POINT ( 'NONE',  ( 30.31940284292418752, 1523.456872492435195, 222.4933038710543372 ) ) ;
#35133=CARTESIAN_POINT ( 'NONE',  ( 33.36586802512172767, 1511.187213306747708, 201.9069332299488622 ) ) ;
#35135=VECTOR ( 'NONE', #23045, 1000.000000000000000 ) ;
#35138=PLANE ( 'NONE',  #76903 ) ;
#35140=LINE ( 'NONE', #17195, #15961 ) ;
#35166=VERTEX_POINT ( 'NONE', #20351 ) ;
#35171=CARTESIAN_POINT ( 'NONE',  ( 0.000000000000000000, 1512.187213306747481, 209.1218459616979999 ) ) ;
#35175=EDGE_LOOP ( 'NONE', ( #45018, #24140, #53250, #20472, #73625 ) ) ;
#35177=CARTESIAN_POINT ( 'NONE',  ( -2.865544263339262265, 1525.651286436460623, 177.1364475444147502 ) ) ;
#35193=DIRECTION ( 'NONE',  ( -0.7414773880254650340, -0.000000000000000000, -0.6709778558543747495 ) ) ;
#35195=DIRECTION ( 'NONE',  ( 0.000000000000000000, -0.000000000000000000, 1.000000000000000000 ) ) ;
#35219=CARTESIAN_POINT ( 'NONE',  ( -16.48487881372712494, 1525.795403621571268, 181.7735847721916684 ) ) ;
#35221=CIRCLE ( 'NONE', #51360, 1.000000000000000888 ) ;
#35222=DIRECTION ( 'NONE',  ( 0.000000000000000000, 0.000000000000000000, -1.000000000000000000 ) ) ;
#35226=CARTESIAN_POINT ( 'NONE',  ( -1.191524307911311809, 1526.382868172863937, 179.0083900503167911 ) ) ;
#35264=ORIENTED_EDGE ( 'NONE', *, *, #4899, .T. ) ;
#35273=AXIS2_PLACEMENT_3D ( 'NONE', #105877, #72824, #63345 ) ;
#35274=CARTESIAN_POINT ( 'NONE',  ( -3.350338079455601026, 1523.604703353109699, 242.0808062845893289 ) ) ;
#35279=ORIENTED_EDGE ( 'NONE', *, *, #21508, .T. ) ;
#35283=FACE_OUTER_BOUND ( 'NONE', #4636, .T. ) ;
#35297=CIRCLE ( 'NONE', #13856, 0.9999999999999952260 ) ;
#35326=DIRECTION ( 'NONE',  ( 0.3090169943749382919, 0.000000000000000000, 0.9510565162951565288 ) ) ;
#35331=AXIS2_PLACEMENT_3D ( 'NONE', #94342, #77025, #76456 ) ;
#35337=ORIENTED_EDGE ( 'NONE', *, *, #74428, .T. ) ;
#35364=CARTESIAN_POINT ( 'NONE',  ( 28.81649562247350360, 1526.349689584397083, 198.1982788008647276 ) ) ;
#35366=CARTESIAN_POINT ( 'NONE',  ( -18.02257621027615997, 1526.382868172863937, 182.8951942368373977 ) ) ;
#35370=ORIENTED_EDGE ( 'NONE', *, *, #33532, .F. ) ;
#35381=AXIS2_PLACEMENT_3D ( 'NONE', #2667, #36793, #70985 ) ;
#35386=ADVANCED_FACE ( 'NONE', ( #103684 ), #394, .T. ) ;
#35391=CARTESIAN_POINT ( 'NONE',  ( 17.78793056501380931, 1523.919943579690425, 237.8334796938502791 ) ) ;
#35400=ORIENTED_EDGE ( 'NONE', *, *, #102331, .F. ) ;
#35403=AXIS2_PLACEMENT_3D ( 'NONE', #96552, #77134, #97649 ) ;
#35407=CIRCLE ( 'NONE', #55333, 1.000000000000002442 ) ;
#35437=CARTESIAN_POINT ( 'NONE',  ( 0.000000000000000000, 1511.187213306747708, 209.1218459616979999 ) ) ;
#35443=ORIENTED_EDGE ( 'NONE', *, *, #6434, .F. ) ;
#35444=ORIENTED_EDGE ( 'NONE', *, *, #25315, .T. ) ;
#35446=CARTESIAN_POINT ( 'NONE',  ( 21.35000886514773555, 1525.163527997504843, 183.8373093396160982 ) ) ;
#35448=CARTESIAN_POINT ( 'NONE',  ( 18.66420869458043796, 1526.382868172863937, 185.4599087859680537 ) ) ;
#35451=CARTESIAN_POINT ( 'NONE',  ( -1.393816646507350487, 1511.187213306747708, 243.1385343369520342 ) ) ;
#35492=AXIS2_PLACEMENT_3D ( 'NONE', #91047, #38443, #5955 ) ;
#35515=AXIS2_PLACEMENT_3D ( 'NONE', #22874, #73873, #97553 ) ;
#35521=DIRECTION ( 'NONE',  ( 0.000000000000000000, 0.000000000000000000, -1.000000000000000000 ) ) ;
#35532=CARTESIAN_POINT ( 'NONE',  ( 20.39146254758223265, 1526.073434386618828, 185.1130326267048645 ) ) ;
#35541=CARTESIAN_POINT ( 'NONE',  ( 19.53786426059019021, 1512.187213306747481, 181.5239794925693388 ) ) ;
#35545=ORIENTED_EDGE ( 'NONE', *, *, #45772, .F. ) ;
#35551=FACE_OUTER_BOUND ( 'NONE', #13015, .T. ) ;
#35554=DIRECTION ( 'NONE',  ( 0.000000000000000000, 0.000000000000000000, 1.000000000000000000 ) ) ;
#35567=AXIS2_PLACEMENT_3D ( 'NONE', #53292, #79048, #80120 ) ;
#35574=CARTESIAN_POINT ( 'NONE',  ( -32.21733215213330936, 1523.844782250843309, 201.4553020982646387 ) ) ;
#35605=ORIENTED_EDGE ( 'NONE', *, *, #93254, .T. ) ;
#35607=CARTESIAN_POINT ( 'NONE',  ( 30.31940284292420174, 1512.187213306747481, 222.4933038710543087 ) ) ;
#35623=AXIS2_PLACEMENT_3D ( 'NONE', #95335, #29234, #61760 ) ;
#35637=ORIENTED_EDGE ( 'NONE', *, *, #42012, .F. ) ;
#35639=CARTESIAN_POINT ( 'NONE',  ( -20.21023357682352994, 1526.107880201381477, 184.5539505003309841 ) ) ;
#35641=AXIS2_PLACEMENT_3D ( 'NONE', #8238, #107542, #41857 ) ;
#35644=( BOUNDED_SURFACE ( )  B_SPLINE_SURFACE ( 3, 2, ( 
 ( #86340, #2926, #71236 ),
 ( #17451, #94181, #95304 ),
 ( #85789, #11310, #9625 ),
 ( #44927, #36496, #96410 ) ),
 .UNSPECIFIED., .F., .F., .F. ) 
 B_SPLINE_SURFACE_WITH_KNOTS ( ( 4, 4 ),
 ( 3, 3 ),
 ( 0.000000000000000000, 0.0002960034161023851105 ),
 ( 0.000000000000000000, 1.000000000000000000 ),
 .UNSPECIFIED. ) 
 GEOMETRIC_REPRESENTATION_ITEM ( )  RATIONAL_B_SPLINE_SURFACE ( (
 ( 1.000000000000000000, 0.8070209408750127489, 1.000000000000000000),
 ( 1.000000000000000000, 0.8071723757218264295, 1.000000000000000000),
 ( 1.000000000000000000, 0.8072480346917805250, 1.000000000000000000),
 ( 1.000000000000000000, 0.8072480644198094524, 1.000000000000000000) ) ) 
 REPRESENTATION_ITEM ( '' )  SURFACE ( )  );
#35649=CARTESIAN_POINT ( 'NONE',  ( -30.04019103850641770, 1524.756004293092019, 195.9352227457331139 ) ) ;
#35668=CARTESIAN_POINT ( 'NONE',  ( 29.13898522073297315, 1526.069472839380978, 221.1027213634262409 ) ) ;
#35693=EDGE_CURVE ( 'NONE', #13874, #237, #8225, .T. ) ;
#35701=ORIENTED_EDGE ( 'NONE', *, *, #65823, .F. ) ;
#35708=ADVANCED_FACE ( 'NONE', ( #75474 ), #58660, .T. ) ;
#35709=DIRECTION ( 'NONE',  ( -0.2054769195713296581, 0.000000000000000000, -0.9786619618251632957 ) ) ;
#35713=FACE_OUTER_BOUND ( 'NONE', #82849, .T. ) ;
#35729=TOROIDAL_SURFACE ( 'NONE', #8854, 1.000000000000000000, 1.000000000000000000 ) ;
#35754=CARTESIAN_POINT ( 'NONE',  ( 2.372478608332516892, 1522.382868172863937, 174.8996806668726549 ) ) ;
#35783=CARTESIAN_POINT ( 'NONE',  ( 3.237130272123891928, 1524.843178112495480, 241.7217292875349415 ) ) ;
#35786=CARTESIAN_POINT ( 'NONE',  ( 21.41029105011577727, 1526.329757971583831, 234.0206363886036343 ) ) ;
#35794=CARTESIAN_POINT ( 'NONE',  ( -28.70874162694016007, 1526.306647125541986, 197.9001931917368893 ) ) ;
#35802=CARTESIAN_POINT ( 'NONE',  ( -30.51231035492526900, 1526.382868172863937, 200.0858385050243555 ) ) ;
#35808=AXIS2_PLACEMENT_3D ( 'NONE', #32938, #59826, #92849 ) ;
#35811=PLANE ( 'NONE',  #28980 ) ;
#35823=CARTESIAN_POINT ( 'NONE',  ( -32.21733187660822040, 1523.844789899202397, 216.7883882218984013 ) ) ;
#35824=ORIENTED_EDGE ( 'NONE', *, *, #47629, .F. ) ;
#35833=VECTOR ( 'NONE', #68473, 1000.000000000000000 ) ;
#35839=CARTESIAN_POINT ( 'NONE',  ( -32.86802468386297704, 1523.382868172864164, 201.0396662540046577 ) ) ;
#35843=VERTEX_POINT ( 'NONE', #9767 ) ;
#35866=EDGE_LOOP ( 'NONE', ( #70268, #12351, #34776, #47598 ) ) ;
#35908=CARTESIAN_POINT ( 'NONE',  ( 30.44527832718689808, 1526.211523310372513, 201.0917162105438933 ) ) ;
#35909=CYLINDRICAL_SURFACE ( 'NONE', #9107, 1.000000000000000888 ) ;
#35929=CARTESIAN_POINT ( 'NONE',  ( -20.71343476518021731, 1522.906561336852974, 179.9059455038230908 ) ) ;
#35942=CARTESIAN_POINT ( 'NONE',  ( 31.12456774391177206, 1525.960063244516959, 217.0912716842394730 ) ) ;
#35949=CARTESIAN_POINT ( 'NONE',  ( -33.28034951413919629, 1522.382868172863937, 217.4407153818824554 ) ) ;
#35962=VERTEX_POINT ( 'NONE', #88703 ) ;
#35966=DIRECTION ( 'NONE',  ( -0.3090169943749582204, 0.000000000000000000, -0.9510565162951499785 ) ) ;
#35968=CARTESIAN_POINT ( 'NONE',  ( -30.16747994869158944, 1524.964230758882877, 196.5181873855272272 ) ) ;
#35983=EDGE_CURVE ( 'NONE', #29937, #50057, #104030, .T. ) ;
#36007=VERTEX_POINT ( 'NONE', #76294 ) ;
#36009=CARTESIAN_POINT ( 'NONE',  ( 20.70484064406382529, 1525.907212628473644, 185.0411015109853565 ) ) ;
#36011=CARTESIAN_POINT ( 'NONE',  ( 19.29374783221134138, 1526.349684470114653, 185.0912796807455152 ) ) ;
#36016=( BOUNDED_CURVE ( )  B_SPLINE_CURVE ( 3, ( #27950, #36896, #44210, #35802 ),
 .UNSPECIFIED., .F., .F. ) 
 B_SPLINE_CURVE_WITH_KNOTS ( ( 4, 4 ),
 ( 3.141592653589793116, 4.712388980384689674 ),
 .UNSPECIFIED. ) 
 CURVE ( )  GEOMETRIC_REPRESENTATION_ITEM ( )  RATIONAL_B_SPLINE_CURVE ( ( 1.000000000000000000, 0.8047378541243649375, 0.8047378541243649375, 1.000000000000000000 ) ) 
 REPRESENTATION_ITEM ( '' )  );
#36029=CYLINDRICAL_SURFACE ( 'NONE', #97720, 1.999999999999998668 ) ;
#36033=CYLINDRICAL_SURFACE ( 'NONE', #16118, 0.9999999999999873435 ) ;
#36072=CARTESIAN_POINT ( 'NONE',  ( -16.97881484272415875, 1525.055402519470135, 236.9933241842670100 ) ) ;
#36074=CARTESIAN_POINT ( 'NONE',  ( 30.61611611310372894, 1526.069472839377568, 216.5565799337455530 ) ) ;
#36075=CARTESIAN_POINT ( 'NONE',  ( 19.01706420256806496, 1526.382868172863937, 232.8536233449245287 ) ) ;
#36091=AXIS2_PLACEMENT_3D ( 'NONE', #15521, #30130, #22815 ) ;
#36106=CARTESIAN_POINT ( 'NONE',  ( -30.51126001304075430, 1526.382868172863937, 198.3878992055731487 ) ) ;
#36138=DIRECTION ( 'NONE',  ( 0.000000000000000000, 1.000000000000000000, 0.000000000000000000 ) ) ;
#36142=CARTESIAN_POINT ( 'NONE',  ( -31.56778878607243044, 1525.408337840050308, 202.0372949643508491 ) ) ;
#36151=EDGE_LOOP ( 'NONE', ( #73537, #31971, #38492, #42862 ) ) ;
#36155=ORIENTED_EDGE ( 'NONE', *, *, #49415, .F. ) ;
#36172=VERTEX_POINT ( 'NONE', #66816 ) ;
#36185=ORIENTED_EDGE ( 'NONE', *, *, #71695, .T. ) ;
#36204=DIRECTION ( 'NONE',  ( -0.01594118961724027769, -0.9969860201949399814, -0.07592597717146752634 ) ) ;
#36211=CARTESIAN_POINT ( 'NONE',  ( -21.54890432409634116, 1524.816846803860926, 234.5807495618499559 ) ) ;
#36217=CARTESIAN_POINT ( 'NONE',  ( -34.18677586421173231, 1522.382868172863937, 219.7932833225216882 ) ) ;
#36242=CARTESIAN_POINT ( 'NONE',  ( 29.40443212115383531, 1511.187213306747708, 196.1539082851714966 ) ) ;
#36280=CARTESIAN_POINT ( 'NONE',  ( -49.24962907673571522, 1526.382868172863937, 10.34030387146701813 ) ) ;
#36281=FACE_OUTER_BOUND ( 'NONE', #18497, .T. ) ;
#36295=DIRECTION ( 'NONE',  ( -0.6709778558543747495, 0.000000000000000000, 0.7414773880254650340 ) ) ;
#36325=DIRECTION ( 'NONE',  ( -0.3090169943749516146, 0.000000000000000000, -0.9510565162951523099 ) ) ;
#36326=CARTESIAN_POINT ( 'NONE',  ( 21.61975802670987790, 1524.130440953581001, 234.4879735737363831 ) ) ;
#36336=EDGE_CURVE ( 'NONE', #105303, #49707, #20023, .T. ) ;
#36363=CARTESIAN_POINT ( 'NONE',  ( -32.18357971100785875, 1524.059663615500540, 216.7473357175133231 ) ) ;
#36364=VERTEX_POINT ( 'NONE', #5085 ) ;
#36371=EDGE_CURVE ( 'NONE', #77376, #68723, #101020, .T. ) ;
#36386=ORIENTED_EDGE ( 'NONE', *, *, #41240, .T. ) ;
#36393=CARTESIAN_POINT ( 'NONE',  ( 32.48417584039749784, 1524.659802833172535, 201.1732701908057379 ) ) ;
#36398=CARTESIAN_POINT ( 'NONE',  ( -2.469101154908970308, 1524.816548299036640, 175.8588282813664705 ) ) ;
#36416=ORIENTED_EDGE ( 'NONE', *, *, #96154, .T. ) ;
#36420=ORIENTED_EDGE ( 'NONE', *, *, #105597, .T. ) ;
#36449=DIRECTION ( 'NONE',  ( -0.000000000000000000, -1.000000000000000000, -0.000000000000000000 ) ) ;
#36461=AXIS2_PLACEMENT_3D ( 'NONE', #68616, #1400, #94903 ) ;
#36462=CARTESIAN_POINT ( 'NONE',  ( 21.83550407203906119, 1523.678648413191468, 183.2743720722706655 ) ) ;
#36466=CARTESIAN_POINT ( 'NONE',  ( -16.68062049856758122, 1526.382868172863937, 181.4122394607865942 ) ) ;
#36467=ADVANCED_FACE ( 'NONE', ( #65012 ), #15122, .T. ) ;
#36471=ORIENTED_EDGE ( 'NONE', *, *, #105916, .F. ) ;
#36480=DIRECTION ( 'NONE',  ( 0.000000000000000000, 1.000000000000000000, 0.000000000000000000 ) ) ;
#36483=ADVANCED_FACE ( 'NONE', ( #5654 ), #83438, .T. ) ;
#36496=CARTESIAN_POINT ( 'NONE',  ( 32.23393008313279040, 1523.382868172864164, 216.8400319010852400 ) ) ;
#36497=B_SPLINE_CURVE_WITH_KNOTS ( 'NONE', 3,
 ( #57460, #55250, #4813, #108389, #80983, #91587, #23262, #21048, #89382, #38959 ),
 .UNSPECIFIED., .F., .F.,
 ( 4, 2, 2, 2, 4 ),
 ( 3.469446951953613804E-18, 0.0007403986298595397093, 0.001480797259719075949, 0.002221195889578612189, 0.002961594519438148429 ),
 .UNSPECIFIED. ) ;
#36500=DIRECTION ( 'NONE',  ( 2.775557561562888827E-14, 0.000000000000000000, 1.000000000000000000 ) ) ;
#36511=FACE_OUTER_BOUND ( 'NONE', #104395, .T. ) ;
#36516=CARTESIAN_POINT ( 'NONE',  ( 20.53760542139786693, 1525.821544997590308, 233.5223198772804949 ) ) ;
#36534=DIRECTION ( 'NONE',  ( 0.000000000000000000, 1.000000000000000000, -0.000000000000000000 ) ) ;
#36536=CARTESIAN_POINT ( 'NONE',  ( -0.4151546846821903003, 1512.187213306747481, 242.9330574173806951 ) ) ;
#36547=EDGE_LOOP ( 'NONE', ( #106812, #9182, #38429, #105124 ) ) ;
#36550=CARTESIAN_POINT ( 'NONE',  ( 21.80586012576933541, 1523.954924407801855, 183.3405100316582832 ) ) ;
#36557=CARTESIAN_POINT ( 'NONE',  ( -33.93019615848960768, 1522.382868172863937, 197.6607374646001176 ) ) ;
#36569=VERTEX_POINT ( 'NONE', #29069 ) ;
#36583=ORIENTED_EDGE ( 'NONE', *, *, #48129, .T. ) ;
#36585=ORIENTED_EDGE ( 'NONE', *, *, #97878, .F. ) ;
#36614=CARTESIAN_POINT ( 'NONE',  ( 30.68434753607487764, 1526.000688113786737, 216.8500914425656845 ) ) ;
#36625=ORIENTED_EDGE ( 'NONE', *, *, #105132, .F. ) ;
#36633=( BOUNDED_SURFACE ( )  B_SPLINE_SURFACE ( 3, 2, ( 
 ( #48594, #83276, #6574 ),
 ( #40722, #74894, #103935 ),
 ( #53563, #25550, #2057 ),
 ( #949, #59742, #95537 ) ),
 .UNSPECIFIED., .F., .F., .T. ) 
 B_SPLINE_SURFACE_WITH_KNOTS ( ( 4, 4 ),
 ( 3, 3 ),
 ( 0.000000000000000000, 0.0002960034161023848936 ),
 ( 0.000000000000000000, 1.000000000000000000 ),
 .UNSPECIFIED. ) 
 GEOMETRIC_REPRESENTATION_ITEM ( )  RATIONAL_B_SPLINE_SURFACE ( (
 ( 1.000000000000000000, 0.8070209408750060875, 1.000000000000000000),
 ( 1.000000000000000000, 0.8071723757218383088, 1.000000000000000000),
 ( 1.000000000000000000, 0.8072480346917747518, 1.000000000000000000),
 ( 1.000000000000000000, 0.8072480644198177790, 1.000000000000000000) ) ) 
 REPRESENTATION_ITEM ( '' )  SURFACE ( )  );
#36643=ORIENTED_EDGE ( 'NONE', *, *, #23070, .T. ) ;
#36645=DIRECTION ( 'NONE',  ( 0.000000000000000000, 0.000000000000000000, -1.000000000000000000 ) ) ;
#36649=CARTESIAN_POINT ( 'NONE',  ( -29.99620953741503371, 1526.382868172863937, 198.4974435154502999 ) ) ;
#36650=EDGE_CURVE ( 'NONE', #94190, #71731, #76022, .T. ) ;
#36680=ORIENTED_EDGE ( 'NONE', *, *, #38125, .T. ) ;
#36684=CARTESIAN_POINT ( 'NONE',  ( 0.000000000000000000, 1524.090675761330203, 232.8211094035767985 ) ) ;
#36688=CARTESIAN_POINT ( 'NONE',  ( -32.36539586358053810, 1523.843263703803586, 202.1341903664009294 ) ) ;
#36696=ORIENTED_EDGE ( 'NONE', *, *, #30850, .T. ) ;
#36705=EDGE_LOOP ( 'NONE', ( #86180, #82828, #53326, #43853, #97973 ) ) ;
#36708=AXIS2_PLACEMENT_3D ( 'NONE', #35133, #69875, #104549 ) ;
#36720=DIRECTION ( 'NONE',  ( 0.000000000000000000, 0.000000000000000000, -1.000000000000000000 ) ) ;
#36746=CARTESIAN_POINT ( 'NONE',  ( -20.92767404034479028, 1512.187213306747481, 235.3888156262297571 ) ) ;
#36754=VERTEX_POINT ( 'NONE', #78517 ) ;
#36760=CARTESIAN_POINT ( 'NONE',  ( -33.05665451062068172, 1523.390106123591067, 200.9313857523611375 ) ) ;
#36761=CARTESIAN_POINT ( 'NONE',  ( -21.32681782946734828, 1525.211473355384896, 234.3841091294584373 ) ) ;
#36764=CARTESIAN_POINT ( 'NONE',  ( -28.27139721233033143, 1526.382868172863937, 219.5606225550389752 ) ) ;
#36771=CARTESIAN_POINT ( 'NONE',  ( -30.25425994616995240, 1522.382868172863937, 218.9520509131593258 ) ) ;
#36778=CARTESIAN_POINT ( 'NONE',  ( -2.038646110889595242, 1525.960063244516959, 241.1857569150894562 ) ) ;
#36788=EDGE_CURVE ( 'NONE', #32282, #46630, #70719, .T. ) ;
#36793=DIRECTION ( 'NONE',  ( 0.8090169943749551118, 0.000000000000000000, 0.5877852522924624790 ) ) ;
#36794=EDGE_LOOP ( 'NONE', ( #22379, #14530, #23470, #62530 ) ) ;
#36795=ORIENTED_EDGE ( 'NONE', *, *, #96189, .T. ) ;
#36811=CARTESIAN_POINT ( 'NONE',  ( 2.857351367441036238, 1525.661276915132476, 241.0960470690656052 ) ) ;
#36836=ORIENTED_EDGE ( 'NONE', *, *, #92004, .T. ) ;
#36848=ORIENTED_EDGE ( 'NONE', *, *, #48798, .T. ) ;
#36853=DIRECTION ( 'NONE',  ( 0.000000000000000000, 0.000000000000000000, -1.000000000000000000 ) ) ;
#36856=AXIS2_PLACEMENT_3D ( 'NONE', #1198, #9568, #26937 ) ;
#36871=DIRECTION ( 'NONE',  ( 0.000000000000000000, 1.000000000000000000, 0.000000000000000000 ) ) ;
#36880=CARTESIAN_POINT ( 'NONE',  ( 22.03465957474240255, 1522.644714754858114, 235.4136513321555810 ) ) ;
#36896=CARTESIAN_POINT ( 'NONE',  ( -34.18677586421193837, 1524.726013923371283, 198.4504086008750505 ) ) ;
#36910=VERTEX_POINT ( 'NONE', #46583 ) ;
#36920=CARTESIAN_POINT ( 'NONE',  ( 33.28034951413924603, 1501.977400791986611, 200.8029765415137433 ) ) ;
#36931=EDGE_LOOP ( 'NONE', ( #98561, #102843, #59595, #96669 ) ) ;
#36938=CARTESIAN_POINT ( 'NONE',  ( 31.54873523816509362, 1525.317349363550193, 201.5741525441649742 ) ) ;
#36942=DIRECTION ( 'NONE',  ( -0.6709778558543776361, 0.000000000000000000, -0.7414773880254624805 ) ) ;
#36948=AXIS2_PLACEMENT_3D ( 'NONE', #74013, #14637, #56660 ) ;
#36955=FACE_OUTER_BOUND ( 'NONE', #20303, .T. ) ;
#36968=LINE ( 'NONE', #12311, #30358 ) ;
#36969=FACE_OUTER_BOUND ( 'NONE', #12314, .T. ) ;
#36975=ORIENTED_EDGE ( 'NONE', *, *, #100788, .T. ) ;
#36983=ADVANCED_FACE ( 'NONE', ( #75635 ), #58242, .F. ) ;
#36991=ORIENTED_EDGE ( 'NONE', *, *, #13717, .F. ) ;
#36996=EDGE_CURVE ( 'NONE', #47062, #98891, #45691, .T. ) ;
#37003=CARTESIAN_POINT ( 'NONE',  ( 0.000000000000000000, 1523.409940573003951, 209.1218459616979999 ) ) ;
#37013=CIRCLE ( 'NONE', #94229, 2.000000000000001776 ) ;
#37015=CARTESIAN_POINT ( 'NONE',  ( -17.43739734485818005, 1526.178928173327449, 180.7274168163475281 ) ) ;
#37028=DIRECTION ( 'NONE',  ( 0.000000000000000000, -1.000000000000000000, -0.000000000000000000 ) ) ;
#37040=DIRECTION ( 'NONE',  ( 0.5877852522924831291, 0.000000000000000000, 0.8090169943749401238 ) ) ;
#37042=CARTESIAN_POINT ( 'NONE',  ( 17.83486663330506872, 1523.678648413191695, 237.8759530894958800 ) ) ;
#37054=CARTESIAN_POINT ( 'NONE',  ( 31.76119286153732091, 1522.906363951597314, 196.2959455099801573 ) ) ;
#37056=EDGE_CURVE ( 'NONE', #2813, #27462, #22356, .T. ) ;
#37061=CARTESIAN_POINT ( 'NONE',  ( -29.86461515634930564, 1525.960063244516959, 197.2746849027939504 ) ) ;
#37064=CARTESIAN_POINT ( 'NONE',  ( 19.38211899476526767, 1526.344110814219221, 232.9251177427934181 ) ) ;
#37065=DIRECTION ( 'NONE',  ( 0.000000000000000000, -1.000000000000000000, 0.000000000000000000 ) ) ;
#37074=DIRECTION ( 'NONE',  ( -1.000000000000000000, -0.000000000000000000, -0.000000000000000000 ) ) ;
#37095=TOROIDAL_SURFACE ( 'NONE', #46075, 2.000000000000000000, 1.000000000000000000 ) ;
#37124=CARTESIAN_POINT ( 'NONE',  ( 2.309262712061971090, 1512.187213306747481, 217.7723287588028143 ) ) ;
#37129=DIRECTION ( 'NONE',  ( 0.000000000000000000, 0.000000000000000000, 1.000000000000000000 ) ) ;
#37135=B_SPLINE_CURVE_WITH_KNOTS ( 'NONE', 3,
 ( #73504, #107639, #66763, #31470, #50502, #5740, #100336, #108737, #32588, #82442, #83522, #75698 ),
 .UNSPECIFIED., .F., .F.,
 ( 4, 2, 2, 2, 2, 4 ),
 ( 0.000000000000000000, 0.0007194225121792582585, 0.001079133768269195789, 0.001438845024359133428, 0.002158267536539008706, 0.002877690048718883550 ),
 .UNSPECIFIED. ) ;
#37148=CARTESIAN_POINT ( 'NONE',  ( 21.84020450222056908, 1501.977400791986611, 234.9798068779740277 ) ) ;
#37162=CARTESIAN_POINT ( 'NONE',  ( -2.404972330437235684, 1525.211473355384896, 242.0950351792775450 ) ) ;
#37167=CARTESIAN_POINT ( 'NONE',  ( 29.53442096303756159, 1525.651285554130254, 221.7311742728463457 ) ) ;
#37174=CARTESIAN_POINT ( 'NONE',  ( -31.33756689035267229, 1523.580203803270933, 196.3415365178086631 ) ) ;
#37193=DIRECTION ( 'NONE',  ( 0.000000000000000000, -1.000000000000000000, 0.000000000000000000 ) ) ;
#37201=EDGE_CURVE ( 'NONE', #50084, #36569, #60159, .T. ) ;
#37205=VECTOR ( 'NONE', #95737, 1000.000000000000000 ) ;
#37206=CARTESIAN_POINT ( 'NONE',  ( -32.41382812665801794, 1525.581535527370306, 197.9832485531580630 ) ) ;
#37235=VERTEX_POINT ( 'NONE', #77695 ) ;
#37236=ORIENTED_EDGE ( 'NONE', *, *, #101696, .F. ) ;
#37243=CARTESIAN_POINT ( 'NONE',  ( -32.21030510514562195, 1524.412455883367329, 202.1448083870403138 ) ) ;
#37244=EDGE_CURVE ( 'NONE', #40573, #48513, #76106, .T. ) ;
#37256=AXIS2_PLACEMENT_3D ( 'NONE', #6455, #14286, #32206 ) ;
#37257=ORIENTED_EDGE ( 'NONE', *, *, #105628, .T. ) ;
#37259=CARTESIAN_POINT ( 'NONE',  ( 1.393816646507355372, 1511.187213306747708, 243.1385343369520342 ) ) ;
#37261=AXIS2_PLACEMENT_3D ( 'NONE', #59259, #18317, #16643 ) ;
#37265=EDGE_CURVE ( 'NONE', #43261, #40565, #70371, .T. ) ;
#37269=VECTOR ( 'NONE', #89068, 1000.000000000000000 ) ;
#37270=AXIS2_PLACEMENT_3D ( 'NONE', #35171, #67694, #25094 ) ;
#37273=CARTESIAN_POINT ( 'NONE',  ( -29.61076270571678748, 1526.107880201381477, 220.7510230871936017 ) ) ;
#37276=CARTESIAN_POINT ( 'NONE',  ( 2.143765237719135186, 1525.848196786131211, 176.8604030897658674 ) ) ;
#37277=ORIENTED_EDGE ( 'NONE', *, *, #47370, .T. ) ;
#37278=EDGE_CURVE ( 'NONE', #94190, #91380, #67169, .T. ) ;
#37288=DIRECTION ( 'NONE',  ( 0.000000000000000000, 0.000000000000000000, 1.000000000000000000 ) ) ;
#37297=ORIENTED_EDGE ( 'NONE', *, *, #14328, .T. ) ;
#37302=CARTESIAN_POINT ( 'NONE',  ( -29.37019419317373448, 1526.382868172864164, 217.2592043484932844 ) ) ;
#37311=CARTESIAN_POINT ( 'NONE',  ( -18.66420869458074350, 1526.382868172863937, 185.4599087859683095 ) ) ;
#37337=DIRECTION ( 'NONE',  ( -0.000000000000000000, -1.000000000000000000, -0.000000000000000000 ) ) ;
#37338=CIRCLE ( 'NONE', #42690, 1.000000000000000888 ) ;
#37363=CARTESIAN_POINT ( 'NONE',  ( -18.66420869458074350, 1526.382868172863937, 185.4599087859683095 ) ) ;
#37365=CARTESIAN_POINT ( 'NONE',  ( 3.350338079455601026, 1523.604703353109699, 242.0808062845893289 ) ) ;
#37384=EDGE_LOOP ( 'NONE', ( #29042, #26434, #62567, #91918 ) ) ;
#37421=ADVANCED_FACE ( 'NONE', ( #42996 ), #29484, .T. ) ;
#37439=CARTESIAN_POINT ( 'NONE',  ( 3.355801963978102709, 1523.843263703804496, 242.0624709300151380 ) ) ;
#37440=ORIENTED_EDGE ( 'NONE', *, *, #44818, .T. ) ;
#37456=CARTESIAN_POINT ( 'NONE',  ( -3.141370515551505260, 1525.159196711359755, 176.7077266983532411 ) ) ;
#37458=CARTESIAN_POINT ( 'NONE',  ( -1.191524307911310698, 1526.382868172864164, 239.2353018730791518 ) ) ;
#37466=DIRECTION ( 'NONE',  ( 0.000000000000000000, 0.000000000000000000, 1.000000000000000000 ) ) ;
#37473=CARTESIAN_POINT ( 'NONE',  ( -31.52384642519460911, 1525.730671215514576, 217.0357139665296700 ) ) ;
#37474=VERTEX_POINT ( 'NONE', #20519 ) ;
#37479=CARTESIAN_POINT ( 'NONE',  ( -29.30029655192934257, 1525.907212628473644, 221.3719603026177367 ) ) ;
#37499=CARTESIAN_POINT ( 'NONE',  ( 32.85805783624305576, 1523.678648413191695, 201.0453875934054224 ) ) ;
#37504=CIRCLE ( 'NONE', #53691, 1.000000000000001554 ) ;
#37525=ORIENTED_EDGE ( 'NONE', *, *, #82945, .F. ) ;
#37535=B_SPLINE_CURVE_WITH_KNOTS ( 'NONE', 3,
 ( #107122, #37174, #89769, #13040 ),
 .UNSPECIFIED., .F., .F.,
 ( 4, 4 ),
 ( 0.000000000000000000, 0.0002960034161023847310 ),
 .UNSPECIFIED. ) ;
#37549=AXIS2_PLACEMENT_3D ( 'NONE', #14652, #108161, #74028 ) ;
#37560=CARTESIAN_POINT ( 'NONE',  ( -21.84020450222076448, 1512.187213306747481, 183.2638850454220858 ) ) ;
#37571=CARTESIAN_POINT ( 'NONE',  ( 21.84020450222037724, 1523.382868172864164, 183.2638850454218016 ) ) ;
#37576=ORIENTED_EDGE ( 'NONE', *, *, #62503, .T. ) ;
#37587=CARTESIAN_POINT ( 'NONE',  ( -20.60985939166187464, 1525.581535527370988, 236.5072125268898731 ) ) ;
#37588=VECTOR ( 'NONE', #58971, 1000.000000000000227 ) ;
#37615=CARTESIAN_POINT ( 'NONE',  ( -29.70307915522685960, 1525.408327360766862, 196.2982788325003867 ) ) ;
#37626=CARTESIAN_POINT ( 'NONE',  ( 2.372478608332516892, 1512.187213306747481, 243.3440112565233449 ) ) ;
#37629=CARTESIAN_POINT ( 'NONE',  ( -22.03465957474533354, 1522.382868172863937, 235.4136513321633117 ) ) ;
#37654=ORIENTED_EDGE ( 'NONE', *, *, #56365, .T. ) ;
#37655=CARTESIAN_POINT ( 'NONE',  ( 20.21024070146847151, 1526.107876515966609, 184.5539461604345775 ) ) ;
#37658=LINE ( 'NONE', #55582, #14675 ) ;
#37672=ORIENTED_EDGE ( 'NONE', *, *, #21926, .F. ) ;
#37696=CARTESIAN_POINT ( 'NONE',  ( 30.51231035492518728, 1524.382868172863937, 200.0858385050239008 ) ) ;
#37716=AXIS2_PLACEMENT_3D ( 'NONE', #72770, #106898, #47564 ) ;
#37732=ADVANCED_FACE ( 'NONE', ( #58019 ), #23870, .F. ) ;
#37734=EDGE_CURVE ( 'NONE', #81438, #82322, #33174, .T. ) ;
#37738=EDGE_CURVE ( 'NONE', #30213, #95653, #86814, .T. ) ;
#37744=ADVANCED_FACE ( 'NONE', ( #35551 ), #77024, .T. ) ;
#37747=CIRCLE ( 'NONE', #23416, 1.000000000000000444 ) ;
#37764=EDGE_CURVE ( 'NONE', #51540, #63441, #78667, .T. ) ;
#37765=CIRCLE ( 'NONE', #10911, 0.9999999999999873435 ) ;
#37789=ORIENTED_EDGE ( 'NONE', *, *, #4853, .F. ) ;
#37805=CARTESIAN_POINT ( 'NONE',  ( -16.69297358003532139, 1526.382868172864164, 183.6963177704346606 ) ) ;
#37818=EDGE_CURVE ( 'NONE', #100587, #52269, #110076, .T. ) ;
#37822=CARTESIAN_POINT ( 'NONE',  ( 20.20959865099491992, 1512.187213306747481, 236.2316688286738611 ) ) ;
#37837=CARTESIAN_POINT ( 'NONE',  ( -2.640434834157761479, 1526.748660780343471, 241.3121066639439221 ) ) ;
#37862=ORIENTED_EDGE ( 'NONE', *, *, #43449, .F. ) ;
#37873=ADVANCED_FACE ( 'NONE', ( #90352 ), #47455, .F. ) ;
#37874=CARTESIAN_POINT ( 'NONE',  ( 17.84338787552341543, 1523.481610118011986, 180.3600277898069919 ) ) ;
#37877=CARTESIAN_POINT ( 'NONE',  ( -32.66476241579304940, 1526.382868172863937, 219.1158660759124643 ) ) ;
#37879=CARTESIAN_POINT ( 'NONE',  ( 2.038847259693655545, 1522.861859112239017, 244.9330574173661716 ) ) ;
#37904=EDGE_LOOP ( 'NONE', ( #33798, #16988, #36991, #93243, #104734 ) ) ;
#37905=EDGE_LOOP ( 'NONE', ( #21914, #39737, #34788, #36643, #50615 ) ) ;
#37922=CARTESIAN_POINT ( 'NONE',  ( 32.77044109517470361, 1525.581535527371443, 199.0807904155084600 ) ) ;
#37932=CIRCLE ( 'NONE', #109465, 1.000000000000002442 ) ;
#37951=( BOUNDED_SURFACE ( )  B_SPLINE_SURFACE ( 3, 2, ( 
 ( #110345, #40938, #102483 ),
 ( #8424, #23579, #24654 ),
 ( #101929, #34191, #77313 ),
 ( #42595, #16802, #49905 ),
 ( #85137, #101363, #58855 ),
 ( #15164, #25772, #93532 ) ),
 .UNSPECIFIED., .F., .F., .F. ) 
 B_SPLINE_SURFACE_WITH_KNOTS ( ( 4, 2, 4 ),
 ( 3, 3 ),
 ( 2.723515857283587138E-16, 0.001312027981647352279, 0.002624055963294432206 ),
 ( 0.000000000000000000, 1.000000000000000000 ),
 .UNSPECIFIED. ) 
 GEOMETRIC_REPRESENTATION_ITEM ( )  RATIONAL_B_SPLINE_SURFACE ( (
 ( 1.000000000000000000, 0.9376006582765955555, 1.000000000000000000),
 ( 1.000000000000000000, 0.9569320108030413552, 1.000000000000000000),
 ( 1.000000000000000000, 0.9725743441608736273, 1.000000000000000000),
 ( 1.000000000000000000, 0.9942095667145922633, 1.000000000000000000),
 ( 1.000000000000000000, 1.000043666449937030, 1.000000000000000000),
 ( 1.000000000000000000, 1.000000000000000000, 1.000000000000000000) ) ) 
 REPRESENTATION_ITEM ( '' )  SURFACE ( )  );
#37975=VERTEX_POINT ( 'NONE', #1854 ) ;
#37976=CARTESIAN_POINT ( 'NONE',  ( -2.470168521978398868, 1512.187213306747481, 242.8787258963054683 ) ) ;
#37977=EDGE_CURVE ( 'NONE', #67344, #77058, #107440, .T. ) ;
#37989=CARTESIAN_POINT ( 'NONE',  ( 3.350338079455627671, 1523.604703353109926, 242.0808062845893289 ) ) ;
#38000=ADVANCED_FACE ( 'NONE', ( #97933 ), #20290, .T. ) ;
#38007=CARTESIAN_POINT ( 'NONE',  ( -3.355892881418364837, 1523.847233649538339, 176.1815261159892145 ) ) ;
#38014=FACE_OUTER_BOUND ( 'NONE', #830, .T. ) ;
#38022=ORIENTED_EDGE ( 'NONE', *, *, #52153, .F. ) ;
#38053=CARTESIAN_POINT ( 'NONE',  ( 31.30542570072814712, 1525.651285554129345, 201.9631097759967133 ) ) ;
#38056=CARTESIAN_POINT ( 'NONE',  ( 3.355893228018326457, 1523.847248782568613, 176.1815272790888685 ) ) ;
#38078=VERTEX_POINT ( 'NONE', #40795 ) ;
#38079=ORIENTED_EDGE ( 'NONE', *, *, #19891, .F. ) ;
#38093=EDGE_LOOP ( 'NONE', ( #94525, #98545, #34522, #24485, #62472, #52694, #28660, #13744 ) ) ;
#38098=CARTESIAN_POINT ( 'NONE',  ( 2.580915939757335575, 1524.130440953581001, 175.8924427158433446 ) ) ;
#38106=DIRECTION ( 'NONE',  ( 0.000000000000000000, 1.000000000000000000, 0.000000000000000000 ) ) ;
#38115=CARTESIAN_POINT ( 'NONE',  ( 21.38516915557986309, 1501.977400791986611, 237.8497028174237471 ) ) ;
#38122=DIRECTION ( 'NONE',  ( 0.000000000000000000, 0.000000000000000000, 1.000000000000000000 ) ) ;
#38125=EDGE_CURVE ( 'NONE', #102452, #89999, #63914, .T. ) ;
#38127=FACE_OUTER_BOUND ( 'NONE', #55597, .T. ) ;
#38132=CARTESIAN_POINT ( 'NONE',  ( -21.19880661588965509, 1526.382868172863937, 233.5487980989313712 ) ) ;
#38146=B_SPLINE_CURVE_WITH_KNOTS ( 'NONE', 3,
 ( #107205, #90949, #14235, #48424 ),
 .UNSPECIFIED., .F., .F.,
 ( 4, 4 ),
 ( 0.000000000000000000, 0.0002220129587134778832 ),
 .UNSPECIFIED. ) ;
#38147=CARTESIAN_POINT ( 'NONE',  ( 19.33418355719898329, 1523.342713519622976, 179.0109766843270052 ) ) ;
#38168=FACE_OUTER_BOUND ( 'NONE', #82223, .T. ) ;
#38172=DIRECTION ( 'NONE',  ( 1.000000000000000000, -0.000000000000000000, 1.224646799147353207E-16 ) ) ;
#38174=LINE ( 'NONE', #11882, #103401 ) ;
#38184=CARTESIAN_POINT ( 'NONE',  ( 41.95590887306681793, 1512.187213306747481, 225.5974093378518148 ) ) ;
#38185=CARTESIAN_POINT ( 'NONE',  ( 16.62993785878378006, 1526.306647125542895, 235.0749286977620045 ) ) ;
#38213=ORIENTED_EDGE ( 'NONE', *, *, #101461, .T. ) ;
#38237=DIRECTION ( 'NONE',  ( 0.000000000000000000, 0.000000000000000000, 1.000000000000000000 ) ) ;
#38243=CARTESIAN_POINT ( 'NONE',  ( -20.60985939166342007, 1525.581535527372353, 181.7364793965089405 ) ) ;
#38255=EDGE_LOOP ( 'NONE', ( #107737, #19940, #8758, #59553, #109830 ) ) ;
#38274=( BOUNDED_SURFACE ( )  B_SPLINE_SURFACE ( 3, 2, ( 
 ( #82316, #49280, #81202 ),
 ( #38652, #72827, #106960 ),
 ( #64439, #5614, #73927 ),
 ( #98555, #21824, #57139 ),
 ( #90148, #91267, #13430 ),
 ( #108057, #73374, #31353 ),
 ( #9466, #109722, #59890 ),
 ( #94559, #86173, #8902 ),
 ( #1091, #84515, #17278 ),
 ( #110820, #33539, #32999 ),
 ( #103514, #26818, #41425 ),
 ( #110263, #50387, #60441 ),
 ( #102411, #25693, #52037 ),
 ( #25141, #24582, #43631 ) ),
 .UNSPECIFIED., .F., .F., .T. ) 
 B_SPLINE_SURFACE_WITH_KNOTS ( ( 4, 2, 2, 2, 2, 2, 4 ),
 ( 3, 3 ),
 ( 2.424276057677587914E-16, 0.0009443072508238471762, 0.001416460876235649605, 0.001888614501647451925, 0.002360768127059254245, 0.002832921752471056782, 0.003777229003294661422 ),
 ( 0.000000000000000000, 1.000000000000000000 ),
 .UNSPECIFIED. ) 
 GEOMETRIC_REPRESENTATION_ITEM ( )  RATIONAL_B_SPLINE_SURFACE ( (
 ( 1.000000000000000000, 0.9376006582765967767, 1.000000000000000000),
 ( 1.000000000000000000, 0.9283977714668572023, 1.000000000000000000),
 ( 1.000000000000000000, 0.9189750060570894830, 1.000000000000000000),
 ( 1.000000000000000000, 0.9042792056081997432, 1.000000000000000000),
 ( 1.000000000000000000, 0.8992469033881916873, 1.000000000000000000),
 ( 1.000000000000000000, 0.8891280264643571796, 1.000000000000000000),
 ( 1.000000000000000000, 0.8840337471673896941, 1.000000000000000000),
 ( 1.000000000000000000, 0.8736395124165009518, 1.000000000000000000),
 ( 1.000000000000000000, 0.8683406746555940581, 1.000000000000000000),
 ( 1.000000000000000000, 0.8573361860704523663, 1.000000000000000000),
 ( 1.000000000000000000, 0.8516508399500207771, 1.000000000000000000),
 ( 1.000000000000000000, 0.8340914917058259714, 1.000000000000000000),
 ( 1.000000000000000000, 0.8215597275867865257, 1.000000000000000000),
 ( 1.000000000000000000, 0.8070209408750127489, 1.000000000000000000) ) ) 
 REPRESENTATION_ITEM ( '' )  SURFACE ( )  );
#38288=DIRECTION ( 'NONE',  ( 0.000000000000000000, 1.000000000000000000, 0.000000000000000000 ) ) ;
#38294=CARTESIAN_POINT ( 'NONE',  ( 32.38114538885255200, 1523.604703353109926, 216.1203639561428815 ) ) ;
#38331=DIRECTION ( 'NONE',  ( 0.000000000000000000, 0.000000000000000000, 1.000000000000000000 ) ) ;
#38335=ORIENTED_EDGE ( 'NONE', *, *, #74662, .T. ) ;
#38338=ORIENTED_EDGE ( 'NONE', *, *, #55256, .T. ) ;
#38343=CARTESIAN_POINT ( 'NONE',  ( -29.55269881708372637, 1525.821544997590536, 197.1295836072968655 ) ) ;
#38355=ADVANCED_FACE ( 'NONE', ( #79805 ), #89836, .T. ) ;
#38359=CARTESIAN_POINT ( 'NONE',  ( -31.18494820112229249, 1524.152444737676660, 196.3673256080876968 ) ) ;
#38365=DIRECTION ( 'NONE',  ( 0.8672669759446630655, 0.000000000000000000, -0.4978433412588735285 ) ) ;
#38380=ORIENTED_EDGE ( 'NONE', *, *, #61317, .F. ) ;
#38382=CYLINDRICAL_SURFACE ( 'NONE', #99595, 1.000000000000001554 ) ;
#38386=CARTESIAN_POINT ( 'NONE',  ( 3.024787391539411242E-15, 1522.051704408389924, 184.4225825198192013 ) ) ;
#38387=EDGE_CURVE ( 'NONE', #24269, #15596, #11491, .T. ) ;
#38412=VERTEX_POINT ( 'NONE', #20410 ) ;
#38418=CARTESIAN_POINT ( 'NONE',  ( 2.596261494520225366, 1525.907212628473644, 240.7735774411713123 ) ) ;
#38419=CARTESIAN_POINT ( 'NONE',  ( -2.646287650837769956, 1525.055427061254704, 241.6502252480098605 ) ) ;
#38429=ORIENTED_EDGE ( 'NONE', *, *, #38387, .T. ) ;
#38443=DIRECTION ( 'NONE',  ( 0.000000000000000000, 1.000000000000000000, 0.000000000000000000 ) ) ;
#38448=AXIS2_PLACEMENT_3D ( 'NONE', #73962, #50422, #99679 ) ;
#38453=CARTESIAN_POINT ( 'NONE',  ( 34.18677586421061676, 1522.906561336852974, 198.4504086008707873 ) ) ;
#38458=B_SPLINE_CURVE_WITH_KNOTS ( 'NONE', 3,
 ( #35448, #87521, #36011, #62339, #37655, #88079 ),
 .UNSPECIFIED., .F., .F.,
 ( 4, 2, 4 ),
 ( -1.285435071110569928E-05, 0.001079388306740477988, 0.002171630964192061610 ),
 .UNSPECIFIED. ) ;
#38463=DIRECTION ( 'NONE',  ( -0.2054769195713296581, 0.000000000000000000, 0.9786619618251632957 ) ) ;
#38471=VERTEX_POINT ( 'NONE', #57372 ) ;
#38472=DIRECTION ( 'NONE',  ( 0.000000000000000000, 0.000000000000000000, -1.000000000000000000 ) ) ;
#38486=AXIS2_PLACEMENT_3D ( 'NONE', #8457, #77343, #68963 ) ;
#38492=ORIENTED_EDGE ( 'NONE', *, *, #11652, .F. ) ;
#38516=CARTESIAN_POINT ( 'NONE',  ( 31.23437356469446868, 1511.187213306747708, 222.8968241038843701 ) ) ;
#38518=CARTESIAN_POINT ( 'NONE',  ( 32.38845792001183810, 1523.456924617338700, 202.1182848006293113 ) ) ;
#38519=EDGE_CURVE ( 'NONE', #65949, #23788, #2834, .T. ) ;
#38528=DIRECTION ( 'NONE',  ( 0.9970203751124365743, 0.07713865185920996959, 0.000000000000000000 ) ) ;
#38530=AXIS2_PLACEMENT_3D ( 'NONE', #92398, #23548, #25188 ) ;
#38543=DIRECTION ( 'NONE',  ( 0.7414773880254614813, 0.000000000000000000, -0.6709778558543786353 ) ) ;
#38549=VECTOR ( 'NONE', #6175, 1000.000000000000000 ) ;
#38566=CARTESIAN_POINT ( 'NONE',  ( -18.19590854888185305, 1522.382868172863937, 180.0410247165186490 ) ) ;
#38575=DIRECTION ( 'NONE',  ( 0.000000000000000000, 0.000000000000000000, -1.000000000000000000 ) ) ;
#38580=CARTESIAN_POINT ( 'NONE',  ( 19.07966196791819513, 1524.244163922424377, 239.0023935151726562 ) ) ;
#38592=CARTESIAN_POINT ( 'NONE',  ( 2.596261494520241353, 1525.907212628473644, 177.4701144822246874 ) ) ;
#38614=ORIENTED_EDGE ( 'NONE', *, *, #110148, .T. ) ;
#38615=DIRECTION ( 'NONE',  ( -0.8672669759446604010, 0.000000000000000000, 0.4978433412588780804 ) ) ;
#38631=ORIENTED_EDGE ( 'NONE', *, *, #25557, .F. ) ;
#38641=CARTESIAN_POINT ( 'NONE',  ( 0.8350686643532179154, 1526.382868172863937, 177.3106345060153046 ) ) ;
#38647=ADVANCED_FACE ( 'NONE', ( #58318 ), #7350, .T. ) ;
#38652=CARTESIAN_POINT ( 'NONE',  ( 29.41653895341896074, 1525.790286462512086, 196.6777156381645284 ) ) ;
#38656=ADVANCED_FACE ( 'NONE', ( #91366 ), #73476, .F. ) ;
#38676=CARTESIAN_POINT ( 'NONE',  ( -21.38516915557942255, 1522.382868172863937, 237.8497028174240313 ) ) ;
#38685=CARTESIAN_POINT ( 'NONE',  ( -31.34137657934000387, 1523.382868172864164, 221.9025654077414345 ) ) ;
#38690=CARTESIAN_POINT ( 'NONE',  ( 16.68062049856716555, 1526.382868172863709, 181.4122394607864521 ) ) ;
#38703=CARTESIAN_POINT ( 'NONE',  ( -17.84338787571900298, 1523.382868172864164, 237.8836641337663309 ) ) ;
#38707=CARTESIAN_POINT ( 'NONE',  ( -18.37487226820823949, 1526.382868172863937, 235.7398599686418663 ) ) ;
#38710=TOROIDAL_SURFACE ( 'NONE', #76291, 24.69926344187880929, 1.000000000000000000 ) ;
#38713=VERTEX_POINT ( 'NONE', #31861 ) ;
#38729=CARTESIAN_POINT ( 'NONE',  ( 17.84338787571943641, 1523.382868172864164, 237.8836641337660467 ) ) ;
#38738=ORIENTED_EDGE ( 'NONE', *, *, #43461, .F. ) ;
#38751=LINE ( 'NONE', #72928, #63477 ) ;
#38767=CIRCLE ( 'NONE', #11929, 2.000000000000001776 ) ;
#38777=ORIENTED_EDGE ( 'NONE', *, *, #44604, .F. ) ;
#38788=DIRECTION ( 'NONE',  ( -0.7414773880254666993, 0.000000000000000000, 0.6709778558543727511 ) ) ;
#38801=CARTESIAN_POINT ( 'NONE',  ( -17.17241001986523941, 1512.187213306747481, 181.6185504016045797 ) ) ;
#38803=ORIENTED_EDGE ( 'NONE', *, *, #9743, .T. ) ;
#38804=CARTESIAN_POINT ( 'NONE',  ( -2.131986625821266745, 1526.000688113749902, 177.5511380990283499 ) ) ;
#38808=CARTESIAN_POINT ( 'NONE',  ( 32.02808312589922224, 1511.187213306747708, 219.9649204700462235 ) ) ;
#38842=CARTESIAN_POINT ( 'NONE',  ( 31.52384429374465569, 1525.730671948511599, 217.0357143952193724 ) ) ;
#38857=AXIS2_PLACEMENT_3D ( 'NONE', #107133, #72997, #39381 ) ;
#38865=ORIENTED_EDGE ( 'NONE', *, *, #99821, .F. ) ;
#38883=ORIENTED_EDGE ( 'NONE', *, *, #14136, .T. ) ;
#38900=EDGE_CURVE ( 'NONE', #64568, #74476, #18441, .T. ) ;
#38914=CARTESIAN_POINT ( 'NONE',  ( 28.27139721233031722, 1526.382868172864164, 198.6830693683572235 ) ) ;
#38939=CARTESIAN_POINT ( 'NONE',  ( 21.84020450222056908, 1523.382868172864164, 234.9798068779740277 ) ) ;
#38954=ORIENTED_EDGE ( 'NONE', *, *, #96530, .F. ) ;
#38957=CARTESIAN_POINT ( 'NONE',  ( 3.350338079455601026, 1523.604703353109699, 242.0808062845893289 ) ) ;
#38959=CARTESIAN_POINT ( 'NONE',  ( -17.19739463999606599, 1525.960063244516959, 236.2603809477411971 ) ) ;
#38962=CARTESIAN_POINT ( 'NONE',  ( -3.355802132529050574, 1523.843271061949963, 242.0624703644778606 ) ) ;
#38966=CYLINDRICAL_SURFACE ( 'NONE', #11006, 33.13701971169416538 ) ;
#38976=ORIENTED_EDGE ( 'NONE', *, *, #108860, .F. ) ;
#38993=VECTOR ( 'NONE', #81379, 1000.000000000000000 ) ;
#38995=CARTESIAN_POINT ( 'NONE',  ( 30.99338347247808656, 1526.382868172863937, 199.8717226395764044 ) ) ;
#38998=VERTEX_POINT ( 'NONE', #27826 ) ;
#39011=ORIENTED_EDGE ( 'NONE', *, *, #66682, .F. ) ;
#39019=CARTESIAN_POINT ( 'NONE',  ( 0.000000000000000000, 1523.382868172864164, 209.1218459616979999 ) ) ;
#39034=LINE ( 'NONE', #82151, #942 ) ;
#39046=EDGE_LOOP ( 'NONE', ( #70811, #106379, #52505, #87191, #36416 ) ) ;
#39050=ORIENTED_EDGE ( 'NONE', *, *, #22759, .T. ) ;
#39059=DIRECTION ( 'NONE',  ( -0.8090169943749422332, 0.000000000000000000, 0.5877852522924802425 ) ) ;
#39063=CIRCLE ( 'NONE', #26600, 1.999999999999999556 ) ;
#39072=DIRECTION ( 'NONE',  ( 0.000000000000000000, 0.000000000000000000, -1.000000000000000000 ) ) ;
#39078=CARTESIAN_POINT ( 'NONE',  ( -22.08622291488090639, 1523.456924617336426, 184.4183880513689928 ) ) ;
#39088=CIRCLE ( 'NONE', #33737, 2.000000000000001776 ) ;
#39090=CARTESIAN_POINT ( 'NONE',  ( -30.60461244942468184, 1523.621879633028584, 221.8232741897821541 ) ) ;
#39099=CYLINDRICAL_SURFACE ( 'NONE', #24607, 2.000000000000001776 ) ;
#39100=ORIENTED_EDGE ( 'NONE', *, *, #2268, .F. ) ;
#39103=EDGE_CURVE ( 'NONE', #50508, #105303, #76188, .T. ) ;
#39114=CARTESIAN_POINT ( 'NONE',  ( 1.771001175045461284, 1526.211523310372513, 177.6852190580647459 ) ) ;
#39115=CARTESIAN_POINT ( 'NONE',  ( 3.347801439296141712, 1523.382868172864164, 242.0893193391992497 ) ) ;
#39133=ADVANCED_FACE ( 'NONE', ( #76523 ), #83274, .T. ) ;
#39186=ORIENTED_EDGE ( 'NONE', *, *, #91388, .T. ) ;
#39187=CARTESIAN_POINT ( 'NONE',  ( 0.4151546846821905778, 1522.382868172863937, 173.3106345060153046 ) ) ;
#39215=TOROIDAL_SURFACE ( 'NONE', #21375, 30.13701971169416538, 3.000000000000000000 ) ;
#39222=EDGE_CURVE ( 'NONE', #56035, #20284, #74371, .T. ) ;
#39226=CARTESIAN_POINT ( 'NONE',  ( -22.03465957473791192, 1522.644714754857205, 235.4136513321467987 ) ) ;
#39227=CARTESIAN_POINT ( 'NONE',  ( 19.53786426059039982, 1501.977400791986611, 236.7197124308265188 ) ) ;
#39229=FACE_OUTER_BOUND ( 'NONE', #99203, .T. ) ;
#39233=CARTESIAN_POINT ( 'NONE',  ( 20.87481493262672672, 1525.712830164893376, 184.1764553469176633 ) ) ;
#39237=( BOUNDED_SURFACE ( )  B_SPLINE_SURFACE ( 3, 2, ( 
 ( #61203, #76309, #51667 ),
 ( #52229, #16912, #9102 ),
 ( #69039, #67931, #69595 ),
 ( #109910, #33191, #101479 ),
 ( #24766, #93096, #16368 ),
 ( #25325, #50566, #84692 ),
 ( #87481, #53906, #44941 ),
 ( #29216, #35968, #3486 ),
 ( #27558, #105938, #71817 ),
 ( #2941, #79638, #52774 ),
 ( #37615, #89115, #63406 ),
 ( #70159, #10203, #1834 ),
 ( #11325, #45497, #11866 ),
 ( #88041, #86912, #37061 ) ),
 .UNSPECIFIED., .F., .F., .F. ) 
 B_SPLINE_SURFACE_WITH_KNOTS ( ( 4, 2, 2, 2, 2, 2, 4 ),
 ( 3, 3 ),
 ( 0.000000000000000000, 0.0009440840677145004387, 0.001416126101571750767, 0.001888168135429000877, 0.002360210169286251422, 0.002832252203143501533, 0.003776336270858001755 ),
 ( 0.000000000000000000, 1.000000000000000000 ),
 .UNSPECIFIED. ) 
 GEOMETRIC_REPRESENTATION_ITEM ( )  RATIONAL_B_SPLINE_SURFACE ( (
 ( 1.000000000000000000, 0.8070209408750090851, 1.000000000000000000),
 ( 1.000000000000000000, 0.8215603905292898634, 1.000000000000000000),
 ( 1.000000000000000000, 0.8340988699049266542, 1.000000000000000000),
 ( 1.000000000000000000, 0.8516751610464631250, 1.000000000000000000),
 ( 1.000000000000000000, 0.8573697395152763967, 1.000000000000000000),
 ( 1.000000000000000000, 0.8683586635663552711, 1.000000000000000000),
 ( 1.000000000000000000, 0.8736518481708266393, 1.000000000000000000),
 ( 1.000000000000000000, 0.8840377753030468355, 1.000000000000000000),
 ( 1.000000000000000000, 0.8891294171307794203, 1.000000000000000000),
 ( 1.000000000000000000, 0.8992456600573223158, 1.000000000000000000),
 ( 1.000000000000000000, 0.9042785869249978514, 1.000000000000000000),
 ( 1.000000000000000000, 0.9189749222844358911, 1.000000000000000000),
 ( 1.000000000000000000, 0.9283978182344505559, 1.000000000000000000),
 ( 1.000000000000000000, 0.9376006582765954445, 1.000000000000000000) ) ) 
 REPRESENTATION_ITEM ( '' )  SURFACE ( )  );
#39243=CARTESIAN_POINT ( 'NONE',  ( 18.00465857451045792, 1523.390106123591067, 180.2140906788903862 ) ) ;
#39250=CARTESIAN_POINT ( 'NONE',  ( -17.10337015679643713, 1524.478200376951008, 180.9725626400690146 ) ) ;
#39267=ADVANCED_FACE ( 'NONE', ( #69695 ), #84702, .F. ) ;
#39268=CARTESIAN_POINT ( 'NONE',  ( 1.439851189671143228, 1526.382868172864164, 178.7402778767489906 ) ) ;
#39278=CIRCLE ( 'NONE', #76855, 1.000000000000000888 ) ;
#39287=CARTESIAN_POINT ( 'NONE',  ( 0.000000000000000000, 1522.051704408389924, 209.1218459616979999 ) ) ;
#39294=ADVANCED_FACE ( 'NONE', ( #98712 ), #63505, .T. ) ;
#39299=ORIENTED_EDGE ( 'NONE', *, *, #50184, .T. ) ;
#39303=DIRECTION ( 'NONE',  ( 0.000000000000000000, 0.000000000000000000, -1.000000000000000000 ) ) ;
#39318=AXIS2_PLACEMENT_3D ( 'NONE', #104448, #96047, #54086 ) ;
#39319=CARTESIAN_POINT ( 'NONE',  ( -16.73628186595804479, 1526.382868172863937, 234.1845039693045862 ) ) ;
#39327=AXIS2_PLACEMENT_3D ( 'NONE', #81679, #108554, #31844 ) ;
#39338=DIRECTION ( 'NONE',  ( 0.000000000000000000, 1.000000000000000000, 0.000000000000000000 ) ) ;
#39341=CARTESIAN_POINT ( 'NONE',  ( -17.78793056501397984, 1523.919943579690425, 180.4102122295458059 ) ) ;
#39365=TOROIDAL_SURFACE ( 'NONE', #98340, 2.000000000000000000, 1.000000000000000000 ) ;
#39377=ORIENTED_EDGE ( 'NONE', *, *, #82409, .T. ) ;
#39380=CARTESIAN_POINT ( 'NONE',  ( 18.51436573157356946, 1511.187213306747708, 181.1015051776552696 ) ) ;
#39381=DIRECTION ( 'NONE',  ( 0.000000000000000000, 0.000000000000000000, 1.000000000000000000 ) ) ;
#39393=CIRCLE ( 'NONE', #92, 2.000000000000001776 ) ;
#39396=CARTESIAN_POINT ( 'NONE',  ( -3.246772394788723481, 1511.187213306747708, 177.1492560608742224 ) ) ;
#39407=CARTESIAN_POINT ( 'NONE',  ( 32.54505059146715951, 1524.547395018737916, 217.0833365843165268 ) ) ;
#39420=CIRCLE ( 'NONE', #5453, 1.000000000000000888 ) ;
#39423=CARTESIAN_POINT ( 'NONE',  ( 0.000000000000000000, 1523.382868172864164, 209.1218459616979999 ) ) ;
#39427=EDGE_CURVE ( 'NONE', #48513, #91956, #50932, .T. ) ;
#39432=ORIENTED_EDGE ( 'NONE', *, *, #60401, .F. ) ;
#39443=AXIS2_PLACEMENT_3D ( 'NONE', #46006, #20219, #4004 ) ;
#39444=CARTESIAN_POINT ( 'NONE',  ( -32.85805783624315524, 1523.678648413191922, 201.0453875934059340 ) ) ;
#39454=CARTESIAN_POINT ( 'NONE',  ( 21.50863349123601509, 1524.374142163904253, 234.1185027681734709 ) ) ;
#39456=VERTEX_POINT ( 'NONE', #5208 ) ;
#39464=VERTEX_POINT ( 'NONE', #56164 ) ;
#39477=CARTESIAN_POINT ( 'NONE',  ( -31.32995031131208918, 1523.678648413191695, 196.3423562208917872 ) ) ;
#39484=CIRCLE ( 'NONE', #55657, 32.13701971169416538 ) ;
#39507=CARTESIAN_POINT ( 'NONE',  ( 21.53712143570556137, 1523.621879633028811, 183.9400870382961841 ) ) ;
#39509=CARTESIAN_POINT ( 'NONE',  ( 33.93019615848559312, 1522.906561336852974, 220.5829544588082740 ) ) ;
#39513=ORIENTED_EDGE ( 'NONE', *, *, #10703, .T. ) ;
#39520=AXIS2_PLACEMENT_3D ( 'NONE', #65573, #99684, #22977 ) ;
#39532=CARTESIAN_POINT ( 'NONE',  ( -29.99620953741502660, 1526.382868172863937, 198.4974435154502999 ) ) ;
#39541=EDGE_CURVE ( 'NONE', #40681, #92786, #59895, .T. ) ;
#39549=VERTEX_POINT ( 'NONE', #33153 ) ;
#39550=VERTEX_POINT ( 'NONE', #5771 ) ;
#39566=CARTESIAN_POINT ( 'NONE',  ( 34.09079054514428719, 1524.667648926107404, 200.3377533957251728 ) ) ;
#39575=CIRCLE ( 'NONE', #75318, 0.9999999999999976685 ) ;
#39584=ORIENTED_EDGE ( 'NONE', *, *, #98917, .T. ) ;
#39595=ORIENTED_EDGE ( 'NONE', *, *, #49377, .T. ) ;
#39600=CARTESIAN_POINT ( 'NONE',  ( -2.038847259689231084, 1501.977400791986611, 244.9330574173806951 ) ) ;
#39623=VERTEX_POINT ( 'NONE', #65681 ) ;
#39634=CARTESIAN_POINT ( 'NONE',  ( 32.86802468363470098, 1523.481610118012213, 201.0396662541351986 ) ) ;
#39651=CARTESIAN_POINT ( 'NONE',  ( -21.84020450222075738, 1523.382868172864164, 183.2638850454220858 ) ) ;
#39672=CARTESIAN_POINT ( 'NONE',  ( 31.29224244793351417, 1525.661276915132476, 216.2849148480870838 ) ) ;
#39675=VECTOR ( 'NONE', #107677, 1000.000000000000000 ) ;
#39679=ORIENTED_EDGE ( 'NONE', *, *, #18018, .F. ) ;
#39696=CARTESIAN_POINT ( 'NONE',  ( 19.39983987835423918, 1522.382868172863937, 239.2921289694223503 ) ) ;
#39698=AXIS2_PLACEMENT_3D ( 'NONE', #30056, #72637, #64247 ) ;
#39699=DIRECTION ( 'NONE',  ( -0.8090169943749507819, 0.000000000000000000, -0.5877852522924685852 ) ) ;
#39710=EDGE_CURVE ( 'NONE', #100597, #43261, #15771, .T. ) ;
#39730=CARTESIAN_POINT ( 'NONE',  ( 21.12212911287032213, 1511.187213306747708, 235.8226600804184159 ) ) ;
#39734=VERTEX_POINT ( 'NONE', #82473 ) ;
#39737=ORIENTED_EDGE ( 'NONE', *, *, #70715, .T. ) ;
#39741=CARTESIAN_POINT ( 'NONE',  ( 0.4151546846821903003, 1512.187213306747481, 173.3106345060153046 ) ) ;
#39743=EDGE_CURVE ( 'NONE', #47552, #47062, #104560, .T. ) ;
#39757=ADVANCED_FACE ( 'NONE', ( #69000 ), #78481, .T. ) ;
#39779=EDGE_CURVE ( 'NONE', #38412, #20993, #69556, .T. ) ;
#39781=EDGE_LOOP ( 'NONE', ( #47852, #4562, #64531, #50305 ) ) ;
#39791=ADVANCED_FACE ( 'NONE', ( #86871 ), #27516, .T. ) ;
#39794=DIRECTION ( 'NONE',  ( 0.000000000000000000, 1.000000000000000000, 0.000000000000000000 ) ) ;
#39796=CARTESIAN_POINT ( 'NONE',  ( 28.96738428617755190, 1526.189899547014647, 220.8024311359775425 ) ) ;
#39812=CARTESIAN_POINT ( 'NONE',  ( -16.86500409606249562, 1525.697947650550304, 181.8505186805997482 ) ) ;
#39813=CARTESIAN_POINT ( 'NONE',  ( -32.97913964219424088, 1512.187213306747481, 220.2739374644216355 ) ) ;
#39827=CARTESIAN_POINT ( 'NONE',  ( -21.84020450222019250, 1523.382868172864164, 234.9798068779743403 ) ) ;
#39828=EDGE_LOOP ( 'NONE', ( #38954, #92577, #21794, #76364 ) ) ;
#39829=DIRECTION ( 'NONE',  ( -0.8386695113602914420, -0.4884709562386498338, -0.2408932868014154460 ) ) ;
#39840=LINE ( 'NONE', #14626, #45086 ) ;
#39848=CARTESIAN_POINT ( 'NONE',  ( 19.53786426059019021, 1501.977400791986611, 181.5239794925693388 ) ) ;
#39849=EDGE_CURVE ( 'NONE', #48271, #82569, #3994, .T. ) ;
#39850=CARTESIAN_POINT ( 'NONE',  ( -32.20549126534956486, 1524.425415513989947, 216.0989951694419346 ) ) ;
#39854=ORIENTED_EDGE ( 'NONE', *, *, #72068, .T. ) ;
#39868=VERTEX_POINT ( 'NONE', #28066 ) ;
#39874=CARTESIAN_POINT ( 'NONE',  ( -20.71343476517555615, 1524.726013923371283, 179.9059455038196802 ) ) ;
#39879=CARTESIAN_POINT ( 'NONE',  ( -3.348647037815654315, 1523.530870145311155, 242.0864809827354520 ) ) ;
#39896=DIRECTION ( 'NONE',  ( -0.3090169943749515036, -0.000000000000000000, -0.9510565162951521989 ) ) ;
#39901=CARTESIAN_POINT ( 'NONE',  ( -22.03465957474590908, 1522.382868172863937, 182.8300405912331144 ) ) ;
#39907=ORIENTED_EDGE ( 'NONE', *, *, #56606, .T. ) ;
#39918=CARTESIAN_POINT ( 'NONE',  ( -17.19757137884673526, 1524.059547553519224, 237.3738383026851011 ) ) ;
#39930=VERTEX_POINT ( 'NONE', #49843 ) ;
#39953=CARTESIAN_POINT ( 'NONE',  ( -29.86461515634900010, 1525.960063244516959, 220.9690070206027031 ) ) ;
#39956=CARTESIAN_POINT ( 'NONE',  ( -19.98413504154930109, 1526.143142182166912, 184.9530087057032119 ) ) ;
#39967=FACE_OUTER_BOUND ( 'NONE', #75467, .T. ) ;
#40000=CARTESIAN_POINT ( 'NONE',  ( 21.83550407203923527, 1523.678648413191922, 234.9693198511250785 ) ) ;
#40036=CARTESIAN_POINT ( 'NONE',  ( -22.07680818022615910, 1523.847248782568613, 233.7985790283582901 ) ) ;
#40044=( BOUNDED_CURVE ( )  B_SPLINE_CURVE ( 3, ( #14941, #93313, #23891, #50770 ),
 .UNSPECIFIED., .F., .F. ) 
 B_SPLINE_CURVE_WITH_KNOTS ( ( 4, 4 ),
 ( 3.141592653589793116, 4.712388980384689674 ),
 .UNSPECIFIED. ) 
 CURVE ( )  GEOMETRIC_REPRESENTATION_ITEM ( )  RATIONAL_B_SPLINE_CURVE ( ( 1.000000000000000000, 0.8047378541243649375, 0.8047378541243649375, 1.000000000000000000 ) ) 
 REPRESENTATION_ITEM ( '' )  );
#40046=CARTESIAN_POINT ( 'NONE',  ( 33.28034951413924603, 1512.187213306747481, 200.8029765415137717 ) ) ;
#40053=CARTESIAN_POINT ( 'NONE',  ( 33.34040796508655546, 1523.342713519622293, 222.1177029624608110 ) ) ;
#40054=ORIENTED_EDGE ( 'NONE', *, *, #82268, .T. ) ;
#40063=EDGE_CURVE ( 'NONE', #41473, #85993, #62378, .T. ) ;
#40081=AXIS2_PLACEMENT_3D ( 'NONE', #39019, #83794, #41244 ) ;
#40124=CARTESIAN_POINT ( 'NONE',  ( 0.000000000000000000, 1518.913060387330006, 209.1218459616979999 ) ) ;
#40129=ORIENTED_EDGE ( 'NONE', *, *, #52970, .F. ) ;
#40136=AXIS2_PLACEMENT_3D ( 'NONE', #24819, #84198, #102631 ) ;
#40139=ORIENTED_EDGE ( 'NONE', *, *, #102056, .F. ) ;
#40144=FACE_OUTER_BOUND ( 'NONE', #97577, .T. ) ;
#40151=VERTEX_POINT ( 'NONE', #104904 ) ;
#40153=CARTESIAN_POINT ( 'NONE',  ( -29.36007807473448139, 1526.208281990539263, 220.5288989449499866 ) ) ;
#40156=DIRECTION ( 'NONE',  ( 0.9125304618753961039, 0.000000000000000000, -0.4090087482554332632 ) ) ;
#40167=DIRECTION ( 'NONE',  ( 0.9149707217702669482, 0.000000000000000000, 0.4035202328300239172 ) ) ;
#40171=EDGE_LOOP ( 'NONE', ( #39432, #82182, #12869, #38022 ) ) ;
#40174=EDGE_CURVE ( 'NONE', #77339, #47552, #29496, .T. ) ;
#40182=FACE_OUTER_BOUND ( 'NONE', #2212, .T. ) ;
#40189=DIRECTION ( 'NONE',  ( -0.4090087482554183862, 0.000000000000000000, 0.9125304618754026542 ) ) ;
#40209=AXIS2_PLACEMENT_3D ( 'NONE', #10164, #95824, #19092 ) ;
#40223=ORIENTED_EDGE ( 'NONE', *, *, #53740, .F. ) ;
#40240=AXIS2_PLACEMENT_3D ( 'NONE', #98252, #5300, #46783 ) ;
#40247=DIRECTION ( 'NONE',  ( 0.000000000000000000, 0.000000000000000000, 1.000000000000000000 ) ) ;
#40257=CARTESIAN_POINT ( 'NONE',  ( 29.00779973304117831, 1526.382868172864164, 200.9494832830835378 ) ) ;
#40295=ORIENTED_EDGE ( 'NONE', *, *, #93471, .T. ) ;
#40324=DIRECTION ( 'NONE',  ( 0.6709778558543625371, 0.000000000000000000, -0.7414773880254761362 ) ) ;
#40339=CARTESIAN_POINT ( 'NONE',  ( -0.7251570665222376588, 1526.278758871496848, 176.2636429491666945 ) ) ;
#40346=CARTESIAN_POINT ( 'NONE',  ( -33.28034951413921760, 1501.977400791986611, 217.4407153818824838 ) ) ;
#40351=CARTESIAN_POINT ( 'NONE',  ( -16.50400130224779360, 1525.907212628473644, 181.9890130758379030 ) ) ;
#40359=CARTESIAN_POINT ( 'NONE',  ( -22.03465957474591619, 1522.382868172863937, 182.8300405912331144 ) ) ;
#40366=DIRECTION ( 'NONE',  ( 0.000000000000000000, 0.000000000000000000, 1.000000000000000000 ) ) ;
#40388=DIRECTION ( 'NONE',  ( 0.000000000000000000, 1.000000000000000000, 0.000000000000000000 ) ) ;
#40394=ORIENTED_EDGE ( 'NONE', *, *, #38519, .T. ) ;
#40403=CARTESIAN_POINT ( 'NONE',  ( 20.20959865099491992, 1501.977400791986611, 236.2316688286738611 ) ) ;
#40407=CARTESIAN_POINT ( 'NONE',  ( -30.90487439922522483, 1525.907212628473872, 216.4335774778785151 ) ) ;
#40459=B_SPLINE_CURVE_WITH_KNOTS ( 'NONE', 3,
 ( #53767, #61597, #45354, #1689 ),
 .UNSPECIFIED., .F., .F.,
 ( 4, 4 ),
 ( 0.000000000000000000, 0.0002220129587134777205 ),
 .UNSPECIFIED. ) ;
#40460=CARTESIAN_POINT ( 'NONE',  ( -1.191524307911313807, 1526.382868172864164, 179.0083900503168479 ) ) ;
#40469=ADVANCED_FACE ( 'NONE', ( #38127 ), #20530, .T. ) ;
#40473=ORIENTED_EDGE ( 'NONE', *, *, #44865, .F. ) ;
#40479=AXIS2_PLACEMENT_3D ( 'NONE', #23877, #109568, #92750 ) ;
#40502=CARTESIAN_POINT ( 'NONE',  ( 0.000000000000000000, 1518.913060387330006, 209.1218459616979999 ) ) ;
#40510=CARTESIAN_POINT ( 'NONE',  ( 31.32995031131198616, 1523.678648413191695, 221.9013357025044115 ) ) ;
#40515=CARTESIAN_POINT ( 'NONE',  ( 16.49279218151955462, 1525.408327360769590, 236.9553615728405589 ) ) ;
#40517=CARTESIAN_POINT ( 'NONE',  ( -29.00779973304142345, 1526.382868172863937, 200.9494832830838789 ) ) ;
#40527=CIRCLE ( 'NONE', #69169, 24.33258347882036432 ) ;
#40534=ORIENTED_EDGE ( 'NONE', *, *, #92242, .F. ) ;
#40552=ADVANCED_FACE ( 'NONE', ( #23520 ), #30823, .T. ) ;
#40565=VERTEX_POINT ( 'NONE', #65555 ) ;
#40573=VERTEX_POINT ( 'NONE', #99665 ) ;
#40583=CARTESIAN_POINT ( 'NONE',  ( -20.92767404034479028, 1511.187213306747708, 235.3888156262297571 ) ) ;
#40605=CARTESIAN_POINT ( 'NONE',  ( 31.76119286153743815, 1522.906363951597314, 221.9477464134155866 ) ) ;
#40613=CARTESIAN_POINT ( 'NONE',  ( 0.000000000000000000, 1518.913060387330006, 209.1218459616979999 ) ) ;
#40616=EDGE_CURVE ( 'NONE', #108592, #80761, #9762, .T. ) ;
#40624=VERTEX_POINT ( 'NONE', #12237 ) ;
#40628=CARTESIAN_POINT ( 'NONE',  ( 32.80315919379400214, 1523.919943579690425, 201.0769014459399102 ) ) ;
#40634=CARTESIAN_POINT ( 'NONE',  ( 16.50400130224750583, 1525.907212628473644, 181.9890130758377040 ) ) ;
#40647=CARTESIAN_POINT ( 'NONE',  ( 19.53786426059019021, 1522.382868172863937, 181.5239794925693388 ) ) ;
#40654=CIRCLE ( 'NONE', #81801, 2.000000000000003997 ) ;
#40664=VERTEX_POINT ( 'NONE', #16074 ) ;
#40681=VERTEX_POINT ( 'NONE', #32355 ) ;
#40683=VERTEX_POINT ( 'NONE', #66534 ) ;
#40686=CARTESIAN_POINT ( 'NONE',  ( -20.69714064973426559, 1525.848198008145346, 184.2818650771049533 ) ) ;
#40700=DIRECTION ( 'NONE',  ( 0.06728379684272006722, -0.9969860201949397593, -0.03862338952348245980 ) ) ;
#40713=DIRECTION ( 'NONE',  ( 0.000000000000000000, 1.000000000000000000, 0.000000000000000000 ) ) ;
#40718=CARTESIAN_POINT ( 'NONE',  ( 21.41971086555086501, 1511.187213306747708, 185.1638823089577670 ) ) ;
#40722=CARTESIAN_POINT ( 'NONE',  ( 22.08523867432350585, 1523.530870145309564, 233.8225105631262863 ) ) ;
#40736=VERTEX_POINT ( 'NONE', #96682 ) ;
#40750=DIRECTION ( 'NONE',  ( -0.000000000000000000, -1.000000000000000000, -0.000000000000000000 ) ) ;
#40753=DIRECTION ( 'NONE',  ( 0.000000000000000000, 0.000000000000000000, 1.000000000000000000 ) ) ;
#40764=AXIS2_PLACEMENT_3D ( 'NONE', #12721, #20012, #64250 ) ;
#40780=CARTESIAN_POINT ( 'NONE',  ( 30.51231035492521571, 1526.382868172863937, 218.1578534183718432 ) ) ;
#40784=CARTESIAN_POINT ( 'NONE',  ( -32.38114538885245963, 1523.604703353109699, 216.1203639561433647 ) ) ;
#40789=CYLINDRICAL_SURFACE ( 'NONE', #3593, 1.000000000000000888 ) ;
#40795=CARTESIAN_POINT ( 'NONE',  ( -33.23571934791658578, 1511.187213306747708, 219.4842663281467026 ) ) ;
#40818=DIRECTION ( 'NONE',  ( 0.000000000000000000, 0.000000000000000000, 1.000000000000000000 ) ) ;
#40825=LINE ( 'NONE', #22342, #99094 ) ;
#40837=TOROIDAL_SURFACE ( 'NONE', #94453, 32.13701971169416538, 1.000000000000000000 ) ;
#40850=VERTEX_POINT ( 'NONE', #105639 ) ;
#40862=CIRCLE ( 'NONE', #80202, 0.9999999999999880096 ) ;
#40868=CARTESIAN_POINT ( 'NONE',  ( 30.90487439922556945, 1525.907212628473644, 201.8101144455177689 ) ) ;
#40889=CARTESIAN_POINT ( 'NONE',  ( -0.8350686643532179154, 1526.382868172863937, 177.3106345060153046 ) ) ;
#40895=ORIENTED_EDGE ( 'NONE', *, *, #27051, .F. ) ;
#40903=CARTESIAN_POINT ( 'NONE',  ( -16.85976061912589330, 1525.821544997590081, 182.0492613858612856 ) ) ;
#40915=CARTESIAN_POINT ( 'NONE',  ( -18.19590854888122067, 1522.382868172863937, 238.2026672068776918 ) ) ;
#40917=ORIENTED_EDGE ( 'NONE', *, *, #71381, .T. ) ;
#40921=CARTESIAN_POINT ( 'NONE',  ( -1.313045906442075417, 1526.382868172863937, 239.3665138341975194 ) ) ;
#40938=CARTESIAN_POINT ( 'NONE',  ( -30.95751052620429888, 1525.821544997590308, 216.7905424461076223 ) ) ;
#40948=VERTEX_POINT ( 'NONE', #14304 ) ;
#40966=CARTESIAN_POINT ( 'NONE',  ( -19.59884465730855396, 1526.382868172863937, 181.1441328703422187 ) ) ;
#40970=FACE_OUTER_BOUND ( 'NONE', #49615, .T. ) ;
#40981=EDGE_LOOP ( 'NONE', ( #30158, #76910, #35279 ) ) ;
#40985=EDGE_LOOP ( 'NONE', ( #3270, #4506, #36386, #75922, #97911 ) ) ;
#41000=AXIS2_PLACEMENT_3D ( 'NONE', #102913, #1054, #60402 ) ;
#41009=ORIENTED_EDGE ( 'NONE', *, *, #92498, .T. ) ;
#41020=DIRECTION ( 'NONE',  ( 0.000000000000000000, 0.000000000000000000, -1.000000000000000000 ) ) ;
#41026=CARTESIAN_POINT ( 'NONE',  ( -19.53786426058999481, 1512.187213306747481, 238.7197124308268030 ) ) ;
#41033=CIRCLE ( 'NONE', #94664, 1.000000000000071498 ) ;
#41067=CARTESIAN_POINT ( 'NONE',  ( 16.97880994394067500, 1525.055427061254477, 236.9933064582837687 ) ) ;
#41089=CARTESIAN_POINT ( 'NONE',  ( 0.000000000000000000, 1511.187213306747708, 209.1218459616979999 ) ) ;
#41099=ORIENTED_EDGE ( 'NONE', *, *, #65274, .T. ) ;
#41102=ORIENTED_EDGE ( 'NONE', *, *, #59611, .T. ) ;
#41107=AXIS2_PLACEMENT_3D ( 'NONE', #34728, #81009, #21627 ) ;
#41118=AXIS2_PLACEMENT_3D ( 'NONE', #78135, #1438, #9287 ) ;
#41146=CARTESIAN_POINT ( 'NONE',  ( 30.61443310237122617, 1523.382868172863937, 196.4193608261158772 ) ) ;
#41159=CARTESIAN_POINT ( 'NONE',  ( 31.81407709659918481, 1522.644714754857659, 221.9534378623320379 ) ) ;
#41163=VECTOR ( 'NONE', #81535, 1000.000000000000114 ) ;
#41177=CARTESIAN_POINT ( 'NONE',  ( 19.00259723422722047, 1526.382868172571079, 185.3307583833850458 ) ) ;
#41190=CARTESIAN_POINT ( 'NONE',  ( -16.66936639845668822, 1523.456872492435195, 180.4828114240741570 ) ) ;
#41198=ORIENTED_EDGE ( 'NONE', *, *, #41579, .F. ) ;
#41199=CIRCLE ( 'NONE', #39443, 0.9999999999999952260 ) ;
#41203=ORIENTED_EDGE ( 'NONE', *, *, #20828, .F. ) ;
#41205=CARTESIAN_POINT ( 'NONE',  ( -19.98413504154972387, 1526.143142182167139, 233.2906832176993817 ) ) ;
#41232=DIRECTION ( 'NONE',  ( 0.000000000000000000, 0.000000000000000000, -1.000000000000000000 ) ) ;
#41235=VERTEX_POINT ( 'NONE', #89932 ) ;
#41236=LINE ( 'NONE', #14910, #96707 ) ;
#41240=EDGE_CURVE ( 'NONE', #58183, #32684, #91593, .T. ) ;
#41244=DIRECTION ( 'NONE',  ( 0.000000000000000000, 0.000000000000000000, -1.000000000000000000 ) ) ;
#41256=AXIS2_PLACEMENT_3D ( 'NONE', #19152, #8014, #76331 ) ;
#41258=CARTESIAN_POINT ( 'NONE',  ( 30.17514222261037915, 1525.712835404586031, 196.9772729963927702 ) ) ;
#41261=CARTESIAN_POINT ( 'NONE',  ( -28.27139721233027458, 1526.382868172864164, 219.5606225550389468 ) ) ;
#41277=ORIENTED_EDGE ( 'NONE', *, *, #11073, .T. ) ;
#41278=CARTESIAN_POINT ( 'NONE',  ( -28.54400548274723093, 1526.382868172864164, 198.4417401822219631 ) ) ;
#41281=CARTESIAN_POINT ( 'NONE',  ( 33.93019615848955084, 1501.977400791986611, 220.5829544587961095 ) ) ;
#41288=EDGE_CURVE ( 'NONE', #90688, #107214, #50399, .T. ) ;
#41299=CARTESIAN_POINT ( 'NONE',  ( 2.744860007233061339, 1525.790287071781222, 177.2996080414773132 ) ) ;
#41306=CARTESIAN_POINT ( 'NONE',  ( -22.08622291482367572, 1523.382868172864164, 184.4183880513178053 ) ) ;
#41310=FACE_OUTER_BOUND ( 'NONE', #83165, .T. ) ;
#41312=VERTEX_POINT ( 'NONE', #77013 ) ;
#41314=B_SPLINE_CURVE_WITH_KNOTS ( 'NONE', 3,
 ( #96591, #45661, #79799, #35012 ),
 .UNSPECIFIED., .F., .F.,
 ( 4, 4 ),
 ( 0.000000000000000000, 0.0002220129587134776392 ),
 .UNSPECIFIED. ) ;
#41329=CLOSED_SHELL ( 'NONE', ( #58471, #13051, #27636, #52015, #6304, #72642, #23330, #87945, #84548, #41374, #4256, #29795, #51079, #25376, #93883, #109561, #12226, #105359, #90306, #16720, #77524, #33985, #33055, #94786, #17231, #100761, #55232, #106788, #35386, #104975, #105817, #95434, #91061, #85065, #59094, #39757, #69895, #77487, #108905, #11497, #108548, #74689, #28520, #88389, #5649, #21264, #92139, #8673, #73359, #13160, #5169, #75094, #57043, #81558, #25307, #20716, #7754, #5591, #7800, #78844, #8305, #45464, #39791, #68920, #11689, #24984, #39294, #55567, #40552, #67859, #96019, #100334, #99395, #19328, #45138, #70642, #38355, #14093, #79015, #84913, #4041, #58254, #33224, #14455, #103460, #53013, #106376, #4266, #54621, #76316, #103493, #98169, #73540, #95876, #67492, #90218, #43972, #106567, #5625, #28916, #53455, #64211, #43360, #33797, #58353, #87202, #92449, #106823, #37421, #2920, #101828, #9814, #36467, #13278, #21885, #62537, #98196, #55732, #13907, #12406, #61162, #2365, #37744, #52427, #7779, #44894, #24680, #16253, #106873, #2207, #38000, #90059, #15233, #48867, #71999, #13329, #46069, #107912, #87350, #38647, #57299, #80971, #59605, #24956, #79737, #74683, #22807, #13679, #83729, #98435, #60405, #93078, #29608, #82381, #104124, #102046, #91947, #30924, #53205, #39267, #94151, #19853, #95389, #88387, #15112, #3267, #30901, #98743, #45134, #80840, #78692, #53601, #84853, #95124, #2876, #22663, #87341, #56981, #51489, #37873, #50798, #98288, #36983, #94598, #41900, #33743, #41862, #99303, #18650, #18935, #10607, #91067, #75069, #102052, #33081, #87470, #88412, #59065, #107155, #97693, #13207, #66228, #62516, #107140, #26398, #89910, #55634, #2104, #23922, #38656, #70779, #3931, #37732, #73945, #96553, #18628, #16465, #73813, #46785, #69965, #90437, #86903, #96797, #102947, #106977, #86418, #105464, #87951, #110330, #4383, #95376, #27185, #86082, #81615, #68749, #39133, #54987, #78295, #93307, #109135, #7953, #60531, #63784, #5514, #43947, #62560, #101458, #65836, #11117, #75212, #87957, #43264, #10934, #28412, #54078, #76355, #10400, #97551, #108983, #9447, #70635, #97977, #56155, #67927, #50904, #85654, #51631, #67377, #50178, #105636, #17481, #76444, #22526, #68710, #36483, #1019, #9155, #42228, #100079, #98519, #5785, #53710, #1386, #78359, #19578, #109636, #49769, #21424, #93238, #16246, #13062, #49056, #57696, #92488, #47388, #35708, #29787, #101299, #57676, #108529, #40469, #101399, #3114, #46921, #5709, #34179, #68625, #67317, #108687 ) ) ;
#41332=CARTESIAN_POINT ( 'NONE',  ( 32.77044109517639470, 1525.581535527371898, 219.1629015078801785 ) ) ;
#41346=AXIS2_PLACEMENT_3D ( 'NONE', #73014, #107150, #81381 ) ;
#41347=CARTESIAN_POINT ( 'NONE',  ( 2.390047989679215501, 1526.069472839385980, 177.7067300826763301 ) ) ;
#41361=B_SPLINE_CURVE_WITH_KNOTS ( 'NONE', 3,
 ( #43283, #85818, #71277, #63420 ),
 .UNSPECIFIED., .F., .F.,
 ( 4, 4 ),
 ( 0.000000000000000000, 0.0002220129587134771513 ),
 .UNSPECIFIED. ) ;
#41374=ADVANCED_FACE ( 'NONE', ( #43956 ), #55108, .T. ) ;
#41393=DIRECTION ( 'NONE',  ( -0.000000000000000000, -1.000000000000000000, -0.000000000000000000 ) ) ;
#41425=CARTESIAN_POINT ( 'NONE',  ( 31.00914578552986711, 1524.547395018738371, 196.4333264031763520 ) ) ;
#41440=CIRCLE ( 'NONE', #107695, 1.999999999999997335 ) ;
#41455=CARTESIAN_POINT ( 'NONE',  ( -33.36586802512182715, 1512.187213306747481, 201.9069332299493169 ) ) ;
#41458=CARTESIAN_POINT ( 'NONE',  ( -2.682480990172567026, 1524.330813522192102, 176.3761848884415997 ) ) ;
#41460=EDGE_CURVE ( 'NONE', #42124, #97968, #6778, .T. ) ;
#41465=CYLINDRICAL_SURFACE ( 'NONE', #78358, 1.000000000000000888 ) ;
#41473=VERTEX_POINT ( 'NONE', #76317 ) ;
#41479=CARTESIAN_POINT ( 'NONE',  ( 30.51231035492518728, 1526.382868172863937, 200.0858385050239008 ) ) ;
#41480=DIRECTION ( 'NONE',  ( 0.6665120492724535550, 0.000000000000000000, 0.7454942576402816545 ) ) ;
#41490=EDGE_LOOP ( 'NONE', ( #96648, #88006, #79948 ) ) ;
#41496=CARTESIAN_POINT ( 'NONE',  ( 0.8350686643532190256, 1526.382868172863937, 177.3106345060153046 ) ) ;
#41503=AXIS2_PLACEMENT_3D ( 'NONE', #83781, #7076, #41232 ) ;
#41518=B_SPLINE_CURVE_WITH_KNOTS ( 'NONE', 3,
 ( #37363, #47421, #4845, #82105, #62609, #96723 ),
 .UNSPECIFIED., .F., .F.,
 ( 4, 2, 4 ),
 ( -1.131363979620092418E-05, 0.001067788114096002898, 0.002146889867988206399 ),
 .UNSPECIFIED. ) ;
#41529=LINE ( 'NONE', #76227, #35135 ) ;
#41542=( BOUNDED_CURVE ( )  B_SPLINE_CURVE ( 3, ( #12687, #46867, #72606, #106735 ),
 .UNSPECIFIED., .F., .F. ) 
 B_SPLINE_CURVE_WITH_KNOTS ( ( 4, 4 ),
 ( 3.141592653589793116, 4.712388980384689674 ),
 .UNSPECIFIED. ) 
 CURVE ( )  GEOMETRIC_REPRESENTATION_ITEM ( )  RATIONAL_B_SPLINE_CURVE ( ( 1.000000000000000000, 0.8047378541243649375, 0.8047378541243649375, 1.000000000000000000 ) ) 
 REPRESENTATION_ITEM ( '' )  );
#41545=EDGE_LOOP ( 'NONE', ( #45107, #110517, #80029, #38079 ) ) ;
#41555=CARTESIAN_POINT ( 'NONE',  ( 21.44520247467869822, 1525.343727714918259, 233.4338397409588595 ) ) ;
#41568=EDGE_LOOP ( 'NONE', ( #86416, #39011, #17388 ) ) ;
#41579=EDGE_CURVE ( 'NONE', #87392, #79695, #103587, .T. ) ;
#41592=CARTESIAN_POINT ( 'NONE',  ( -32.23393008313268382, 1523.382868172863937, 216.8400319010857515 ) ) ;
#41620=DIRECTION ( 'NONE',  ( 3.469446951953611033E-14, 0.000000000000000000, 1.000000000000000000 ) ) ;
#41624=CARTESIAN_POINT ( 'NONE',  ( 16.86500412378484981, 1525.697946996602695, 181.8505176293797660 ) ) ;
#41638=CARTESIAN_POINT ( 'NONE',  ( -49.24962907673570811, 1526.382868172863937, 407.9033880519289710 ) ) ;
#41645=ORIENTED_EDGE ( 'NONE', *, *, #96661, .T. ) ;
#41684=DIRECTION ( 'NONE',  ( 0.9510565162951566398, 0.000000000000000000, 0.3090169943749382919 ) ) ;
#41693=DIRECTION ( 'NONE',  ( 1.224646799147353454E-16, 0.000000000000000000, -1.000000000000000000 ) ) ;
#41694=CARTESIAN_POINT ( 'NONE',  ( -16.50400130224731754, 1525.907212628473644, 236.2546788475584094 ) ) ;
#41708=CARTESIAN_POINT ( 'NONE',  ( 31.55762699681134009, 1523.390106123591067, 221.9258384720627646 ) ) ;
#41725=CARTESIAN_POINT ( 'NONE',  ( -21.35005939118667584, 1525.163457223744217, 183.8372695436867446 ) ) ;
#41745=ORIENTED_EDGE ( 'NONE', *, *, #21296, .F. ) ;
#41764=CARTESIAN_POINT ( 'NONE',  ( -33.23571934791681315, 1511.187213306747708, 198.7594255952499793 ) ) ;
#41782=CARTESIAN_POINT ( 'NONE',  ( 2.472529913803023227, 1523.678648413191695, 242.8674788698241400 ) ) ;
#41784=ORIENTED_EDGE ( 'NONE', *, *, #53746, .T. ) ;
#41786=CARTESIAN_POINT ( 'NONE',  ( 22.03465957474552184, 1522.862737210649811, 182.8300405912328870 ) ) ;
#41795=EDGE_CURVE ( 'NONE', #7367, #40565, #35407, .T. ) ;
#41805=AXIS2_PLACEMENT_3D ( 'NONE', #73487, #23604, #24139 ) ;
#41823=DIRECTION ( 'NONE',  ( -0.000000000000000000, -1.000000000000000000, -0.000000000000000000 ) ) ;
#41836=VERTEX_POINT ( 'NONE', #15555 ) ;
#41844=CARTESIAN_POINT ( 'NONE',  ( 2.599451791485461349, 1525.231887713385959, 176.7177626659179452 ) ) ;
#41854=ORIENTED_EDGE ( 'NONE', *, *, #18763, .T. ) ;
#41857=DIRECTION ( 'NONE',  ( 0.000000000000000000, 0.000000000000000000, 1.000000000000000000 ) ) ;
#41862=ADVANCED_FACE ( 'NONE', ( #107026 ), #73274, .F. ) ;
#41875=EDGE_CURVE ( 'NONE', #64568, #71455, #83918, .T. ) ;
#41880=FACE_OUTER_BOUND ( 'NONE', #60172, .T. ) ;
#41883=CARTESIAN_POINT ( 'NONE',  ( 18.19590854888164699, 1501.977400791986611, 238.2026672068774644 ) ) ;
#41884=CARTESIAN_POINT ( 'NONE',  ( 0.000000000000000000, 1518.913060387330006, 209.1218459616979999 ) ) ;
#41897=VECTOR ( 'NONE', #12430, 999.9999999999998863 ) ;
#41899=ORIENTED_EDGE ( 'NONE', *, *, #44574, .F. ) ;
#41900=ADVANCED_FACE ( 'NONE', ( #38168 ), #93213, .F. ) ;
#41906=EDGE_CURVE ( 'NONE', #29269, #76248, #100932, .T. ) ;
#41912=DIRECTION ( 'NONE',  ( 0.000000000000000000, 0.000000000000000000, 1.000000000000000000 ) ) ;
#41928=ORIENTED_EDGE ( 'NONE', *, *, #60333, .T. ) ;
#41949=EDGE_CURVE ( 'NONE', #63792, #46121, #64289, .T. ) ;
#41959=DIRECTION ( 'NONE',  ( 0.000000000000000000, 0.000000000000000000, 1.000000000000000000 ) ) ;
#41978=CARTESIAN_POINT ( 'NONE',  ( -32.38845792001078649, 1523.456924617338927, 202.1182848006243944 ) ) ;
#41994=CARTESIAN_POINT ( 'NONE',  ( -29.37542415142715768, 1526.382868172864164, 200.9849896654584143 ) ) ;
#42004=CARTESIAN_POINT ( 'NONE',  ( -0.4992773797353766141, 1524.841055067849993, 174.1119671515087930 ) ) ;
#42012=EDGE_CURVE ( 'NONE', #68807, #48271, #35140, .T. ) ;
#42026=CARTESIAN_POINT ( 'NONE',  ( 0.000000000000000000, 1511.187213306747708, 209.1218459616979999 ) ) ;
#42043=LINE ( 'NONE', #43699, #17473 ) ;
#42075=ORIENTED_EDGE ( 'NONE', *, *, #15380, .F. ) ;
#42076=DIRECTION ( 'NONE',  ( 0.000000000000000000, 0.000000000000000000, 1.000000000000000000 ) ) ;
#42097=VERTEX_POINT ( 'NONE', #65331 ) ;
#42119=CARTESIAN_POINT ( 'NONE',  ( -21.53712143570538373, 1523.621879633028811, 234.3036048850999578 ) ) ;
#42122=DIRECTION ( 'NONE',  ( -0.8090169943749551118, 0.000000000000000000, -0.5877852522924625900 ) ) ;
#42124=VERTEX_POINT ( 'NONE', #64229 ) ;
#42148=LINE ( 'NONE', #103131, #69415 ) ;
#42186=FACE_OUTER_BOUND ( 'NONE', #29934, .T. ) ;
#42202=( BOUNDED_SURFACE ( )  B_SPLINE_SURFACE ( 3, 2, ( 
 ( #65844, #13190, #74793 ),
 ( #5366, #108936, #32226 ),
 ( #66405, #93223, #77544 ),
 ( #24892, #17595, #66952 ),
 ( #43394, #41177, #75351 ),
 ( #32768, #60198, #848 ) ),
 .UNSPECIFIED., .F., .F., .F. ) 
 B_SPLINE_SURFACE_WITH_KNOTS ( ( 4, 2, 4 ),
 ( 3, 3 ),
 ( 2.211772431870429045E-17, 0.001312027981647160809, 0.002624055963294299500 ),
 ( 0.000000000000000000, 1.000000000000000000 ),
 .UNSPECIFIED. ) 
 GEOMETRIC_REPRESENTATION_ITEM ( )  RATIONAL_B_SPLINE_SURFACE ( (
 ( 1.000000000000000000, 0.9376006582766006625, 1.000000000000000000),
 ( 1.000000000000000000, 0.9569320108033070316, 1.000000000000000000),
 ( 1.000000000000000000, 0.9725743441605053663, 1.000000000000000000),
 ( 1.000000000000000000, 0.9942095667149576377, 1.000000000000000000),
 ( 1.000000000000000000, 1.000043666449661917, 1.000000000000000000),
 ( 1.000000000000000000, 1.000000000000000000, 1.000000000000000000) ) ) 
 REPRESENTATION_ITEM ( '' )  SURFACE ( )  );
#42224=CARTESIAN_POINT ( 'NONE',  ( -19.53786426059057746, 1512.187213306747481, 181.5239794925695946 ) ) ;
#42228=ADVANCED_FACE ( 'NONE', ( #4839 ), #10645, .T. ) ;
#42241=CARTESIAN_POINT ( 'NONE',  ( -31.23437356469425907, 1512.187213306747481, 222.8968241038848248 ) ) ;
#42242=LINE ( 'NONE', #104353, #21663 ) ;
#42246=DIRECTION ( 'NONE',  ( -1.000000000000000000, 0.000000000000000000, 0.000000000000000000 ) ) ;
#42275=CARTESIAN_POINT ( 'NONE',  ( -18.51436573157397092, 1511.187213306747708, 181.1015051776554969 ) ) ;
#42278=CARTESIAN_POINT ( 'NONE',  ( -20.72500163405283047, 1525.697946996666815, 184.6549699785309144 ) ) ;
#42292=CARTESIAN_POINT ( 'NONE',  ( -33.93019615848961479, 1524.726013923371283, 197.6607374646001460 ) ) ;
#42315=MECHANICAL_DESIGN_GEOMETRIC_PRESENTATION_REPRESENTATION('',(#44087),#51268);
#42325=CARTESIAN_POINT ( 'NONE',  ( 1.775988990176029736, 1526.208281990539717, 240.5699127611650567 ) ) ;
#42328=DIRECTION ( 'NONE',  ( 1.000000000000000000, 0.000000000000000000, 0.000000000000000000 ) ) ;
#42335=CARTESIAN_POINT ( 'NONE',  ( 2.485536261606702269, 1523.919934424249959, 242.8055311927600144 ) ) ;
#42353=ORIENTED_EDGE ( 'NONE', *, *, #70651, .F. ) ;
#42395=EDGE_CURVE ( 'NONE', #47896, #37975, #31882, .T. ) ;
#42421=CARTESIAN_POINT ( 'NONE',  ( 31.95643112691247367, 1526.329757971584741, 216.6807372298920313 ) ) ;
#42430=CYLINDRICAL_SURFACE ( 'NONE', #98487, 23.69926344187880929 ) ;
#42432=AXIS2_PLACEMENT_3D ( 'NONE', #95706, #18972, #53168 ) ;
#42434=CARTESIAN_POINT ( 'NONE',  ( -22.08622291482314282, 1523.382868172864164, 233.8253038720786776 ) ) ;
#42444=VERTEX_POINT ( 'NONE', #74825 ) ;
#42461=EDGE_LOOP ( 'NONE', ( #49535, #67416, #3848, #41099, #5584, #106827, #22348, #113, #8574, #41277, #15849, #73971, #44431, #93153, #61971, #32343, #86394, #40917, #64951, #34024, #89028, #62335, #47949, #59318, #62116, #3399, #110239, #59389, #19064, #102619, #106923, #98669, #89128, #81879, #93226, #96480, #85235, #74875, #104064, #70199, #58351, #71523, #11903, #28165, #72588, #55047, #65867, #69849, #65233, #41645, #38335, #79800, #39050, #55896, #44449, #79415, #70386, #20407, #56065, #81838, #89041, #78647, #96892, #80211, #75288, #99867, #11046, #80159, #68404, #74723, #58198, #63759, #69442, #51011, #23590, #104676, #59313, #40054, #98726, #33368, #105834, #7790, #105140, #49015, #35337, #15547, #57758, #2812, #110805, #48688, #2472, #77842 ) ) ;
#42477=CARTESIAN_POINT ( 'NONE',  ( 20.79738390328720499, 1511.187213306747708, 181.2030061003470394 ) ) ;
#42494=CARTESIAN_POINT ( 'NONE',  ( -29.79881796581611297, 1526.748660780343471, 221.5803863269308636 ) ) ;
#42500=FACE_OUTER_BOUND ( 'NONE', #81606, .T. ) ;
#42512=CIRCLE ( 'NONE', #35403, 2.000000000000000444 ) ;
#42513=DIRECTION ( 'NONE',  ( -0.1070030146457423004, 0.000000000000000000, -0.9942586961433744763 ) ) ;
#42515=CARTESIAN_POINT ( 'NONE',  ( 2.599446155150029636, 1525.231909165033585, 241.5259142133259047 ) ) ;
#42516=VERTEX_POINT ( 'NONE', #93256 ) ;
#42536=EDGE_CURVE ( 'NONE', #74589, #20620, #24656, .T. ) ;
#42537=CARTESIAN_POINT ( 'NONE',  ( -30.37359097063415803, 1526.143142182216934, 201.3152257445480871 ) ) ;
#42542=CARTESIAN_POINT ( 'NONE',  ( 33.13357216314884823, 1523.313115944345100, 217.3564597502656568 ) ) ;
#42559=CARTESIAN_POINT ( 'NONE',  ( -2.596261494520225366, 1525.907212628473644, 177.4701144822246874 ) ) ;
#42573=CARTESIAN_POINT ( 'NONE',  ( 0.000000000000000000, 1523.382868172864164, 209.1218459616979999 ) ) ;
#42583=EDGE_LOOP ( 'NONE', ( #62191, #26721, #1042, #10531 ) ) ;
#42595=CARTESIAN_POINT ( 'NONE',  ( -29.67167576299870646, 1526.344110814219675, 216.9865736510277827 ) ) ;
#42597=CIRCLE ( 'NONE', #13966, 1.000000000000000888 ) ;
#42605=CARTESIAN_POINT ( 'NONE',  ( 31.92108011125344191, 1511.187213306747708, 197.2845127572061301 ) ) ;
#42607=VECTOR ( 'NONE', #19656, 1000.000000000000000 ) ;
#42614=TOROIDAL_SURFACE ( 'NONE', #46244, 2.000000000000000000, 1.000000000000000000 ) ;
#42636=CARTESIAN_POINT ( 'NONE',  ( 0.4151546846821903003, 1512.187213306747481, 244.9330574173806951 ) ) ;
#42640=VERTEX_POINT ( 'NONE', #33871 ) ;
#42650=CARTESIAN_POINT ( 'NONE',  ( 22.07680858347410435, 1523.847233649538339, 233.7985801730517323 ) ) ;
#42653=EDGE_CURVE ( 'NONE', #100587, #47989, #87479, .T. ) ;
#42665=CARTESIAN_POINT ( 'NONE',  ( -21.28823305372391772, 1525.253996226948175, 234.3566951577463158 ) ) ;
#42690=AXIS2_PLACEMENT_3D ( 'NONE', #66052, #15586, #40818 ) ;
#42694=AXIS2_PLACEMENT_3D ( 'NONE', #78758, #36204, #69833 ) ;
#42709=CARTESIAN_POINT ( 'NONE',  ( 21.83550407203919974, 1523.678648413191695, 234.9693198511250785 ) ) ;
#42711=CARTESIAN_POINT ( 'NONE',  ( 30.12521068615187048, 1524.538969332612623, 195.8585657628962906 ) ) ;
#42719=DIRECTION ( 'NONE',  ( 0.000000000000000000, -1.000000000000000000, 0.000000000000000000 ) ) ;
#42723=DIRECTION ( 'NONE',  ( 0.6709778558543766369, 0.000000000000000000, 0.7414773880254632576 ) ) ;
#42725=CARTESIAN_POINT ( 'NONE',  ( -29.99620953741480278, 1526.382868172863937, 219.7462484079463252 ) ) ;
#42728=CARTESIAN_POINT ( 'NONE',  ( 16.58908872130572121, 1524.412455883367329, 180.6440485805556193 ) ) ;
#42744=ORIENTED_EDGE ( 'NONE', *, *, #55075, .T. ) ;
#42747=CARTESIAN_POINT ( 'NONE',  ( 21.78049460968683348, 1524.843416604514687, 184.6507917665084335 ) ) ;
#42756=TOROIDAL_SURFACE ( 'NONE', #64271, 2.000000000000000000, 1.000000000000000000 ) ;
#42768=ORIENTED_EDGE ( 'NONE', *, *, #76478, .T. ) ;
#42771=CARTESIAN_POINT ( 'NONE',  ( -32.02808312589930040, 1512.187213306747481, 198.2787714533499752 ) ) ;
#42793=CARTESIAN_POINT ( 'NONE',  ( -34.68852446352951802, 1501.977400791986611, 199.9946320047955339 ) ) ;
#42803=CARTESIAN_POINT ( 'NONE',  ( 30.36939524941482205, 1525.506916460681623, 221.4200585932857166 ) ) ;
#42831=DIRECTION ( 'NONE',  ( -0.4090087482554316534, 0.000000000000000000, -0.9125304618753967700 ) ) ;
#42835=DIRECTION ( 'NONE',  ( -0.6709778558543678662, 0.000000000000000000, 0.7414773880254711402 ) ) ;
#42836=CARTESIAN_POINT ( 'NONE',  ( 20.71343476517534299, 1501.977400791986611, 238.3377464195763764 ) ) ;
#42844=DIRECTION ( 'NONE',  ( 0.9510565162951566398, 0.000000000000000000, 0.3090169943749382919 ) ) ;
#42845=CARTESIAN_POINT ( 'NONE',  ( 30.31404213106226919, 1524.330813522192102, 196.4516891724779271 ) ) ;
#42851=CIRCLE ( 'NONE', #69805, 0.9999999999999981126 ) ;
#42853=CARTESIAN_POINT ( 'NONE',  ( -29.99620953741502660, 1526.382868172863937, 198.4974435154502999 ) ) ;
#42859=ORIENTED_EDGE ( 'NONE', *, *, #23624, .T. ) ;
#42862=ORIENTED_EDGE ( 'NONE', *, *, #23926, .F. ) ;
#42878=CARTESIAN_POINT ( 'NONE',  ( 32.02808312589916540, 1501.977400791986611, 198.2787714533495489 ) ) ;
#42880=ORIENTED_EDGE ( 'NONE', *, *, #72805, .T. ) ;
#42887=CARTESIAN_POINT ( 'NONE',  ( 1.389373685237508260, 1526.382868173645647, 239.5386865367409825 ) ) ;
#42890=DIRECTION ( 'NONE',  ( 0.000000000000000000, 0.000000000000000000, 1.000000000000000000 ) ) ;
#42903=CARTESIAN_POINT ( 'NONE',  ( -21.80961449745526437, 1523.919934424249959, 183.3321337352031435 ) ) ;
#42908=ORIENTED_EDGE ( 'NONE', *, *, #89272, .F. ) ;
#42912=CIRCLE ( 'NONE', #37549, 1.000000000000000888 ) ;
#42933=ORIENTED_EDGE ( 'NONE', *, *, #6036, .F. ) ;
#42937=ORIENTED_EDGE ( 'NONE', *, *, #55066, .F. ) ;
#42958=CARTESIAN_POINT ( 'NONE',  ( 2.444956619880277682, 1524.972613296788722, 175.9713629724293469 ) ) ;
#42972=ORIENTED_EDGE ( 'NONE', *, *, #70910, .F. ) ;
#42980=DIRECTION ( 'NONE',  ( -0.9942586961433749204, 0.000000000000000000, 0.1070030146457375819 ) ) ;
#42986=EDGE_CURVE ( 'NONE', #58330, #77302, #80033, .T. ) ;
#42994=VERTEX_POINT ( 'NONE', #37479 ) ;
#42996=FACE_OUTER_BOUND ( 'NONE', #37905, .T. ) ;
#42999=CARTESIAN_POINT ( 'NONE',  ( 31.32995031131189378, 1523.678648413191695, 196.3423562208913324 ) ) ;
#43012=CARTESIAN_POINT ( 'NONE',  ( 32.86802468386292730, 1523.382868172864164, 217.2040256693915410 ) ) ;
#43014=ORIENTED_EDGE ( 'NONE', *, *, #85913, .F. ) ;
#43030=CARTESIAN_POINT ( 'NONE',  ( 32.38845791999500534, 1512.187213306747481, 216.1254071228445639 ) ) ;
#43041=CARTESIAN_POINT ( 'NONE',  ( -2.691689582131152836, 1524.775785348137561, 176.4304728337446306 ) ) ;
#43056=CARTESIAN_POINT ( 'NONE',  ( 18.86688640473602874, 1512.187213306747481, 237.4611898188519774 ) ) ;
#43086=CARTESIAN_POINT ( 'NONE',  ( -32.23107245337178739, 1523.542365884048195, 201.4053004075473439 ) ) ;
#43102=DIRECTION ( 'NONE',  ( 0.000000000000000000, 0.000000000000000000, 1.000000000000000000 ) ) ;
#43104=TOROIDAL_SURFACE ( 'NONE', #282, 30.13701971169416538, 3.000000000000000000 ) ;
#43137=CARTESIAN_POINT ( 'NONE',  ( -20.71343476517093052, 1522.906561336852974, 238.3377464195795596 ) ) ;
#43160=COLOUR_RGB ( '', 0.31764706, 0.68627451, 0.89019608) ;
#43165=CARTESIAN_POINT ( 'NONE',  ( -17.84338787571961049, 1501.977400791986611, 180.3600277896300383 ) ) ;
#43179=EDGE_CURVE ( 'NONE', #80823, #44004, #81121, .T. ) ;
#43187=VERTEX_POINT ( 'NONE', #64352 ) ;
#43194=DIRECTION ( 'NONE',  ( 0.000000000000000000, 0.000000000000000000, 1.000000000000000000 ) ) ;
#43202=( BOUNDED_SURFACE ( )  B_SPLINE_SURFACE ( 3, 2, ( 
 ( #47115, #38690, #66550 ),
 ( #72865, #46577, #21861 ),
 ( #106458, #23938, #72328 ),
 ( #67094, #56060, #47661 ),
 ( #58133, #74941, #7166 ),
 ( #49734, #5090, #81241 ),
 ( #55521, #58682, #39243 ),
 ( #4020, #38147, #30289 ),
 ( #21317, #100652, #92816 ),
 ( #7707, #12391, #90187 ) ),
 .UNSPECIFIED., .F., .F., .F. ) 
 B_SPLINE_SURFACE_WITH_KNOTS ( ( 4, 2, 2, 2, 4 ),
 ( 3, 3 ),
 ( 1.570796326794896558, 1.963495408493620697, 2.356194490192344837, 2.748893571891068976, 3.141592653589793116 ),
 ( 0.000000000000000000, 1.000000000000000000 ),
 .UNSPECIFIED. ) 
 GEOMETRIC_REPRESENTATION_ITEM ( )  RATIONAL_B_SPLINE_SURFACE ( (
 ( 1.000000000000000000, 0.7071067811865872077, 1.000000000000000000),
 ( 1.000000000000000000, 0.7166207884826032437, 1.000000000000000000),
 ( 1.000000000000000000, 0.7259222650901892004, 1.000000000000000000),
 ( 1.000000000000000000, 0.7428408967935505869, 1.000000000000000000),
 ( 1.000000000000000000, 0.7504512394523125129, 1.000000000000000000),
 ( 1.000000000000000000, 0.7630177051951873013, 1.000000000000000000),
 ( 1.000000000000000000, 0.7679730451971447103, 1.000000000000000000),
 ( 1.000000000000000000, 0.7746454561799092087, 1.000000000000000000),
 ( 1.000000000000000000, 0.7763684247033758590, 1.000000000000000000),
 ( 1.000000000000000000, 0.7763623250684337229, 1.000000000000000000) ) ) 
 REPRESENTATION_ITEM ( '' )  SURFACE ( )  );
#43207=AXIS2_PLACEMENT_3D ( 'NONE', #43542, #77687, #62019 ) ;
#43230=CARTESIAN_POINT ( 'NONE',  ( -18.15646965371467658, 1522.906363951597314, 180.0767137688672221 ) ) ;
#43241=CARTESIAN_POINT ( 'NONE',  ( -1.336801414592336812, 1526.382868172864164, 239.5691425648093116 ) ) ;
#43253=B_SPLINE_CURVE_WITH_KNOTS ( 'NONE', 3,
 ( #69161, #103265, #52911, #60771 ),
 .UNSPECIFIED., .F., .F.,
 ( 4, 4 ),
 ( 0.000000000000000000, 0.0002220129587134788318 ),
 .UNSPECIFIED. ) ;
#43255=CARTESIAN_POINT ( 'NONE',  ( -16.89233068642501934, 1526.349684470114653, 183.3465479968500631 ) ) ;
#43261=VERTEX_POINT ( 'NONE', #69316 ) ;
#43264=ADVANCED_FACE ( 'NONE', ( #43549 ), #26732, .T. ) ;
#43266=CARTESIAN_POINT ( 'NONE',  ( -33.23571934791658578, 1511.187213306747708, 219.4842663281467026 ) ) ;
#43272=CARTESIAN_POINT ( 'NONE',  ( -20.12564951288307213, 1511.187213306747708, 180.7149624981946658 ) ) ;
#43282=CIRCLE ( 'NONE', #84348, 1.000000000000000888 ) ;
#43283=CARTESIAN_POINT ( 'NONE',  ( 16.66231036550703593, 1523.604703353109699, 180.4882076302513099 ) ) ;
#43284=EDGE_CURVE ( 'NONE', #2813, #35962, #30040, .T. ) ;
#43286=LINE ( 'NONE', #77976, #26505 ) ;
#43289=CARTESIAN_POINT ( 'NONE',  ( 17.44952998132189848, 1525.163457223744217, 181.0033690456834847 ) ) ;
#43310=ORIENTED_EDGE ( 'NONE', *, *, #14876, .T. ) ;
#43319=EDGE_CURVE ( 'NONE', #85956, #92642, #89116, .T. ) ;
#43331=ORIENTED_EDGE ( 'NONE', *, *, #81579, .T. ) ;
#43352=ORIENTED_EDGE ( 'NONE', *, *, #78980, .T. ) ;
#43358=LINE ( 'NONE', #18669, #25263 ) ;
#43360=ADVANCED_FACE ( 'NONE', ( #92015 ), #60647, .T. ) ;
#43394=CARTESIAN_POINT ( 'NONE',  ( 19.02270174365926536, 1526.382868172864164, 185.3889643599916610 ) ) ;
#43404=CYLINDRICAL_SURFACE ( 'NONE', #92842, 3.999999999999999112 ) ;
#43405=DIRECTION ( 'NONE',  ( -0.8642610224695990162, 0.000000000000000000, 0.5030436214085248769 ) ) ;
#43408=LINE ( 'NONE', #77559, #32422 ) ;
#43419=ORIENTED_EDGE ( 'NONE', *, *, #1710, .T. ) ;
#43427=CARTESIAN_POINT ( 'NONE',  ( -0.7800921441517141286, 1526.382868172863937, 241.4567505818336031 ) ) ;
#43440=CARTESIAN_POINT ( 'NONE',  ( 20.12564951288265647, 1512.187213306747481, 180.7149624981944100 ) ) ;
#43449=EDGE_CURVE ( 'NONE', #71455, #10257, #38174, .T. ) ;
#43457=CARTESIAN_POINT ( 'NONE',  ( -24.25895011704391990, 1512.187213306747481, 247.1119212070238405 ) ) ;
#43461=EDGE_CURVE ( 'NONE', #81049, #13345, #42597, .T. ) ;
#43464=B_SPLINE_CURVE_WITH_KNOTS ( 'NONE', 3,
 ( #99708, #108680, #98069, #39827 ),
 .UNSPECIFIED., .F., .F.,
 ( 4, 4 ),
 ( 0.000000000000000000, 0.0002960034161023838636 ),
 .UNSPECIFIED. ) ;
#43482=EDGE_CURVE ( 'NONE', #29531, #83952, #2957, .T. ) ;
#43491=CARTESIAN_POINT ( 'NONE',  ( 2.470168521978398424, 1523.382868172864164, 242.8787258963054683 ) ) ;
#43516=CARTESIAN_POINT ( 'NONE',  ( -31.47409394596237320, 1526.278758871497757, 199.6577681796610761 ) ) ;
#43542=CARTESIAN_POINT ( 'NONE',  ( -20.12564951288246107, 1512.187213306747481, 237.5287294252017603 ) ) ;
#43549=FACE_OUTER_BOUND ( 'NONE', #30098, .T. ) ;
#43591=CARTESIAN_POINT ( 'NONE',  ( -3.351183042480982976, 1524.075000532256581, 176.2264671304546368 ) ) ;
#43597=VERTEX_POINT ( 'NONE', #80186 ) ;
#43605=CARTESIAN_POINT ( 'NONE',  ( -30.51231035492510557, 1526.382868172863937, 218.1578534183722979 ) ) ;
#43631=CARTESIAN_POINT ( 'NONE',  ( 31.32995031131189378, 1523.678648413191922, 196.3423562208913324 ) ) ;
#43644=CARTESIAN_POINT ( 'NONE',  ( -29.30029655192939586, 1525.907212628473872, 196.8717316207790589 ) ) ;
#43657=AXIS2_PLACEMENT_3D ( 'NONE', #71820, #37065, #71260 ) ;
#43687=EDGE_LOOP ( 'NONE', ( #11977, #48517, #58163, #44579 ) ) ;
#43690=VERTEX_POINT ( 'NONE', #76189 ) ;
#43691=DIRECTION ( 'NONE',  ( -0.5877852522924629231, 0.000000000000000000, 0.8090169943749548898 ) ) ;
#43697=FACE_OUTER_BOUND ( 'NONE', #109026, .T. ) ;
#43699=CARTESIAN_POINT ( 'NONE',  ( 33.28034951413933129, 1501.977400791986611, 217.4407153818819722 ) ) ;
#43710=ORIENTED_EDGE ( 'NONE', *, *, #26107, .F. ) ;
#43726=VERTEX_POINT ( 'NONE', #50454 ) ;
#43730=ORIENTED_EDGE ( 'NONE', *, *, #17890, .F. ) ;
#43744=CARTESIAN_POINT ( 'NONE',  ( -32.86802468386298415, 1512.187213306747481, 201.0396662540046577 ) ) ;
#43752=ORIENTED_EDGE ( 'NONE', *, *, #24716, .T. ) ;
#43754=CARTESIAN_POINT ( 'NONE',  ( 17.17241001986506888, 1518.913060387330006, 238.6251415217915337 ) ) ;
#43771=CARTESIAN_POINT ( 'NONE',  ( -17.44374831407532866, 1524.130440953581001, 180.7216696960686591 ) ) ;
#43780=DIRECTION ( 'NONE',  ( 0.000000000000000000, 0.000000000000000000, -1.000000000000000000 ) ) ;
#43783=CARTESIAN_POINT ( 'NONE',  ( 31.23437356469435144, 1512.187213306747481, 196.3468678195113739 ) ) ;
#43797=CARTESIAN_POINT ( 'NONE',  ( -16.73628186595857059, 1526.382868172863937, 184.0591879540917546 ) ) ;
#43804=DIRECTION ( 'NONE',  ( 0.000000000000000000, 1.000000000000000000, 0.000000000000000000 ) ) ;
#43809=VECTOR ( 'NONE', #11780, 1000.000000000000227 ) ;
#43813=CARTESIAN_POINT ( 'NONE',  ( 30.31052258194586102, 1523.604703353109699, 195.7506062427368079 ) ) ;
#43833=CARTESIAN_POINT ( 'NONE',  ( 17.19739463999635021, 1525.960063244516959, 181.9833109756549163 ) ) ;
#43839=DIRECTION ( 'NONE',  ( 0.000000000000000000, 0.000000000000000000, 1.000000000000000000 ) ) ;
#43845=FACE_OUTER_BOUND ( 'NONE', #106508, .T. ) ;
#43853=ORIENTED_EDGE ( 'NONE', *, *, #95934, .F. ) ;
#43865=EDGE_CURVE ( 'NONE', #42097, #32377, #53210, .T. ) ;
#43885=VERTEX_POINT ( 'NONE', #8413 ) ;
#43899=LINE ( 'NONE', #1350, #8745 ) ;
#43901=CARTESIAN_POINT ( 'NONE',  ( 21.13130013988266853, 1524.397344074319108, 180.8335768739904381 ) ) ;
#43907=DIRECTION ( 'NONE',  ( -0.9948834766775040972, 0.000000000000000000, 0.1010290445074205484 ) ) ;
#43911=CARTESIAN_POINT ( 'NONE',  ( 30.01483979338928165, 1525.231887713385959, 221.6074839523207345 ) ) ;
#43937=DIRECTION ( 'NONE',  ( 0.000000000000000000, 0.000000000000000000, 1.000000000000000000 ) ) ;
#43941=CARTESIAN_POINT ( 'NONE',  ( -21.55808780550650283, 1523.844782250843537, 183.9826089808311735 ) ) ;
#43944=EDGE_LOOP ( 'NONE', ( #76486, #99336, #10506 ) ) ;
#43947=ADVANCED_FACE ( 'NONE', ( #92295 ), #76646, .T. ) ;
#43956=FACE_OUTER_BOUND ( 'NONE', #66347, .T. ) ;
#43972=ADVANCED_FACE ( 'NONE', ( #44125 ), #101785, .T. ) ;
#43977=DIRECTION ( 'NONE',  ( 0.000000000000000000, 1.000000000000000000, 0.000000000000000000 ) ) ;
#43985=CIRCLE ( 'NONE', #85121, 33.13701971169416538 ) ;
#43992=CARTESIAN_POINT ( 'NONE',  ( -32.16567119605149827, 1524.523992613102564, 202.1429910727728725 ) ) ;
#44004=VERTEX_POINT ( 'NONE', #60939 ) ;
#44011=AXIS2_PLACEMENT_3D ( 'NONE', #75472, #57569, #40189 ) ;
#44014=CIRCLE ( 'NONE', #58317, 1.000000000000000000 ) ;
#44040=ORIENTED_EDGE ( 'NONE', *, *, #75729, .F. ) ;
#44058=ORIENTED_EDGE ( 'NONE', *, *, #82080, .T. ) ;
#44060=B_SPLINE_CURVE_WITH_KNOTS ( 'NONE', 3,
 ( #69008, #43241, #86880, #103685, #44914, #94729 ),
 .UNSPECIFIED., .F., .F.,
 ( 4, 2, 4 ),
 ( -1.285435071114489149E-05, 0.001079388306740552582, 0.002171630964192249828 ),
 .UNSPECIFIED. ) ;
#44061=EDGE_CURVE ( 'NONE', #88474, #63875, #39063, .T. ) ;
#44065=CARTESIAN_POINT ( 'NONE',  ( -34.31402925621634381, 1524.244163922423695, 200.2096061136544165 ) ) ;
#44071=CARTESIAN_POINT ( 'NONE',  ( 76.99707197885321364, 1524.382868172863937, 398.8876973329328735 ) ) ;
#44083=CARTESIAN_POINT ( 'NONE',  ( 33.28034951413933129, 1522.382868172863937, 217.4407153818819722 ) ) ;
#44087=STYLED_ITEM ( 'NONE', ( #19160 ), #8479 ) ;
#44099=ORIENTED_EDGE ( 'NONE', *, *, #104518, .F. ) ;
#44101=CARTESIAN_POINT ( 'NONE',  ( 29.82178186784435425, 1526.306647125543122, 201.3257788173809786 ) ) ;
#44120=FACE_OUTER_BOUND ( 'NONE', #102301, .T. ) ;
#44125=FACE_OUTER_BOUND ( 'NONE', #3365, .T. ) ;
#44130=CARTESIAN_POINT ( 'NONE',  ( 31.23437356469435144, 1511.187213306747708, 195.3468678195113739 ) ) ;
#44137=ORIENTED_EDGE ( 'NONE', *, *, #33831, .T. ) ;
#44154=VERTEX_POINT ( 'NONE', #45797 ) ;
#44164=CARTESIAN_POINT ( 'NONE',  ( -22.08622291482314282, 1523.456872492435195, 233.8253038720786776 ) ) ;
#44166=CIRCLE ( 'NONE', #79965, 1.000000000000000888 ) ;
#44193=CARTESIAN_POINT ( 'NONE',  ( 2.214867471995963566, 1525.730671948510917, 241.5483233331381427 ) ) ;
#44195=DIRECTION ( 'NONE',  ( 0.000000000000000000, 1.000000000000000000, 0.000000000000000000 ) ) ;
#44210=CARTESIAN_POINT ( 'NONE',  ( -32.66476241579324125, 1526.382868172863937, 199.1278258474841891 ) ) ;
#44212=FACE_OUTER_BOUND ( 'NONE', #87766, .T. ) ;
#44213=CARTESIAN_POINT ( 'NONE',  ( -1.488474718485068182, 1526.348417187222367, 239.9133697138384775 ) ) ;
#44227=ORIENTED_EDGE ( 'NONE', *, *, #65051, .T. ) ;
#44231=CARTESIAN_POINT ( 'NONE',  ( -32.36539537780667786, 1523.843271061948144, 216.1095012219382454 ) ) ;
#44248=ORIENTED_EDGE ( 'NONE', *, *, #26107, .T. ) ;
#44250=CARTESIAN_POINT ( 'NONE',  ( -0.4151546846821903003, 1512.187213306747481, 175.3106345060153046 ) ) ;
#44259=DIRECTION ( 'NONE',  ( 5.312590645178966993E-15, 0.000000000000000000, 1.000000000000000000 ) ) ;
#44261=CARTESIAN_POINT ( 'NONE',  ( 32.35345263957275108, 1524.872178180562969, 201.1945832501413634 ) ) ;
#44269=DIRECTION ( 'NONE',  ( -0.000000000000000000, -1.000000000000000000, -0.000000000000000000 ) ) ;
#44292=ORIENTED_EDGE ( 'NONE', *, *, #108894, .F. ) ;
#44295=FACE_OUTER_BOUND ( 'NONE', #93979, .T. ) ;
#44297=ORIENTED_EDGE ( 'NONE', *, *, #87963, .T. ) ;
#44309=EDGE_LOOP ( 'NONE', ( #61847, #81063, #52305, #73759, #25608, #76225, #31136, #19027, #72141, #3681, #27673, #38883, #30100, #31442, #66796, #21577, #78989, #74053, #82243, #101700, #10116, #55124, #97602, #95550, #82925, #17655, #10409, #100125, #74874, #41784, #36848, #86784, #86679, #5210, #87196, #50894, #90912, #100526, #22609, #67417 ) ) ;
#44318=CARTESIAN_POINT ( 'NONE',  ( -31.81407709660762606, 1522.862737210649811, 221.9534378623334874 ) ) ;
#44336=CARTESIAN_POINT ( 'NONE',  ( -20.70484064406351621, 1525.907212628473644, 233.2025904124107569 ) ) ;
#44348=DIRECTION ( 'NONE',  ( 0.7414773880254711402, -0.000000000000000000, 0.6709778558543678662 ) ) ;
#44367=EDGE_CURVE ( 'NONE', #54639, #108510, #100566, .T. ) ;
#44370=CARTESIAN_POINT ( 'NONE',  ( 32.28466283162156714, 1511.187213306747708, 219.1752493337713190 ) ) ;
#44376=CARTESIAN_POINT ( 'NONE',  ( 31.34137657934019927, 1523.382868172864164, 221.9025654077410081 ) ) ;
#44377=FACE_OUTER_BOUND ( 'NONE', #14894, .T. ) ;
#44386=VECTOR ( 'NONE', #14029, 1000.000000000000000 ) ;
#44415=VERTEX_POINT ( 'NONE', #108986 ) ;
#44417=CARTESIAN_POINT ( 'NONE',  ( 21.14964295068612898, 1525.231887713385959, 184.4343113153503566 ) ) ;
#44431=ORIENTED_EDGE ( 'NONE', *, *, #36996, .T. ) ;
#44436=EDGE_LOOP ( 'NONE', ( #57053, #72157, #59959, #57206 ) ) ;
#44449=ORIENTED_EDGE ( 'NONE', *, *, #106519, .T. ) ;
#44458=CARTESIAN_POINT ( 'NONE',  ( -2.372478608332516892, 1522.862737210649811, 174.8996806668726549 ) ) ;
#44461=CARTESIAN_POINT ( 'NONE',  ( 22.41686883764370464, 1524.667648926078527, 181.9773018742387194 ) ) ;
#44471=CARTESIAN_POINT ( 'NONE',  ( 30.77244971921734873, 1524.972613296803956, 221.6912005025092753 ) ) ;
#44496=DIRECTION ( 'NONE',  ( -0.000000000000000000, 1.000000000000000000, -0.000000000000000000 ) ) ;
#44499=CARTESIAN_POINT ( 'NONE',  ( -21.55489959617492346, 1524.059547553519451, 184.0356378790828273 ) ) ;
#44507=CARTESIAN_POINT ( 'NONE',  ( -31.02592223166987395, 1526.278758871497075, 198.2784374727513352 ) ) ;
#44522=CARTESIAN_POINT ( 'NONE',  ( -22.08622291487980149, 1523.456924617336199, 233.8253038720280301 ) ) ;
#44529=AXIS2_PLACEMENT_3D ( 'NONE', #66308, #90358, #64649 ) ;
#44545=CARTESIAN_POINT ( 'NONE',  ( -32.35368859299580180, 1524.871836253796118, 201.1945538962762896 ) ) ;
#44547=DIRECTION ( 'NONE',  ( 0.6665120492724535550, 0.000000000000000000, -0.7454942576402816545 ) ) ;
#44560=CIRCLE ( 'NONE', #51668, 2.000000000000007550 ) ;
#44574=EDGE_CURVE ( 'NONE', #15990, #47552, #73068, .T. ) ;
#44579=ORIENTED_EDGE ( 'NONE', *, *, #6036, .T. ) ;
#44589=CARTESIAN_POINT ( 'NONE',  ( -29.95987888842740787, 1525.317359687841190, 221.5595086622937799 ) ) ;
#44604=EDGE_CURVE ( 'NONE', #92713, #100110, #1531, .T. ) ;
#44606=CARTESIAN_POINT ( 'NONE',  ( -21.84020450222076448, 1501.977400791986611, 183.2638850454220858 ) ) ;
#44655=VECTOR ( 'NONE', #23711, 1000.000000000000114 ) ;
#44661=CARTESIAN_POINT ( 'NONE',  ( -31.81407709660787830, 1522.862737210649811, 196.2902540610632229 ) ) ;
#44684=DIRECTION ( 'NONE',  ( -0.9786619618251657382, 0.000000000000000000, 0.2054769195713184449 ) ) ;
#44701=CARTESIAN_POINT ( 'NONE',  ( -2.472529913803022783, 1523.678648413191695, 242.8674788698241400 ) ) ;
#44706=CARTESIAN_POINT ( 'NONE',  ( -3.350338079455627671, 1523.604703353109926, 176.1628856388066708 ) ) ;
#44755=CARTESIAN_POINT ( 'NONE',  ( -21.05711716160297797, 1526.748660780343471, 233.6123052680180194 ) ) ;
#44756=VERTEX_POINT ( 'NONE', #74713 ) ;
#44777=TOROIDAL_SURFACE ( 'NONE', #107343, 2.000000000000000000, 1.000000000000000000 ) ;
#44784=DIRECTION ( 'NONE',  ( 0.000000000000000000, 1.000000000000000000, 0.000000000000000000 ) ) ;
#44791=CARTESIAN_POINT ( 'NONE',  ( -32.32092748916725355, 1524.075132568164918, 216.0999031672498063 ) ) ;
#44792=ORIENTED_EDGE ( 'NONE', *, *, #15827, .T. ) ;
#44798=EDGE_CURVE ( 'NONE', #62492, #67163, #99893, .T. ) ;
#44803=DIRECTION ( 'NONE',  ( 0.000000000000000000, 1.000000000000000000, 0.000000000000000000 ) ) ;
#44818=EDGE_CURVE ( 'NONE', #72801, #75901, #4727, .T. ) ;
#44827=CARTESIAN_POINT ( 'NONE',  ( -29.30029655192934257, 1525.907212628473644, 221.3719603026177367 ) ) ;
#44863=VECTOR ( 'NONE', #41823, 1000.000000000000000 ) ;
#44865=EDGE_CURVE ( 'NONE', #63875, #32555, #75804, .T. ) ;
#44877=ORIENTED_EDGE ( 'NONE', *, *, #78189, .T. ) ;
#44894=ADVANCED_FACE ( 'NONE', ( #15855 ), #16954, .T. ) ;
#44899=CARTESIAN_POINT ( 'NONE',  ( -20.88378052025218068, 1525.556089352309073, 233.6619250012938380 ) ) ;
#44907=CIRCLE ( 'NONE', #73512, 1.000000000000000888 ) ;
#44914=CARTESIAN_POINT ( 'NONE',  ( -1.909779004914694767, 1526.107876515966382, 240.8769758466254132 ) ) ;
#44927=CARTESIAN_POINT ( 'NONE',  ( 32.38845791999501245, 1523.382868172864164, 216.1254071228445639 ) ) ;
#44929=CARTESIAN_POINT ( 'NONE',  ( -17.04521562810680280, 1526.211523310372513, 182.6481121783497770 ) ) ;
#44941=CARTESIAN_POINT ( 'NONE',  ( -30.77244971921803085, 1524.972613296804866, 196.5524914208872644 ) ) ;
#44975=ORIENTED_EDGE ( 'NONE', *, *, #80239, .F. ) ;
#44978=CARTESIAN_POINT ( 'NONE',  ( 21.83550407203902921, 1523.678648413191468, 183.2743720722706939 ) ) ;
#44980=DIRECTION ( 'NONE',  ( 0.000000000000000000, 0.000000000000000000, 1.000000000000000000 ) ) ;
#44995=DIRECTION ( 'NONE',  ( 2.081668171172166620E-14, 0.000000000000000000, 1.000000000000000000 ) ) ;
#45012=CARTESIAN_POINT ( 'NONE',  ( 20.20959865099471031, 1512.187213306747481, 182.0120230947219966 ) ) ;
#45013=ORIENTED_EDGE ( 'NONE', *, *, #24212, .F. ) ;
#45018=ORIENTED_EDGE ( 'NONE', *, *, #100730, .F. ) ;
#45034=CARTESIAN_POINT ( 'NONE',  ( -2.485536755124557740, 1523.919943579690425, 242.8055288421958267 ) ) ;
#45039=EDGE_CURVE ( 'NONE', #72142, #49931, #90655, .T. ) ;
#45040=CARTESIAN_POINT ( 'NONE',  ( 30.51921334599647651, 1524.059663615500540, 221.8697286789197278 ) ) ;
#45062=AXIS2_PLACEMENT_3D ( 'NONE', #62834, #46000, #3451 ) ;
#45063=CARTESIAN_POINT ( 'NONE',  ( -20.70484064406366187, 1525.907212628473644, 233.2025904124108706 ) ) ;
#45077=CARTESIAN_POINT ( 'NONE',  ( -31.55762699681141115, 1523.390106123591067, 196.3178534513334341 ) ) ;
#45080=CIRCLE ( 'NONE', #59371, 0.9999999999999927836 ) ;
#45086=VECTOR ( 'NONE', #25076, 1000.000000000000000 ) ;
#45096=DIRECTION ( 'NONE',  ( 0.5877852522924685852, 0.000000000000000000, -0.8090169943749507819 ) ) ;
#45103=CARTESIAN_POINT ( 'NONE',  ( -31.23437356469455040, 1512.187213306747481, 195.3468678195118287 ) ) ;
#45107=ORIENTED_EDGE ( 'NONE', *, *, #62600, .F. ) ;
#45108=ORIENTED_EDGE ( 'NONE', *, *, #38900, .F. ) ;
#45109=DIRECTION ( 'NONE',  ( 0.000000000000000000, 1.000000000000000000, 0.000000000000000000 ) ) ;
#45114=CARTESIAN_POINT ( 'NONE',  ( -31.54872587855235722, 1525.317359687841190, 201.5741514857012930 ) ) ;
#45116=CYLINDRICAL_SURFACE ( 'NONE', #69868, 1.999999999999995337 ) ;
#45130=CARTESIAN_POINT ( 'NONE',  ( 1.491506560153233130, 1512.187213306747481, 175.5704429466618421 ) ) ;
#45131=VERTEX_POINT ( 'NONE', #27062 ) ;
#45134=ADVANCED_FACE ( 'NONE', ( #61248 ), #16662, .F. ) ;
#45138=ADVANCED_FACE ( 'NONE', ( #100166 ), #82264, .T. ) ;
#45147=CARTESIAN_POINT ( 'NONE',  ( 22.08622291482331335, 1518.913060387330006, 184.4183880513174927 ) ) ;
#45182=CARTESIAN_POINT ( 'NONE',  ( -32.40058737600818972, 1524.130440953581001, 201.3079925683071281 ) ) ;
#45189=CARTESIAN_POINT ( 'NONE',  ( 18.69816095120750532, 1522.382868172863937, 183.3860352823955679 ) ) ;
#45191=CARTESIAN_POINT ( 'NONE',  ( 0.000000000000000000, 1523.409940573003951, 209.1218459616979999 ) ) ;
#45198=CARTESIAN_POINT ( 'NONE',  ( -2.599451791485461349, 1525.231887713385959, 241.5259292574780545 ) ) ;
#45200=CARTESIAN_POINT ( 'NONE',  ( 28.54794148642324103, 1526.382868172864164, 219.8054320332928171 ) ) ;
#45214=EDGE_CURVE ( 'NONE', #79230, #12203, #48124, .T. ) ;
#45220=CARTESIAN_POINT ( 'NONE',  ( 22.69876404240077505, 1501.977400791986611, 181.3483716558180276 ) ) ;
#45253=CARTESIAN_POINT ( 'NONE',  ( -0.4151546846821903003, 1512.187213306747481, 244.9330574173806951 ) ) ;
#45276=ORIENTED_EDGE ( 'NONE', *, *, #15968, .F. ) ;
#45284=CARTESIAN_POINT ( 'NONE',  ( -34.18677586421173231, 1522.382868172863937, 219.7932833225216882 ) ) ;
#45295=CYLINDRICAL_SURFACE ( 'NONE', #97287, 2.000000000000003997 ) ;
#45327=DIRECTION ( 'NONE',  ( -0.7414773880254760252, -0.000000000000000000, -0.6709778558543624261 ) ) ;
#45330=CARTESIAN_POINT ( 'NONE',  ( -1.338895077072838058, 1526.382868172864164, 239.5739613961735586 ) ) ;
#45348=DIRECTION ( 'NONE',  ( 0.000000000000000000, 0.000000000000000000, 1.000000000000000000 ) ) ;
#45349=ORIENTED_EDGE ( 'NONE', *, *, #36650, .T. ) ;
#45354=CARTESIAN_POINT ( 'NONE',  ( -16.66936639845610557, 1523.456872492435195, 237.7608804993221838 ) ) ;
#45364=DIRECTION ( 'NONE',  ( 0.000000000000000000, 0.000000000000000000, -1.000000000000000000 ) ) ;
#45369=ORIENTED_EDGE ( 'NONE', *, *, #90605, .F. ) ;
#45375=CARTESIAN_POINT ( 'NONE',  ( 31.87595007833802896, 1525.042412244735260, 202.1059224821480882 ) ) ;
#45377=EDGE_CURVE ( 'NONE', #52269, #39456, #110688, .T. ) ;
#45387=EDGE_CURVE ( 'NONE', #76248, #39549, #65983, .T. ) ;
#45402=DIRECTION ( 'NONE',  ( -0.8672669759446595128, 0.000000000000000000, 0.4978433412588795237 ) ) ;
#45427=CARTESIAN_POINT ( 'NONE',  ( 29.37019419317383750, 1526.382868172864164, 200.9844875749016921 ) ) ;
#45451=CARTESIAN_POINT ( 'NONE',  ( -18.00465857450906171, 1523.390106123591067, 180.2140906788921768 ) ) ;
#45458=EDGE_CURVE ( 'NONE', #1895, #64042, #24791, .T. ) ;
#45459=CARTESIAN_POINT ( 'NONE',  ( 0.4151546846821903003, 1512.187213306747481, 175.3106345060153046 ) ) ;
#45461=CARTESIAN_POINT ( 'NONE',  ( 31.81407709660777527, 1522.382868172863937, 221.9534378623329758 ) ) ;
#45464=ADVANCED_FACE ( 'NONE', ( #110483 ), #3517, .T. ) ;
#45465=DIRECTION ( 'NONE',  ( 0.000000000000000000, 0.000000000000000000, -1.000000000000000000 ) ) ;
#45497=CARTESIAN_POINT ( 'NONE',  ( -29.67375891016008893, 1525.697947650397282, 196.9718794197341651 ) ) ;
#45506=CARTESIAN_POINT ( 'NONE',  ( -31.22294729666638347, 1523.678648413191695, 195.3480975247483968 ) ) ;
#45511=DIRECTION ( 'NONE',  ( -0.000000000000000000, -1.000000000000000000, -0.000000000000000000 ) ) ;
#45527=CARTESIAN_POINT ( 'NONE',  ( 22.75273496409597485, 1518.913060387330006, 234.5707981297185825 ) ) ;
#45537=ORIENTED_EDGE ( 'NONE', *, *, #5587, .T. ) ;
#45586=CARTESIAN_POINT ( 'NONE',  ( -2.485500793217951809, 1524.600389084707103, 242.5122197736536975 ) ) ;
#45594=CARTESIAN_POINT ( 'NONE',  ( -17.22627300064457145, 1525.856064936156827, 236.4663892367293556 ) ) ;
#45596=CARTESIAN_POINT ( 'NONE',  ( 29.67167576299816645, 1526.344110814219903, 216.9865736510273280 ) ) ;
#45614=CARTESIAN_POINT ( 'NONE',  ( 20.12564951288265291, 1511.187213306747708, 180.7149624981943816 ) ) ;
#45639=AXIS2_PLACEMENT_3D ( 'NONE', #98, #35326, #70616 ) ;
#45659=EDGE_CURVE ( 'NONE', #94817, #44756, #4950, .T. ) ;
#45661=CARTESIAN_POINT ( 'NONE',  ( -3.347801439296148818, 1523.456872492435195, 242.0893193391992497 ) ) ;
#45671=CARTESIAN_POINT ( 'NONE',  ( -31.80537271888373496, 1525.137881624895499, 202.0924996609166158 ) ) ;
#45680=DIRECTION ( 'NONE',  ( 0.000000000000000000, 0.000000000000000000, -1.000000000000000000 ) ) ;
#45684=LINE ( 'NONE', #37259, #25069 ) ;
#45691=CIRCLE ( 'NONE', #17000, 2.000000000000001776 ) ;
#45709=CARTESIAN_POINT ( 'NONE',  ( -30.15968401513964281, 1524.412455883367329, 222.4100463060516972 ) ) ;
#45744=CARTESIAN_POINT ( 'NONE',  ( 17.84338787571921969, 1523.382868172864164, 180.3600277896298110 ) ) ;
#45749=DIRECTION ( 'NONE',  ( 0.000000000000000000, 0.000000000000000000, 1.000000000000000000 ) ) ;
#45750=ORIENTED_EDGE ( 'NONE', *, *, #26231, .F. ) ;
#45756=CARTESIAN_POINT ( 'NONE',  ( -3.062931151456462775, 1525.320827368860137, 241.4069010772119555 ) ) ;
#45759=CARTESIAN_POINT ( 'NONE',  ( -33.36586802512182715, 1518.913060387330006, 201.9069332299493169 ) ) ;
#45772=EDGE_CURVE ( 'NONE', #50084, #82691, #13888, .T. ) ;
#45797=CARTESIAN_POINT ( 'NONE',  ( -1.491506560153233352, 1511.187213306747708, 175.5704429466618421 ) ) ;
#45806=ORIENTED_EDGE ( 'NONE', *, *, #70687, .F. ) ;
#45830=CARTESIAN_POINT ( 'NONE',  ( 0.000000000000000000, 1511.187213306747708, 239.2297105040643714 ) ) ;
#45850=CARTESIAN_POINT ( 'NONE',  ( 32.02808312589922224, 1522.382868172863937, 219.9649204700462235 ) ) ;
#45858=FACE_OUTER_BOUND ( 'NONE', #92519, .T. ) ;
#45876=CARTESIAN_POINT ( 'NONE',  ( -2.131986625842082095, 1526.000688113726937, 240.6925538243687015 ) ) ;
#45879=CARTESIAN_POINT ( 'NONE',  ( -16.50400130224726780, 1525.907212628473644, 236.2546788475583242 ) ) ;
#45891=EDGE_CURVE ( 'NONE', #39734, #82569, #10397, .T. ) ;
#45892=CARTESIAN_POINT ( 'NONE',  ( -31.32941610406987820, 1525.856065479234758, 217.0550767640555136 ) ) ;
#45901=CARTESIAN_POINT ( 'NONE',  ( 2.470168521978402421, 1523.382868172864164, 242.8787258963054398 ) ) ;
#45909=ORIENTED_EDGE ( 'NONE', *, *, #27940, .F. ) ;
#45951=CARTESIAN_POINT ( 'NONE',  ( 16.85976061912576185, 1525.821544997590536, 236.1944305375347142 ) ) ;
#45970=AXIS2_PLACEMENT_3D ( 'NONE', #72169, #64865, #71634 ) ;
#45989=VECTOR ( 'NONE', #55515, 1000.000000000000000 ) ;
#46000=DIRECTION ( 'NONE',  ( -0.8642610224696035681, -0.000000000000000000, -0.5030436214085171054 ) ) ;
#46006=CARTESIAN_POINT ( 'NONE',  ( 17.16388877745050934, 1523.678648413191695, 179.6262614458745190 ) ) ;
#46009=CYLINDRICAL_SURFACE ( 'NONE', #67634, 1.000000000000000888 ) ;
#46023=DIRECTION ( 'NONE',  ( 0.9786619618251627406, 0.000000000000000000, -0.2054769195713317953 ) ) ;
#46027=CARTESIAN_POINT ( 'NONE',  ( 0.000000000000000000, 1518.913060387330006, 209.1218459616979999 ) ) ;
#46030=DIRECTION ( 'NONE',  ( -0.000000000000000000, -1.000000000000000000, -0.000000000000000000 ) ) ;
#46040=CARTESIAN_POINT ( 'NONE',  ( -17.30126322264801786, 1523.462669333490567, 237.3930845918954731 ) ) ;
#46069=ADVANCED_FACE ( 'NONE', ( #88202 ), #47296, .T. ) ;
#46075=AXIS2_PLACEMENT_3D ( 'NONE', #31825, #109643, #6626 ) ;
#46099=CARTESIAN_POINT ( 'NONE',  ( -16.89232299734799980, 1526.349689584397083, 234.8971085836487873 ) ) ;
#46121=VERTEX_POINT ( 'NONE', #81979 ) ;
#46139=CARTESIAN_POINT ( 'NONE',  ( -2.143765237719136518, 1525.848196786131211, 241.3832888336301323 ) ) ;
#46140=EDGE_CURVE ( 'NONE', #89941, #22899, #109961, .T. ) ;
#46158=ORIENTED_EDGE ( 'NONE', *, *, #91968, .T. ) ;
#46198=AXIS2_PLACEMENT_3D ( 'NONE', #28414, #20000, #54192 ) ;
#46201=DIRECTION ( 'NONE',  ( 0.000000000000000000, 0.000000000000000000, -1.000000000000000000 ) ) ;
#46228=CARTESIAN_POINT ( 'NONE',  ( -16.56816485275624373, 1526.186458717540290, 182.6341057012185445 ) ) ;
#46229=CARTESIAN_POINT ( 'NONE',  ( 21.46350454714117717, 1524.972383263452457, 234.5041546974912023 ) ) ;
#46230=ORIENTED_EDGE ( 'NONE', *, *, #80522, .T. ) ;
#46244=AXIS2_PLACEMENT_3D ( 'NONE', #80059, #106365, #12848 ) ;
#46252=CARTESIAN_POINT ( 'NONE',  ( 2.472529913803022783, 1523.678648413191695, 175.3762130535718597 ) ) ;
#46272=LINE ( 'NONE', #108349, #28728 ) ;
#46276=B_SPLINE_CURVE_WITH_KNOTS ( 'NONE', 3,
 ( #16028, #50757, #17114, #23338, #57530, #84355, #91654, #41258, #75959, #14928 ),
 .UNSPECIFIED., .F., .F.,
 ( 4, 2, 2, 2, 4 ),
 ( 0.000000000000000000, 0.0007403986298595364567, 0.001480797259719072913, 0.002221195889578609153, 0.002961594519438145827 ),
 .UNSPECIFIED. ) ;
#46311=VECTOR ( 'NONE', #103761, 1000.000000000000000 ) ;
#46313=CARTESIAN_POINT ( 'NONE',  ( -2.708816481115378760, 1524.478200376950781, 241.9482032910334510 ) ) ;
#46327=ORIENTED_EDGE ( 'NONE', *, *, #9754, .F. ) ;
#46330=DIRECTION ( 'NONE',  ( 0.9125304618753996566, 0.000000000000000000, 0.4090087482554252696 ) ) ;
#46344=CARTESIAN_POINT ( 'NONE',  ( 3.355892881418364837, 1523.847233649538339, 242.0621658074067852 ) ) ;
#46375=EDGE_CURVE ( 'NONE', #49270, #55773, #83685, .T. ) ;
#46383=ORIENTED_EDGE ( 'NONE', *, *, #59611, .F. ) ;
#46393=AXIS2_PLACEMENT_3D ( 'NONE', #35541, #79775, #108257 ) ;
#46398=EDGE_LOOP ( 'NONE', ( #6166, #12054, #94353, #33812 ) ) ;
#46409=CARTESIAN_POINT ( 'NONE',  ( 32.23107245337714488, 1523.542365884048195, 201.4053004075441038 ) ) ;
#46411=AXIS2_PLACEMENT_3D ( 'NONE', #1481, #55207, #37288 ) ;
#46414=CARTESIAN_POINT ( 'NONE',  ( -32.86802468386279941, 1523.481610426287716, 217.2040256693919957 ) ) ;
#46417=CARTESIAN_POINT ( 'NONE',  ( 20.98221433428943428, 1524.841055067849538, 237.1519650095368092 ) ) ;
#46428=CARTESIAN_POINT ( 'NONE',  ( -2.038646110889678287, 1525.960063244516959, 241.1857569150893994 ) ) ;
#46436=CARTESIAN_POINT ( 'NONE',  ( -16.56816485275871287, 1526.186458717539836, 235.6095862221776258 ) ) ;
#46456=VECTOR ( 'NONE', #65046, 1000.000000000000000 ) ;
#46467=ORIENTED_EDGE ( 'NONE', *, *, #46140, .T. ) ;
#46468=EDGE_LOOP ( 'NONE', ( #2690, #97705, #20712, #34999, #16869, #34809, #74736, #97807 ) ) ;
#46476=CARTESIAN_POINT ( 'NONE',  ( 32.36539537780658549, 1523.843271061948144, 202.1341907014572428 ) ) ;
#46487=DIRECTION ( 'NONE',  ( 0.000000000000000000, 1.000000000000000000, 0.000000000000000000 ) ) ;
#46508=ORIENTED_EDGE ( 'NONE', *, *, #19256, .T. ) ;
#46512=CARTESIAN_POINT ( 'NONE',  ( 16.77192111138402453, 1526.333389947941896, 234.9129815758702762 ) ) ;
#46530=AXIS2_PLACEMENT_3D ( 'NONE', #88358, #79957, #30083 ) ;
#46532=CARTESIAN_POINT ( 'NONE',  ( -204.2714532754874881, 1526.382868172863937, 194.5341519463070767 ) ) ;
#46543=CIRCLE ( 'NONE', #66212, 0.9999999999999947820 ) ;
#46571=DIRECTION ( 'NONE',  ( -0.000000000000000000, -1.000000000000000000, -0.000000000000000000 ) ) ;
#46572=CARTESIAN_POINT ( 'NONE',  ( 0.8350686643532178044, 1524.382868172863937, 177.3106345060153046 ) ) ;
#46576=AXIS2_PLACEMENT_3D ( 'NONE', #80694, #28078, #10742 ) ;
#46577=CARTESIAN_POINT ( 'NONE',  ( 17.06401309437439906, 1526.329757971584968, 181.0652997614131721 ) ) ;
#46582=EDGE_LOOP ( 'NONE', ( #14081, #96613, #79821, #64917, #67580, #15208, #48265, #79563 ) ) ;
#46583=CARTESIAN_POINT ( 'NONE',  ( 18.86688640473580847, 1511.187213306747708, 180.7825021045438518 ) ) ;
#46585=CARTESIAN_POINT ( 'NONE',  ( -32.02808312589908013, 1512.187213306747481, 221.9649204700466782 ) ) ;
#46596=LINE ( 'NONE', #72348, #55686 ) ;
#46607=CIRCLE ( 'NONE', #75209, 2.000000000000001776 ) ;
#46617=CARTESIAN_POINT ( 'NONE',  ( 20.55201027734717201, 1526.382868172863937, 181.8366482295329263 ) ) ;
#46619=DIRECTION ( 'NONE',  ( 0.000000000000000000, 1.000000000000000000, 0.000000000000000000 ) ) ;
#46621=DIRECTION ( 'NONE',  ( 0.000000000000000000, 1.000000000000000000, 0.000000000000000000 ) ) ;
#46630=VERTEX_POINT ( 'NONE', #101545 ) ;
#46652=ORIENTED_EDGE ( 'NONE', *, *, #24671, .T. ) ;
#46697=DIRECTION ( 'NONE',  ( 0.000000000000000000, 0.000000000000000000, 1.000000000000000000 ) ) ;
#46698=CARTESIAN_POINT ( 'NONE',  ( 16.69297358002692278, 1526.382868172864164, 183.6963177704308521 ) ) ;
#46701=DIRECTION ( 'NONE',  ( 0.5877852522924568168, 0.000000000000000000, -0.8090169943749592196 ) ) ;
#46715=EDGE_CURVE ( 'NONE', #56418, #23046, #79703, .T. ) ;
#46778=CARTESIAN_POINT ( 'NONE',  ( 21.15380500792148766, 1525.425686270224105, 234.2557952880171683 ) ) ;
#46781=ORIENTED_EDGE ( 'NONE', *, *, #23951, .F. ) ;
#46783=DIRECTION ( 'NONE',  ( 0.000000000000000000, 0.000000000000000000, 1.000000000000000000 ) ) ;
#46785=ADVANCED_FACE ( 'NONE', ( #107635 ), #28155, .F. ) ;
#46819=VECTOR ( 'NONE', #90022, 1000.000000000000114 ) ;
#46830=ORIENTED_EDGE ( 'NONE', *, *, #88448, .F. ) ;
#46840=EDGE_CURVE ( 'NONE', #75732, #51540, #17478, .T. ) ;
#46849=ORIENTED_EDGE ( 'NONE', *, *, #93911, .T. ) ;
#46857=CARTESIAN_POINT ( 'NONE',  ( -3.017180836140621825, 1525.408327360769817, 241.3338531177342929 ) ) ;
#46866=ORIENTED_EDGE ( 'NONE', *, *, #97442, .F. ) ;
#46867=CARTESIAN_POINT ( 'NONE',  ( 33.93019615848946557, 1524.726013923371283, 197.6607374645996344 ) ) ;
#46885=CARTESIAN_POINT ( 'NONE',  ( -2.038847259693655545, 1522.861859112239244, 244.9330574173661432 ) ) ;
#46890=EDGE_CURVE ( 'NONE', #66323, #101705, #49736, .T. ) ;
#46891=CARTESIAN_POINT ( 'NONE',  ( 34.68852446352035201, 1522.861859112239472, 199.9946320047950508 ) ) ;
#46904=CARTESIAN_POINT ( 'NONE',  ( 0.000000000000000000, 1526.382868172863937, 209.1218459616979999 ) ) ;
#46921=ADVANCED_FACE ( 'NONE', ( #101552 ), #67453, .T. ) ;
#46924=B_SPLINE_CURVE_WITH_KNOTS ( 'NONE', 3,
 ( #1228, #77921, #94715, #35364, #77377, #26971 ),
 .UNSPECIFIED., .F., .F.,
 ( 4, 2, 4 ),
 ( 3.469446951953614189E-17, 0.001087661325621730500, 0.002175322651243426306 ),
 .UNSPECIFIED. ) ;
#46926=ORIENTED_EDGE ( 'NONE', *, *, #108297, .T. ) ;
#46939=CARTESIAN_POINT ( 'NONE',  ( -33.13357216314875586, 1523.313115944345327, 217.3564597502661115 ) ) ;
#46955=CYLINDRICAL_SURFACE ( 'NONE', #85076, 1.000000000000000888 ) ;
#46956=FACE_OUTER_BOUND ( 'NONE', #57904, .T. ) ;
#46967=CARTESIAN_POINT ( 'NONE',  ( -20.55201027734757702, 1526.382868172863937, 181.8366482295332105 ) ) ;
#46973=CARTESIAN_POINT ( 'NONE',  ( -31.29224244793355680, 1525.661276915132476, 201.9587770753091718 ) ) ;
#46988=EDGE_LOOP ( 'NONE', ( #21756, #48740, #71742, #89720, #20423 ) ) ;
#46994=ORIENTED_EDGE ( 'NONE', *, *, #66712, .T. ) ;
#47002=CARTESIAN_POINT ( 'NONE',  ( 2.621078202464464546, 1523.542365884047967, 242.1599611597542037 ) ) ;
#47007=DIRECTION ( 'NONE',  ( -0.000000000000000000, -1.000000000000000000, -0.000000000000000000 ) ) ;
#47009=EDGE_CURVE ( 'NONE', #23879, #47496, #1539, .T. ) ;
#47010=ORIENTED_EDGE ( 'NONE', *, *, #9351, .T. ) ;
#47024=CARTESIAN_POINT ( 'NONE',  ( 2.596261494520225366, 1525.907212628473644, 240.7735774411713123 ) ) ;
#47045=CARTESIAN_POINT ( 'NONE',  ( -32.78250617288034618, 1512.187213306747481, 218.3079823578271430 ) ) ;
#47054=DIRECTION ( 'NONE',  ( 0.000000000000000000, 0.000000000000000000, 1.000000000000000000 ) ) ;
#47062=VERTEX_POINT ( 'NONE', #89741 ) ;
#47067=CARTESIAN_POINT ( 'NONE',  ( 2.372478608334043670, 1522.644714754858114, 174.8996806668799024 ) ) ;
#47068=CARTESIAN_POINT ( 'NONE',  ( -29.33475263078172546, 1526.373507135058617, 217.1429229503218039 ) ) ;
#47101=CARTESIAN_POINT ( 'NONE',  ( -21.71247731329013675, 1523.982201850120191, 234.6948375436862193 ) ) ;
#47115=CARTESIAN_POINT ( 'NONE',  ( 18.02257621027576562, 1526.382868172863937, 182.8951942368371988 ) ) ;
#47121=DIRECTION ( 'NONE',  ( 0.9510565162951478690, 0.000000000000000000, -0.3090169943749654369 ) ) ;
#47132=CARTESIAN_POINT ( 'NONE',  ( -16.68062049856698081, 1526.382868172863937, 236.8314524626096897 ) ) ;
#47135=CARTESIAN_POINT ( 'NONE',  ( -3.347801439372898979, 1523.456924617338245, 176.1543725842045376 ) ) ;
#47139=CARTESIAN_POINT ( 'NONE',  ( -31.43069643840468075, 1526.748660780343698, 216.5579808171739842 ) ) ;
#47152=CYLINDRICAL_SURFACE ( 'NONE', #98472, 0.9999999999999950040 ) ;
#47183=AXIS2_PLACEMENT_3D ( 'NONE', #10823, #105989, #44995 ) ;
#47211=CARTESIAN_POINT ( 'NONE',  ( -22.01290455779466271, 1522.906363951597314, 182.8785777331678446 ) ) ;
#47215=DIRECTION ( 'NONE',  ( -0.000000000000000000, -1.000000000000000000, -0.000000000000000000 ) ) ;
#47223=ORIENTED_EDGE ( 'NONE', *, *, #96690, .F. ) ;
#47238=FACE_OUTER_BOUND ( 'NONE', #59554, .T. ) ;
#47245=DIRECTION ( 'NONE',  ( -0.000000000000000000, -1.000000000000000000, -0.000000000000000000 ) ) ;
#47249=( BOUNDED_CURVE ( )  B_SPLINE_CURVE ( 3, ( #66473, #41786, #93287, #92736 ),
 .UNSPECIFIED., .F., .T. ) 
 B_SPLINE_CURVE_WITH_KNOTS ( ( 4, 4 ),
 ( 0.000000000000000000, 0.7048113239776826466 ),
 .UNSPECIFIED. ) 
 CURVE ( )  GEOMETRIC_REPRESENTATION_ITEM ( )  RATIONAL_B_SPLINE_CURVE ( ( 1.000000000000000000, 0.9590300661663233583, 0.9590300661663233583, 1.000000000000000000 ) ) 
 REPRESENTATION_ITEM ( '' )  );
#47255=CARTESIAN_POINT ( 'NONE',  ( 21.38516915557965703, 1501.977400791986611, 180.3939891059721106 ) ) ;
#47257=CARTESIAN_POINT ( 'NONE',  ( 30.90487439922560498, 1525.907212628473644, 216.4335774778780035 ) ) ;
#47263=CARTESIAN_POINT ( 'NONE',  ( 32.00465973459103708, 1524.843178112495480, 216.1170700846211901 ) ) ;
#47269=EDGE_CURVE ( 'NONE', #71507, #44004, #85504, .T. ) ;
#47286=VERTEX_POINT ( 'NONE', #103652 ) ;
#47295=CARTESIAN_POINT ( 'NONE',  ( -30.61443310237140381, 1523.382868172863937, 196.4193608261162467 ) ) ;
#47296=PLANE ( 'NONE',  #110469 ) ;
#47306=ORIENTED_EDGE ( 'NONE', *, *, #23299, .F. ) ;
#47332=AXIS2_PLACEMENT_3D ( 'NONE', #4001, #2363, #96950 ) ;
#47370=EDGE_CURVE ( 'NONE', #47286, #21147, #76658, .T. ) ;
#47380=EDGE_CURVE ( 'NONE', #79801, #77058, #19332, .T. ) ;
#47388=ADVANCED_FACE ( 'NONE', ( #42500 ), #65892, .T. ) ;
#47392=CARTESIAN_POINT ( 'NONE',  ( -2.596261494520262225, 1525.907212628473644, 240.7735774411712271 ) ) ;
#47405=CARTESIAN_POINT ( 'NONE',  ( -16.65010197087777399, 1526.345556099435726, 234.9005341682540973 ) ) ;
#47421=CARTESIAN_POINT ( 'NONE',  ( -19.01706420256807917, 1526.382868172863937, 185.3900685784704478 ) ) ;
#47424=CARTESIAN_POINT ( 'NONE',  ( 31.47409394596293453, 1526.278758871496848, 199.6577681796570118 ) ) ;
#47442=DIRECTION ( 'NONE',  ( 1.000000000000000000, 0.000000000000000000, 0.000000000000000000 ) ) ;
#47454=CIRCLE ( 'NONE', #27774, 1.000000000000000888 ) ;
#47455=( BOUNDED_SURFACE ( )  B_SPLINE_SURFACE ( 3, 2, ( 
 ( #9662, #84709, #43833 ),
 ( #50581, #41624, #59536 ),
 ( #18055, #77979, #76326 ),
 ( #61223, #68498, #103158 ),
 ( #109931, #85259, #60654 ),
 ( #93648, #77437, #102597 ),
 ( #25898, #110476, #43289 ),
 ( #8009, #196, #34869 ),
 ( #7462, #84161, #60096 ),
 ( #94212, #33208, #16931 ),
 ( #42728, #34320, #75778 ),
 ( #1287, #67398, #76887 ),
 ( #17487, #736, #101496 ),
 ( #69057, #51685, #26459 ) ),
 .UNSPECIFIED., .F., .F., .F. ) 
 B_SPLINE_SURFACE_WITH_KNOTS ( ( 4, 2, 2, 2, 2, 2, 4 ),
 ( 3, 3 ),
 ( 7.665309359472516348E-17, 0.0009443072508236404188, 0.001416460876235422356, 0.001888614501647204293, 0.002360768127058986230, 0.002832921752470767950, 0.003777229003294331824 ),
 ( 0.000000000000000000, 1.000000000000000000 ),
 .UNSPECIFIED. ) 
 GEOMETRIC_REPRESENTATION_ITEM ( )  RATIONAL_B_SPLINE_SURFACE ( (
 ( 1.000000000000000000, 0.9376006582765954445, 1.000000000000000000),
 ( 1.000000000000000000, 0.9283977714737452480, 1.000000000000000000),
 ( 1.000000000000000000, 0.9189750060478982796, 1.000000000000000000),
 ( 1.000000000000000000, 0.9042792056127966216, 1.000000000000000000),
 ( 1.000000000000000000, 0.8992469033839340931, 1.000000000000000000),
 ( 1.000000000000000000, 0.8891280264686174384, 1.000000000000000000),
 ( 1.000000000000000000, 0.8840337471669303948, 1.000000000000000000),
 ( 1.000000000000000000, 0.8736395124169680226, 1.000000000000000000),
 ( 1.000000000000000000, 0.8683406746541313392, 1.000000000000000000),
 ( 1.000000000000000000, 0.8573361860719177496, 1.000000000000000000),
 ( 1.000000000000000000, 0.8516508399498529114, 1.000000000000000000),
 ( 1.000000000000000000, 0.8340914917061317269, 1.000000000000000000),
 ( 1.000000000000000000, 0.8215597275865531568, 1.000000000000000000),
 ( 1.000000000000000000, 0.8070209408750207425, 1.000000000000000000) ) ) 
 REPRESENTATION_ITEM ( '' )  SURFACE ( )  );
#47474=CARTESIAN_POINT ( 'NONE',  ( -33.28034951413919629, 1522.862737210649811, 217.4407153818824554 ) ) ;
#47496=VERTEX_POINT ( 'NONE', #24858 ) ;
#47501=CARTESIAN_POINT ( 'NONE',  ( -31.92108011125358047, 1512.187213306747481, 197.2845127572065849 ) ) ;
#47504=CARTESIAN_POINT ( 'NONE',  ( 20.71343476517513338, 1501.977400791986611, 179.9059455038194528 ) ) ;
#47538=VECTOR ( 'NONE', #71496, 1000.000000000000000 ) ;
#47544=CARTESIAN_POINT ( 'NONE',  ( 1.191524307911311586, 1526.382868172863937, 179.0083900503167911 ) ) ;
#47546=PLANE ( 'NONE',  #79012 ) ;
#47552=VERTEX_POINT ( 'NONE', #53424 ) ;
#47564=DIRECTION ( 'NONE',  ( 0.000000000000000000, 0.000000000000000000, 1.000000000000000000 ) ) ;
#47598=ORIENTED_EDGE ( 'NONE', *, *, #62445, .F. ) ;
#47609=CARTESIAN_POINT ( 'NONE',  ( 0.4260839224734093711, 1523.429859730329781, 173.4147438076381604 ) ) ;
#47629=EDGE_CURVE ( 'NONE', #24499, #4978, #108382, .T. ) ;
#47641=CARTESIAN_POINT ( 'NONE',  ( 30.79106905599203969, 1526.107880201381477, 217.1184136641281839 ) ) ;
#47644=CARTESIAN_POINT ( 'NONE',  ( -32.52439779765793304, 1524.599984580802129, 201.1674557869507964 ) ) ;
#47650=VECTOR ( 'NONE', #84196, 1000.000000000000000 ) ;
#47656=EDGE_CURVE ( 'NONE', #83547, #97968, #31886, .T. ) ;
#47661=CARTESIAN_POINT ( 'NONE',  ( 17.44374831407675686, 1524.130440953581001, 180.7216696960668116 ) ) ;
#47666=ORIENTED_EDGE ( 'NONE', *, *, #87166, .T. ) ;
#47667=CARTESIAN_POINT ( 'NONE',  ( -17.36692773919844512, 1525.425665131969481, 181.2365449020387871 ) ) ;
#47681=AXIS2_PLACEMENT_3D ( 'NONE', #50468, #107601, #65064 ) ;
#47682=CARTESIAN_POINT ( 'NONE',  ( 2.165176160181045528, 1526.186458717538926, 177.9542909903756254 ) ) ;
#47700=DIRECTION ( 'NONE',  ( -0.9786619618251657382, 0.000000000000000000, 0.2054769195713184449 ) ) ;
#47710=ORIENTED_EDGE ( 'NONE', *, *, #66712, .F. ) ;
#47712=ORIENTED_EDGE ( 'NONE', *, *, #67067, .T. ) ;
#47761=CARTESIAN_POINT ( 'NONE',  ( -33.28034951413922471, 1512.187213306747481, 217.4407153818824838 ) ) ;
#47763=EDGE_CURVE ( 'NONE', #59940, #5947, #93681, .T. ) ;
#47767=( BOUNDED_CURVE ( )  B_SPLINE_CURVE ( 3, ( #54536, #52318, #44458, #78602 ),
 .UNSPECIFIED., .F., .F. ) 
 B_SPLINE_CURVE_WITH_KNOTS ( ( 4, 4 ),
 ( 2.436781329611989122, 3.141592653589793116 ),
 .UNSPECIFIED. ) 
 CURVE ( )  GEOMETRIC_REPRESENTATION_ITEM ( )  RATIONAL_B_SPLINE_CURVE ( ( 1.000000000000000000, 0.9590300661663093695, 0.9590300661663093695, 1.000000000000000000 ) ) 
 REPRESENTATION_ITEM ( '' )  );
#47770=VERTEX_POINT ( 'NONE', #97616 ) ;
#47800=TOROIDAL_SURFACE ( 'NONE', #55019, 2.000000000000000000, 1.000000000000000000 ) ;
#47806=CARTESIAN_POINT ( 'NONE',  ( 2.038646110889675178, 1525.960063244516959, 241.1857569150893994 ) ) ;
#47818=CARTESIAN_POINT ( 'NONE',  ( 31.33756689035257992, 1523.580203803270933, 221.9021554055875356 ) ) ;
#47821=CYLINDRICAL_SURFACE ( 'NONE', #8543, 1.000000000000000888 ) ;
#47845=CARTESIAN_POINT ( 'NONE',  ( -32.22536377336285085, 1523.621879633029039, 201.4085774011533090 ) ) ;
#47852=ORIENTED_EDGE ( 'NONE', *, *, #32415, .F. ) ;
#47853=CARTESIAN_POINT ( 'NONE',  ( -16.77192111137889441, 1526.333389947941896, 183.3307103475322322 ) ) ;
#47875=CARTESIAN_POINT ( 'NONE',  ( 2.493590731671294414, 1524.152444737676660, 175.5218342203271504 ) ) ;
#47879=CIRCLE ( 'NONE', #71164, 0.9999999999999976685 ) ;
#47896=VERTEX_POINT ( 'NONE', #6841 ) ;
#47898=CARTESIAN_POINT ( 'NONE',  ( 30.61443310214306024, 1523.462669333491704, 196.4193608261350334 ) ) ;
#47908=CARTESIAN_POINT ( 'NONE',  ( 30.04822308544837384, 1524.382868172804365, 221.7633950662767290 ) ) ;
#47933=VECTOR ( 'NONE', #21346, 1000.000000000000000 ) ;
#47934=CARTESIAN_POINT ( 'NONE',  ( 31.34491535884036040, 1525.848196786131211, 201.1913537499540894 ) ) ;
#47940=CARTESIAN_POINT ( 'NONE',  ( 0.000000000000000000, 1522.051704408389924, 209.1218459616979999 ) ) ;
#47949=ORIENTED_EDGE ( 'NONE', *, *, #76982, .T. ) ;
#47964=CIRCLE ( 'NONE', #110543, 2.000000000000001776 ) ;
#47977=EDGE_CURVE ( 'NONE', #41836, #42097, #83548, .T. ) ;
#47988=CYLINDRICAL_SURFACE ( 'NONE', #48443, 4.000000000000003553 ) ;
#47989=VERTEX_POINT ( 'NONE', #65676 ) ;
#47993=AXIS2_PLACEMENT_3D ( 'NONE', #35437, #27588, #1865 ) ;
#48004=EDGE_CURVE ( 'NONE', #37474, #10931, #56159, .T. ) ;
#48014=DIRECTION ( 'NONE',  ( -0.8642610224695934651, -1.396226527196591439E-14, -0.5030436214085343138 ) ) ;
#48046=CIRCLE ( 'NONE', #62389, 1.000000000000000888 ) ;
#48065=LINE ( 'NONE', #64885, #6774 ) ;
#48068=VECTOR ( 'NONE', #94965, 1000.000000000000000 ) ;
#48069=EDGE_CURVE ( 'NONE', #108182, #40151, #46924, .T. ) ;
#48085=CARTESIAN_POINT ( 'NONE',  ( -31.12456774391166547, 1525.960063244516959, 217.0912716842400130 ) ) ;
#48096=CARTESIAN_POINT ( 'NONE',  ( 22.69876404240077505, 1501.977400791986611, 181.3483716558180276 ) ) ;
#48105=EDGE_CURVE ( 'NONE', #73515, #106529, #81925, .T. ) ;
#48109=LINE ( 'NONE', #5548, #83984 ) ;
#48111=CYLINDRICAL_SURFACE ( 'NONE', #55489, 33.13701971169416538 ) ;
#48119=CARTESIAN_POINT ( 'NONE',  ( -30.51231035492526900, 1524.382868172863937, 200.0858385050243555 ) ) ;
#48124=CIRCLE ( 'NONE', #67790, 0.9999999999999981126 ) ;
#48126=CARTESIAN_POINT ( 'NONE',  ( 29.67167576298692566, 1526.344110814223313, 201.2571182723716845 ) ) ;
#48129=EDGE_CURVE ( 'NONE', #24247, #17035, #6868, .T. ) ;
#48141=ORIENTED_EDGE ( 'NONE', *, *, #108376, .F. ) ;
#48154=DIRECTION ( 'NONE',  ( 0.000000000000000000, 1.000000000000000000, 0.000000000000000000 ) ) ;
#48169=CARTESIAN_POINT ( 'NONE',  ( 0.4151546846839010985, 1522.906561336852974, 173.3106345060153046 ) ) ;
#48195=AXIS2_PLACEMENT_3D ( 'NONE', #2377, #11308, #37040 ) ;
#48204=EDGE_CURVE ( 'NONE', #98270, #13874, #66951, .T. ) ;
#48205=CARTESIAN_POINT ( 'NONE',  ( -31.93049531883793790, 1525.394081235439444, 201.2251851172232762 ) ) ;
#48206=CARTESIAN_POINT ( 'NONE',  ( 0.000000000000000000, 1524.090675761330203, 209.1218459616979999 ) ) ;
#48209=AXIS2_PLACEMENT_3D ( 'NONE', #48483, #65283, #33297 ) ;
#48215=CARTESIAN_POINT ( 'NONE',  ( -204.2714532754873744, 1524.382868172863937, 223.7095399770903725 ) ) ;
#48220=EDGE_CURVE ( 'NONE', #911, #83491, #54939, .T. ) ;
#48233=CARTESIAN_POINT ( 'NONE',  ( -17.83486663330467437, 1523.678648413191695, 237.8759530894961642 ) ) ;
#48262=EDGE_CURVE ( 'NONE', #72816, #30026, #71771, .T. ) ;
#48265=ORIENTED_EDGE ( 'NONE', *, *, #47656, .F. ) ;
#48271=VERTEX_POINT ( 'NONE', #86868 ) ;
#48274=CARTESIAN_POINT ( 'NONE',  ( -3.614223185717699405, 1512.187213306747481, 237.6097657867471469 ) ) ;
#48282=PRODUCT_CONTEXT ( 'NONE', #57061, 'mechanical' ) ;
#48298=CARTESIAN_POINT ( 'NONE',  ( -2.620401159595308727, 1523.462669333491021, 242.1631858338596146 ) ) ;
#48305=ORIENTED_EDGE ( 'NONE', *, *, #37265, .T. ) ;
#48317=CARTESIAN_POINT ( 'NONE',  ( 21.38516915557987375, 1512.187213306747481, 237.8497028174237471 ) ) ;
#48321=CARTESIAN_POINT ( 'NONE',  ( -19.90023153800462552, 1526.278758871497530, 182.9652379492368652 ) ) ;
#48333=DIRECTION ( 'NONE',  ( -0.000000000000000000, -1.000000000000000000, -0.000000000000000000 ) ) ;
#48340=LINE ( 'NONE', #74638, #39675 ) ;
#48354=CARTESIAN_POINT ( 'NONE',  ( 21.83550407203919974, 1523.678648413191695, 234.9693198511250785 ) ) ;
#48377=CARTESIAN_POINT ( 'NONE',  ( -20.21716934225085183, 1526.104292489130103, 184.5497256588658672 ) ) ;
#48384=DIRECTION ( 'NONE',  ( 0.000000000000000000, 1.000000000000000000, -0.000000000000000000 ) ) ;
#48389=CARTESIAN_POINT ( 'NONE',  ( 16.57695357295475347, 1524.524650307243292, 237.5563529681140835 ) ) ;
#48403=EDGE_CURVE ( 'NONE', #70982, #102300, #55191, .T. ) ;
#48413=CARTESIAN_POINT ( 'NONE',  ( -30.61443310214375657, 1523.462669333491476, 196.4193608261409452 ) ) ;
#48424=CARTESIAN_POINT ( 'NONE',  ( 22.08327125186925954, 1523.604703353109699, 184.4267662568470598 ) ) ;
#48425=B_SPLINE_CURVE_WITH_KNOTS ( 'NONE', 3,
 ( #98213, #29898, #64091, #4173, #21481, #89815 ),
 .UNSPECIFIED., .F., .F.,
 ( 4, 2, 4 ),
 ( -1.285435071114495078E-05, 0.001079388306740513117, 0.002171630964192170898 ),
 .UNSPECIFIED. ) ;
#48428=DIRECTION ( 'NONE',  ( 0.000000000000000000, 0.000000000000000000, -1.000000000000000000 ) ) ;
#48431=CARTESIAN_POINT ( 'NONE',  ( 30.51126001304307067, 1526.382868172863937, 198.3878992055866775 ) ) ;
#48438=( BOUNDED_CURVE ( )  B_SPLINE_CURVE ( 3, ( #16899, #34286, #51652, #100392 ),
 .UNSPECIFIED., .F., .F. ) 
 B_SPLINE_CURVE_WITH_KNOTS ( ( 4, 4 ),
 ( 3.141592653589793116, 4.712388980384689674 ),
 .UNSPECIFIED. ) 
 CURVE ( )  GEOMETRIC_REPRESENTATION_ITEM ( )  RATIONAL_B_SPLINE_CURVE ( ( 1.000000000000000000, 0.8047378541243649375, 0.8047378541243649375, 1.000000000000000000 ) ) 
 REPRESENTATION_ITEM ( '' )  );
#48443=AXIS2_PLACEMENT_3D ( 'NONE', #88886, #47442, #97279 ) ;
#48455=AXIS2_PLACEMENT_3D ( 'NONE', #58438, #75787, #16392 ) ;
#48462=CARTESIAN_POINT ( 'NONE',  ( 17.73225504275583830, 1524.152349020271004, 180.4731530606409819 ) ) ;
#48472=DIRECTION ( 'NONE',  ( 0.8672669759446630655, -0.000000000000000000, -0.4978433412588735285 ) ) ;
#48478=CARTESIAN_POINT ( 'NONE',  ( 33.43367350703651653, 1524.397344074318426, 220.4773507679699662 ) ) ;
#48483=CARTESIAN_POINT ( 'NONE',  ( 0.000000000000000000, 1518.913060387330006, 209.1218459616979999 ) ) ;
#48507=CIRCLE ( 'NONE', #16326, 1.000000000000000888 ) ;
#48508=FACE_OUTER_BOUND ( 'NONE', #77340, .T. ) ;
#48513=VERTEX_POINT ( 'NONE', #57702 ) ;
#48517=ORIENTED_EDGE ( 'NONE', *, *, #79618, .T. ) ;
#48520=CARTESIAN_POINT ( 'NONE',  ( -20.53760542139750456, 1525.821544997590536, 233.5223198772807507 ) ) ;
#48534=ORIENTED_EDGE ( 'NONE', *, *, #75449, .T. ) ;
#48542=AXIS2_PLACEMENT_3D ( 'NONE', #45012, #79157, #2465 ) ;
#48556=AXIS2_PLACEMENT_3D ( 'NONE', #48206, #18416, #563 ) ;
#48594=CARTESIAN_POINT ( 'NONE',  ( 22.08327125186943718, 1523.604703353109699, 233.8169256665487694 ) ) ;
#48613=B_SPLINE_CURVE_WITH_KNOTS ( 'NONE', 3,
 ( #33438, #69294, #8240, #93357, #51928, #16082 ),
 .UNSPECIFIED., .F., .F.,
 ( 4, 2, 4 ),
 ( -1.131363979615587220E-05, 0.001067788114096031088, 0.002146889867988218108 ),
 .UNSPECIFIED. ) ;
#48637=CARTESIAN_POINT ( 'NONE',  ( -30.31644210120117577, 1523.530870145311383, 222.4932309826520793 ) ) ;
#48639=CARTESIAN_POINT ( 'NONE',  ( 21.12212911287033279, 1512.187213306747481, 235.8226600804184443 ) ) ;
#48646=CARTESIAN_POINT ( 'NONE',  ( 34.18677586421187442, 1522.382868172863937, 219.7932833225211766 ) ) ;
#48659=DIRECTION ( 'NONE',  ( 0.000000000000000000, 1.000000000000000000, 0.000000000000000000 ) ) ;
#48663=CARTESIAN_POINT ( 'NONE',  ( 17.17241001986483795, 1518.913060387330006, 179.6185504016043240 ) ) ;
#48671=VECTOR ( 'NONE', #10246, 1000.000000000000114 ) ;
#48680=CARTESIAN_POINT ( 'NONE',  ( -29.86461515634900010, 1525.960063244516959, 220.9690070206027031 ) ) ;
#48688=ORIENTED_EDGE ( 'NONE', *, *, #102331, .T. ) ;
#48719=ORIENTED_EDGE ( 'NONE', *, *, #105597, .F. ) ;
#48740=ORIENTED_EDGE ( 'NONE', *, *, #2268, .T. ) ;
#48742=CIRCLE ( 'NONE', #82698, 2.000000000000004885 ) ;
#48752=CARTESIAN_POINT ( 'NONE',  ( 16.58770733237511052, 1524.425415513989037, 237.5950306126129590 ) ) ;
#48767=DIRECTION ( 'NONE',  ( 0.000000000000000000, 0.07083107041561081951, -0.9974883254774358221 ) ) ;
#48782=CARTESIAN_POINT ( 'NONE',  ( -17.22627284987310148, 1525.856065479244762, 181.7773037624300798 ) ) ;
#48785=CARTESIAN_POINT ( 'NONE',  ( 2.470955850358387718, 1523.580204110581235, 175.3687159778809814 ) ) ;
#48796=CARTESIAN_POINT ( 'NONE',  ( 17.84338787571921969, 1523.382868172864164, 180.3600277896298110 ) ) ;
#48798=EDGE_CURVE ( 'NONE', #90688, #30404, #85611, .T. ) ;
#48839=FACE_OUTER_BOUND ( 'NONE', #50856, .T. ) ;
#48844=ORIENTED_EDGE ( 'NONE', *, *, #63832, .F. ) ;
#48850=CARTESIAN_POINT ( 'NONE',  ( 18.19590854888164699, 1522.382868172863937, 238.2026672068774644 ) ) ;
#48862=ORIENTED_EDGE ( 'NONE', *, *, #65142, .T. ) ;
#48867=ADVANCED_FACE ( 'NONE', ( #2214 ), #8178, .T. ) ;
#48879=CARTESIAN_POINT ( 'NONE',  ( -19.63708787179735538, 1526.382868172863937, 183.4208852702759884 ) ) ;
#48885=DIRECTION ( 'NONE',  ( -0.8672669759446595128, -0.000000000000000000, 0.4978433412588795237 ) ) ;
#48887=CARTESIAN_POINT ( 'NONE',  ( -21.55491250604931608, 1524.059663615499630, 234.2080302846968891 ) ) ;
#48893=CARTESIAN_POINT ( 'NONE',  ( -16.64711273905149724, 1523.843263703803132, 237.7438622704431737 ) ) ;
#48917=FACE_OUTER_BOUND ( 'NONE', #79734, .T. ) ;
#48922=EDGE_CURVE ( 'NONE', #15037, #97242, #98153, .T. ) ;
#48934=CARTESIAN_POINT ( 'NONE',  ( 32.05523756949320813, 1525.253972588461465, 217.0243587599946409 ) ) ;
#48945=CARTESIAN_POINT ( 'NONE',  ( 16.51370421206613059, 1525.137906803776559, 237.1983439667824030 ) ) ;
#49007=CARTESIAN_POINT ( 'NONE',  ( 29.55269881708361979, 1525.821544997590536, 197.1295836072963539 ) ) ;
#49015=ORIENTED_EDGE ( 'NONE', *, *, #63868, .T. ) ;
#49028=CARTESIAN_POINT ( 'NONE',  ( 18.66420869458061205, 1526.382868172863937, 232.7837831374278039 ) ) ;
#49033=DIRECTION ( 'NONE',  ( 0.000000000000000000, 1.000000000000000000, 0.000000000000000000 ) ) ;
#49048=ORIENTED_EDGE ( 'NONE', *, *, #70715, .F. ) ;
#49056=ADVANCED_FACE ( 'NONE', ( #98433 ), #6960, .T. ) ;
#49059=LINE ( 'NONE', #73145, #50347 ) ;
#49090=DIRECTION ( 'NONE',  ( -0.000000000000000000, -1.000000000000000000, -0.000000000000000000 ) ) ;
#49111=AXIS2_PLACEMENT_3D ( 'NONE', #80903, #80356, #38331 ) ;
#49118=PLANE ( 'NONE',  #87397 ) ;
#49127=FACE_OUTER_BOUND ( 'NONE', #41490, .T. ) ;
#49163=DIRECTION ( 'NONE',  ( 0.000000000000000000, -1.000000000000000000, 0.000000000000000000 ) ) ;
#49166=DIRECTION ( 'NONE',  ( 0.000000000000000000, 1.000000000000000000, 0.000000000000000000 ) ) ;
#49174=ORIENTED_EDGE ( 'NONE', *, *, #27002, .T. ) ;
#49176=ORIENTED_EDGE ( 'NONE', *, *, #13686, .F. ) ;
#49192=CARTESIAN_POINT ( 'NONE',  ( 33.23571934791666393, 1511.187213306747708, 198.7594255952494677 ) ) ;
#49194=CARTESIAN_POINT ( 'NONE',  ( 34.18677586421137704, 1522.906561336852064, 219.7932833225227114 ) ) ;
#49198=ORIENTED_EDGE ( 'NONE', *, *, #98132, .T. ) ;
#49199=VERTEX_POINT ( 'NONE', #92789 ) ;
#49216=AXIS2_PLACEMENT_3D ( 'NONE', #50231, #48014, #75434 ) ;
#49246=CARTESIAN_POINT ( 'NONE',  ( -2.372478608332516892, 1522.382868172863937, 243.3440112565233449 ) ) ;
#49247=ORIENTED_EDGE ( 'NONE', *, *, #65142, .F. ) ;
#49270=VERTEX_POINT ( 'NONE', #17705 ) ;
#49280=CARTESIAN_POINT ( 'NONE',  ( 29.55269881708354163, 1525.821544997590308, 197.1295836072964391 ) ) ;
#49302=FACE_OUTER_BOUND ( 'NONE', #91137, .T. ) ;
#49323=CARTESIAN_POINT ( 'NONE',  ( -16.49871591222072809, 1525.320827368861501, 181.2023419493034169 ) ) ;
#49326=CARTESIAN_POINT ( 'NONE',  ( -3.451191875628180750, 1523.678648413191695, 243.0729557893954791 ) ) ;
#49334=CARTESIAN_POINT ( 'NONE',  ( -18.40343465886406094, 1525.402221411349501, 238.3904617729373001 ) ) ;
#49348=CARTESIAN_POINT ( 'NONE',  ( -18.86027053263874009, 1512.187213306747481, 230.7762769316009042 ) ) ;
#49365=DIRECTION ( 'NONE',  ( 0.9786619618251634067, 0.000000000000000000, -0.2054769195713292418 ) ) ;
#49377=EDGE_CURVE ( 'NONE', #31391, #105138, #68138, .T. ) ;
#49390=CARTESIAN_POINT ( 'NONE',  ( 33.36586802512179162, 1518.913060387330006, 216.3367586934468818 ) ) ;
#49397=EDGE_CURVE ( 'NONE', #95189, #31615, #28383, .T. ) ;
#49403=CARTESIAN_POINT ( 'NONE',  ( 32.02808312589916540, 1522.382868172863937, 198.2787714533495489 ) ) ;
#49413=CARTESIAN_POINT ( 'NONE',  ( -32.02808312589930040, 1511.187213306747708, 198.2787714533499752 ) ) ;
#49415=EDGE_CURVE ( 'NONE', #20993, #108510, #49895, .T. ) ;
#49422=EDGE_LOOP ( 'NONE', ( #76735, #42353, #43014, #32908 ) ) ;
#49426=B_SPLINE_CURVE_WITH_KNOTS ( 'NONE', 3,
 ( #19821, #87033, #88706, #54028 ),
 .UNSPECIFIED., .F., .F.,
 ( 4, 4 ),
 ( 0.000000000000000000, 0.0002220129587134773411 ),
 .UNSPECIFIED. ) ;
#49428=FACE_OUTER_BOUND ( 'NONE', #35866, .T. ) ;
#49434=CARTESIAN_POINT ( 'NONE',  ( -1.439851189675433574, 1526.382868172864164, 178.7402778767507243 ) ) ;
#49445=ORIENTED_EDGE ( 'NONE', *, *, #12608, .T. ) ;
#49475=CYLINDRICAL_SURFACE ( 'NONE', #14311, 33.13701971169416538 ) ;
#49490=CARTESIAN_POINT ( 'NONE',  ( 16.58903855651479020, 1524.412928176729110, 237.5994789871142814 ) ) ;
#49535=ORIENTED_EDGE ( 'NONE', *, *, #84859, .T. ) ;
#49556=CARTESIAN_POINT ( 'NONE',  ( 28.62766089293252136, 1526.344110814219675, 198.0439708941995605 ) ) ;
#49557=DIRECTION ( 'NONE',  ( 0.6709778558543655347, 0.000000000000000000, -0.7414773880254732497 ) ) ;
#49566=CARTESIAN_POINT ( 'NONE',  ( 30.31052258194586102, 1523.604703353109699, 195.7506062427368079 ) ) ;
#49572=CARTESIAN_POINT ( 'NONE',  ( -18.19590854888185305, 1522.382868172863937, 180.0410247165186490 ) ) ;
#49573=DIRECTION ( 'NONE',  ( -0.000000000000000000, -1.000000000000000000, -0.000000000000000000 ) ) ;
#49576=CARTESIAN_POINT ( 'NONE',  ( 33.93019615848955084, 1522.382868172863937, 220.5829544587960811 ) ) ;
#49577=ORIENTED_EDGE ( 'NONE', *, *, #45891, .T. ) ;
#49593=CARTESIAN_POINT ( 'NONE',  ( -20.88377839292641625, 1525.556090473914082, 184.5817676602346751 ) ) ;
#49598=EDGE_CURVE ( 'NONE', #17762, #90799, #77018, .T. ) ;
#49611=VERTEX_POINT ( 'NONE', #106443 ) ;
#49615=EDGE_LOOP ( 'NONE', ( #99110, #48862, #13130, #78577 ) ) ;
#49618=CARTESIAN_POINT ( 'NONE',  ( -20.70484064406360503, 1525.907212628473644, 233.2025904124107285 ) ) ;
#49624=CIRCLE ( 'NONE', #76461, 0.9999999999999865663 ) ;
#49626=CARTESIAN_POINT ( 'NONE',  ( -2.580915939757335575, 1524.130440953581001, 242.3512492075526552 ) ) ;
#49659=CARTESIAN_POINT ( 'NONE',  ( 22.69876404240077505, 1522.382868172863937, 181.3483716558180276 ) ) ;
#49662=EDGE_CURVE ( 'NONE', #54701, #28004, #41199, .T. ) ;
#49697=CARTESIAN_POINT ( 'NONE',  ( 17.04521188157742984, 1526.211528530236592, 182.6481290776079334 ) ) ;
#49707=VERTEX_POINT ( 'NONE', #90730 ) ;
#49718=CARTESIAN_POINT ( 'NONE',  ( -21.53712143570592730, 1523.621879633028584, 183.9400870382964968 ) ) ;
#49724=ORIENTED_EDGE ( 'NONE', *, *, #22731, .F. ) ;
#49725=AXIS2_PLACEMENT_3D ( 'NONE', #88033, #77954, #104261 ) ;
#49734=CARTESIAN_POINT ( 'NONE',  ( 20.17436656406337292, 1524.841055067847719, 180.5047911526335440 ) ) ;
#49736=CIRCLE ( 'NONE', #80184, 2.000000000000001776 ) ;
#49742=ORIENTED_EDGE ( 'NONE', *, *, #67514, .F. ) ;
#49743=DIRECTION ( 'NONE',  ( -1.000000000000000000, 0.000000000000000000, 0.000000000000000000 ) ) ;
#49750=DIRECTION ( 'NONE',  ( 0.000000000000000000, 1.000000000000000000, 0.000000000000000000 ) ) ;
#49751=CARTESIAN_POINT ( 'NONE',  ( -32.02808312589908013, 1501.977400791986611, 219.9649204700466782 ) ) ;
#49755=CARTESIAN_POINT ( 'NONE',  ( -29.36867415615329335, 1526.382868172863937, 200.9843407519612981 ) ) ;
#49763=CARTESIAN_POINT ( 'NONE',  ( 32.85805783624308418, 1523.678648413191695, 217.1983043299902931 ) ) ;
#49764=ORIENTED_EDGE ( 'NONE', *, *, #54811, .F. ) ;
#49769=ADVANCED_FACE ( 'NONE', ( #49302 ), #30271, .T. ) ;
#49775=CARTESIAN_POINT ( 'NONE',  ( -34.68852446352935459, 1522.382868172863937, 218.2490599186011764 ) ) ;
#49779=VECTOR ( 'NONE', #89421, 1000.000000000000000 ) ;
#49795=ORIENTED_EDGE ( 'NONE', *, *, #67279, .F. ) ;
#49802=VERTEX_POINT ( 'NONE', #81770 ) ;
#49819=EDGE_LOOP ( 'NONE', ( #72629, #53078, #25402 ) ) ;
#49826=CARTESIAN_POINT ( 'NONE',  ( -16.66936639845609847, 1512.187213306747481, 237.7608804993221838 ) ) ;
#49833=CARTESIAN_POINT ( 'NONE',  ( 29.61076903484002898, 1526.107876515966609, 220.7510285220318167 ) ) ;
#49841=CARTESIAN_POINT ( 'NONE',  ( 0.000000000000000000, 1526.382868172863937, 209.1218459616979999 ) ) ;
#49843=CARTESIAN_POINT ( 'NONE',  ( 18.19590854888164699, 1522.382868172863937, 238.2026672068774644 ) ) ;
#49861=DIRECTION ( 'NONE',  ( 0.9774101051267758411, 0.000000000000000000, 0.2113515706023144369 ) ) ;
#49866=CARTESIAN_POINT ( 'NONE',  ( -18.66420869458026388, 1526.382868172863937, 232.7837831374280881 ) ) ;
#49867=ORIENTED_EDGE ( 'NONE', *, *, #54225, .T. ) ;
#49868=CARTESIAN_POINT ( 'NONE',  ( 1.313045906442016575, 1526.382868172864619, 178.8771780891984804 ) ) ;
#49875=CARTESIAN_POINT ( 'NONE',  ( -16.58903855651428572, 1524.412928176728428, 180.6442129362811784 ) ) ;
#49878=CARTESIAN_POINT ( 'NONE',  ( -16.53242990339613883, 1526.073434386619283, 182.3092812937424583 ) ) ;
#49888=ORIENTED_EDGE ( 'NONE', *, *, #83701, .T. ) ;
#49893=EDGE_LOOP ( 'NONE', ( #9832, #105017, #55741, #12096, #66627 ) ) ;
#49895=CIRCLE ( 'NONE', #3385, 1.000000000000009104 ) ;
#49899=PLANE ( 'NONE',  #98388 ) ;
#49905=CARTESIAN_POINT ( 'NONE',  ( -29.74444329485024596, 1526.348417187218502, 217.2213265034480969 ) ) ;
#49930=ORIENTED_EDGE ( 'NONE', *, *, #109496, .F. ) ;
#49931=VERTEX_POINT ( 'NONE', #85078 ) ;
#49966=ORIENTED_EDGE ( 'NONE', *, *, #93911, .F. ) ;
#49975=ORIENTED_EDGE ( 'NONE', *, *, #65090, .T. ) ;
#50013=FACE_OUTER_BOUND ( 'NONE', #56540, .T. ) ;
#50021=CARTESIAN_POINT ( 'NONE',  ( -19.38211899475993860, 1526.344110814221267, 185.3185741806069871 ) ) ;
#50026=DIRECTION ( 'NONE',  ( -0.000000000000000000, -1.000000000000000000, -0.000000000000000000 ) ) ;
#50027=CIRCLE ( 'NONE', #32112, 1.000000000000000888 ) ;
#50041=EDGE_CURVE ( 'NONE', #13824, #58183, #54282, .T. ) ;
#50050=CIRCLE ( 'NONE', #23244, 2.000000000000003109 ) ;
#50057=VERTEX_POINT ( 'NONE', #96258 ) ;
#50061=( BOUNDED_SURFACE ( )  B_SPLINE_SURFACE ( 3, 2, ( 
 ( #22983, #30846, #58274 ),
 ( #108103, #82366, #73424 ),
 ( #92397, #66145, #101333 ),
 ( #49875, #99691, #24623 ),
 ( #58820, #39250, #31399 ),
 ( #57188, #91312, #57739 ),
 ( #107560, #13477, #32517 ),
 ( #65022, #14594, #84008 ),
 ( #15133, #75634, #100268 ),
 ( #49323, #23547, #47667 ),
 ( #5097, #99140, #15670 ),
 ( #5664, #22417, #65579 ),
 ( #14034, #39812, #48782 ),
 ( #40351, #40903, #74532 ) ),
 .UNSPECIFIED., .F., .F., .T. ) 
 B_SPLINE_SURFACE_WITH_KNOTS ( ( 4, 2, 2, 2, 2, 2, 4 ),
 ( 3, 3 ),
 ( 0.000000000000000000, 0.0009440840677143893080, 0.001416126101571584016, 0.001888168135428778616, 0.002360210169285973433, 0.002832252203143168032, 0.003776336270857557232 ),
 ( 0.000000000000000000, 1.000000000000000000 ),
 .UNSPECIFIED. ) 
 GEOMETRIC_REPRESENTATION_ITEM ( )  RATIONAL_B_SPLINE_SURFACE ( (
 ( 1.000000000000000000, 0.8070209408750173008, 1.000000000000000000),
 ( 1.000000000000000000, 0.8215603905299677656, 1.000000000000000000),
 ( 1.000000000000000000, 0.8340988699039975085, 1.000000000000000000),
 ( 1.000000000000000000, 0.8516751610468989986, 1.000000000000000000),
 ( 1.000000000000000000, 0.8573697395150979839, 1.000000000000000000),
 ( 1.000000000000000000, 0.8683586635665277997, 1.000000000000000000),
 ( 1.000000000000000000, 0.8736518481714815598, 1.000000000000000000),
 ( 1.000000000000000000, 0.8840377753023912488, 1.000000000000000000),
 ( 1.000000000000000000, 0.8891294171303538718, 1.000000000000000000),
 ( 1.000000000000000000, 0.8992456600576697046, 1.000000000000000000),
 ( 1.000000000000000000, 0.9042785869253191500, 1.000000000000000000),
 ( 1.000000000000000000, 0.9189749222837818587, 1.000000000000000000),
 ( 1.000000000000000000, 0.9283978182348824326, 1.000000000000000000),
 ( 1.000000000000000000, 0.9376006582765940012, 1.000000000000000000) ) ) 
 REPRESENTATION_ITEM ( '' )  SURFACE ( )  );
#50067=CARTESIAN_POINT ( 'NONE',  ( 17.84338787571921969, 1501.977400791986611, 180.3600277896298110 ) ) ;
#50079=AXIS2_PLACEMENT_3D ( 'NONE', #17575, #49573, #93201 ) ;
#50084=VERTEX_POINT ( 'NONE', #18970 ) ;
#50097=ORIENTED_EDGE ( 'NONE', *, *, #82206, .F. ) ;
#50117=CIRCLE ( 'NONE', #7174, 2.000000000000001776 ) ;
#50135=EDGE_CURVE ( 'NONE', #63792, #30404, #36016, .T. ) ;
#50148=CARTESIAN_POINT ( 'NONE',  ( -20.49599333844888349, 1525.960063244516959, 184.3798832129037635 ) ) ;
#50171=CARTESIAN_POINT ( 'NONE',  ( -20.20959865099451847, 1511.187213306747708, 236.2316688286741453 ) ) ;
#50178=ADVANCED_FACE ( 'NONE', ( #3693 ), #68080, .T. ) ;
#50184=EDGE_CURVE ( 'NONE', #57810, #967, #86746, .T. ) ;
#50198=CIRCLE ( 'NONE', #51942, 1.999999999999996669 ) ;
#50208=ORIENTED_EDGE ( 'NONE', *, *, #23454, .F. ) ;
#50225=AXIS2_PLACEMENT_3D ( 'NONE', #18464, #110343, #33616 ) ;
#50231=CARTESIAN_POINT ( 'NONE',  ( 16.16632277704778176, 1512.187213306747481, 181.3470724465435069 ) ) ;
#50250=CIRCLE ( 'NONE', #59202, 1.000000000000000888 ) ;
#50259=CARTESIAN_POINT ( 'NONE',  ( 19.53786426059039982, 1511.187213306747708, 236.7197124308265188 ) ) ;
#50269=CARTESIAN_POINT ( 'NONE',  ( 2.646287650837769956, 1525.055427061254704, 176.5934666753861677 ) ) ;
#50282=EDGE_CURVE ( 'NONE', #55064, #79230, #8764, .T. ) ;
#50290=CIRCLE ( 'NONE', #48455, 32.13701971169416538 ) ;
#50299=TOROIDAL_SURFACE ( 'NONE', #2029, 32.13701971169416538, 1.000000000000000000 ) ;
#50305=ORIENTED_EDGE ( 'NONE', *, *, #63312, .F. ) ;
#50331=AXIS2_PLACEMENT_3D ( 'NONE', #93196, #57967, #74767 ) ;
#50347=VECTOR ( 'NONE', #13757, 1000.000000000000000 ) ;
#50351=CARTESIAN_POINT ( 'NONE',  ( -2.471035510942674485, 1525.556090473913855, 176.9933286210197423 ) ) ;
#50356=CARTESIAN_POINT ( 'NONE',  ( -33.93019615848960768, 1512.187213306747481, 197.6607374646001176 ) ) ;
#50357=CARTESIAN_POINT ( 'NONE',  ( -34.18677586421195969, 1512.187213306747481, 198.4504086008750505 ) ) ;
#50358=ORIENTED_EDGE ( 'NONE', *, *, #26227, .T. ) ;
#50363=ORIENTED_EDGE ( 'NONE', *, *, #956, .F. ) ;
#50371=DIRECTION ( 'NONE',  ( 0.7882878497004317531, 0.000000000000000000, 0.6153066438895888890 ) ) ;
#50387=CARTESIAN_POINT ( 'NONE',  ( 30.51923195337197114, 1524.059547553518769, 196.3739828646224055 ) ) ;
#50392=CARTESIAN_POINT ( 'NONE',  ( 2.865544263339262265, 1525.651286436460623, 241.1072443789812496 ) ) ;
#50399=( BOUNDED_CURVE ( )  B_SPLINE_CURVE ( 3, ( #42853, #59661, #42292, #100536 ),
 .UNSPECIFIED., .F., .F. ) 
 B_SPLINE_CURVE_WITH_KNOTS ( ( 4, 4 ),
 ( 4.712388980384689674, 6.283185307179586232 ),
 .UNSPECIFIED. ) 
 CURVE ( )  GEOMETRIC_REPRESENTATION_ITEM ( )  RATIONAL_B_SPLINE_CURVE ( ( 1.000000000000000000, 0.8047378541243649375, 0.8047378541243649375, 1.000000000000000000 ) ) 
 REPRESENTATION_ITEM ( '' )  );
#50402=CIRCLE ( 'NONE', #16379, 23.69926344187880929 ) ;
#50418=DIRECTION ( 'NONE',  ( 0.4978433412588673113, 0.000000000000000000, -0.8672669759446667292 ) ) ;
#50419=LINE ( 'NONE', #83993, #32564 ) ;
#50422=DIRECTION ( 'NONE',  ( 0.7414773880254711402, -0.000000000000000000, 0.6709778558543678662 ) ) ;
#50425=AXIS2_PLACEMENT_3D ( 'NONE', #57653, #16148, #73886 ) ;
#50430=CARTESIAN_POINT ( 'NONE',  ( 0.000000000000000000, 1526.382868172863937, 209.1218459616979999 ) ) ;
#50436=CARTESIAN_POINT ( 'NONE',  ( 3.348647037815641436, 1523.530870145310701, 176.1572109406605193 ) ) ;
#50440=DIRECTION ( 'NONE',  ( -0.000000000000000000, 1.000000000000000000, -0.000000000000000000 ) ) ;
#50443=DIRECTION ( 'NONE',  ( 0.000000000000000000, 0.000000000000000000, 1.000000000000000000 ) ) ;
#50445=EDGE_CURVE ( 'NONE', #53780, #1895, #89475, .T. ) ;
#50448=LINE ( 'NONE', #100809, #46819 ) ;
#50453=EDGE_CURVE ( 'NONE', #12155, #87976, #59121, .T. ) ;
#50454=CARTESIAN_POINT ( 'NONE',  ( -20.71343476517554905, 1522.382868172863937, 179.9059455038197086 ) ) ;
#50458=DIRECTION ( 'NONE',  ( 0.000000000000000000, 0.000000000000000000, 1.000000000000000000 ) ) ;
#50468=CARTESIAN_POINT ( 'NONE',  ( 32.28466283162151029, 1522.382868172863937, 199.0684425896244250 ) ) ;
#50489=DIRECTION ( 'NONE',  ( 0.000000000000000000, 1.000000000000000000, 0.000000000000000000 ) ) ;
#50494=CARTESIAN_POINT ( 'NONE',  ( 17.83486663330506872, 1523.678648413191695, 237.8759530894958800 ) ) ;
#50502=CARTESIAN_POINT ( 'NONE',  ( 30.11977250498251379, 1524.538768545234007, 222.3783518056995945 ) ) ;
#50505=VERTEX_POINT ( 'NONE', #71497 ) ;
#50508=VERTEX_POINT ( 'NONE', #70380 ) ;
#50545=ORIENTED_EDGE ( 'NONE', *, *, #21926, .T. ) ;
#50566=CARTESIAN_POINT ( 'NONE',  ( -30.30249668296272958, 1524.678872986481338, 196.4365537040479239 ) ) ;
#50568=DIRECTION ( 'NONE',  ( 0.8090169943749422332, 0.000000000000000000, -0.5877852522924802425 ) ) ;
#50573=CARTESIAN_POINT ( 'NONE',  ( -16.55108609117688445, 1524.760046179776054, 237.4542795853993482 ) ) ;
#50581=CARTESIAN_POINT ( 'NONE',  ( 16.48400364722103362, 1525.790286462515496, 181.7637252794370397 ) ) ;
#50584=CARTESIAN_POINT ( 'NONE',  ( 16.49871591221882738, 1525.320827368860819, 237.0413499740942029 ) ) ;
#50600=ORIENTED_EDGE ( 'NONE', *, *, #25098, .T. ) ;
#50615=ORIENTED_EDGE ( 'NONE', *, *, #48204, .T. ) ;
#50617=VERTEX_POINT ( 'NONE', #97193 ) ;
#50625=LINE ( 'NONE', #101003, #21454 ) ;
#50633=CARTESIAN_POINT ( 'NONE',  ( -2.309262712062270850, 1512.187213306747481, 217.7723287588028995 ) ) ;
#50655=ORIENTED_EDGE ( 'NONE', *, *, #79634, .F. ) ;
#50666=VERTEX_POINT ( 'NONE', #94296 ) ;
#50670=CARTESIAN_POINT ( 'NONE',  ( -31.50799703744276670, 1526.382868172863709, 216.4233194664831785 ) ) ;
#50680=CARTESIAN_POINT ( 'NONE',  ( -21.08703188482416380, 1525.317359687841190, 184.4717570622386518 ) ) ;
#50681=CYLINDRICAL_SURFACE ( 'NONE', #72549, 1.000000000000000888 ) ;
#50706=FACE_OUTER_BOUND ( 'NONE', #20573, .T. ) ;
#50713=CARTESIAN_POINT ( 'NONE',  ( -2.397475438392928204, 1525.713797967456912, 243.2249543484664116 ) ) ;
#50721=ORIENTED_EDGE ( 'NONE', *, *, #77606, .F. ) ;
#50727=LINE ( 'NONE', #57502, #1790 ) ;
#50752=DIRECTION ( 'NONE',  ( 0.000000000000000000, 0.000000000000000000, 1.000000000000000000 ) ) ;
#50757=CARTESIAN_POINT ( 'NONE',  ( 31.26701538686466719, 1523.919934424249959, 196.3491293340342736 ) ) ;
#50770=CARTESIAN_POINT ( 'NONE',  ( -18.02257621027557377, 1526.382868172863937, 235.3484976865589147 ) ) ;
#50778=CARTESIAN_POINT ( 'NONE',  ( -2.738357492517908387, 1525.795403621571040, 240.9366226831509437 ) ) ;
#50788=DIRECTION ( 'NONE',  ( -0.000000000000000000, 1.000000000000000000, -0.000000000000000000 ) ) ;
#50798=ADVANCED_FACE ( 'NONE', ( #63513 ), #73938, .F. ) ;
#50801=CARTESIAN_POINT ( 'NONE',  ( 3.062931151456462775, 1525.320827368860137, 176.8367908461840443 ) ) ;
#50829=DIRECTION ( 'NONE',  ( 0.000000000000000000, -1.000000000000000000, 0.000000000000000000 ) ) ;
#50841=CARTESIAN_POINT ( 'NONE',  ( -2.407253779970412566, 1523.313115944345554, 243.1783812783781116 ) ) ;
#50842=CIRCLE ( 'NONE', #100855, 2.000000000000001776 ) ;
#50856=EDGE_LOOP ( 'NONE', ( #58201, #47712, #12689, #67063 ) ) ;
#50862=EDGE_CURVE ( 'NONE', #67358, #61077, #16342, .T. ) ;
#50864=CARTESIAN_POINT ( 'NONE',  ( 28.27139721233048419, 1526.382868172863937, 219.5606225550385489 ) ) ;
#50894=ORIENTED_EDGE ( 'NONE', *, *, #52970, .T. ) ;
#50904=ADVANCED_FACE ( 'NONE', ( #93068 ), #80685, .T. ) ;
#50912=EDGE_LOOP ( 'NONE', ( #70894, #28562, #88986, #53053 ) ) ;
#50929=DIRECTION ( 'NONE',  ( 0.000000000000000000, 1.000000000000000000, 0.000000000000000000 ) ) ;
#50932=CIRCLE ( 'NONE', #79554, 32.13701971169416538 ) ;
#50933=EDGE_CURVE ( 'NONE', #100321, #24499, #44060, .T. ) ;
#50936=FACE_OUTER_BOUND ( 'NONE', #55619, .T. ) ;
#50946=CARTESIAN_POINT ( 'NONE',  ( -33.42844755917204225, 1501.977400791986611, 196.1165140606796058 ) ) ;
#50962=CARTESIAN_POINT ( 'NONE',  ( 31.41104781486823327, 1512.187213306747481, 215.9140555522422460 ) ) ;
#50977=DIRECTION ( 'NONE',  ( 0.000000000000000000, 0.000000000000000000, 1.000000000000000000 ) ) ;
#50979=DIRECTION ( 'NONE',  ( 0.01594118961724027769, -0.9969860201949399814, 0.07592597717146752634 ) ) ;
#50999=DIRECTION ( 'NONE',  ( -0.9942586961433751425, 0.000000000000000000, 0.1070030146457376097 ) ) ;
#51008=CARTESIAN_POINT ( 'NONE',  ( -31.99468309217327189, 1524.860077346005255, 216.1184527756807370 ) ) ;
#51011=ORIENTED_EDGE ( 'NONE', *, *, #88612, .T. ) ;
#51013=EDGE_LOOP ( 'NONE', ( #25033, #92826, #53093, #9298 ) ) ;
#51036=EDGE_CURVE ( 'NONE', #17035, #66323, #104239, .T. ) ;
#51072=EDGE_CURVE ( 'NONE', #84410, #76626, #88013, .T. ) ;
#51077=CARTESIAN_POINT ( 'NONE',  ( -21.26059330700258343, 1525.055427061272212, 233.8824087493117929 ) ) ;
#51079=ADVANCED_FACE ( 'NONE', ( #105345 ), #18007, .F. ) ;
#51084=CYLINDRICAL_SURFACE ( 'NONE', #29847, 1.999999999999995781 ) ;
#51094=CARTESIAN_POINT ( 'NONE',  ( -2.472529913803022783, 1523.678648413191695, 242.8674788698241400 ) ) ;
#51098=CARTESIAN_POINT ( 'NONE',  ( -19.37374569213905318, 1526.382868172863937, 234.3668155954421479 ) ) ;
#51119=DIRECTION ( 'NONE',  ( 0.9149707217702551798, 0.000000000000000000, -0.4035202328300510621 ) ) ;
#51151=CARTESIAN_POINT ( 'NONE',  ( 21.46337646344914774, 1524.972613296804866, 183.7396512953049807 ) ) ;
#51152=EDGE_LOOP ( 'NONE', ( #33509, #110372, #90621 ) ) ;
#51168=EDGE_LOOP ( 'NONE', ( #103636, #34338, #70198, #25013 ) ) ;
#51178=TOROIDAL_SURFACE ( 'NONE', #72600, 30.13701971169416538, 3.000000000000000000 ) ;
#51184=EDGE_CURVE ( 'NONE', #5789, #72142, #94991, .T. ) ;
#51192=PLANE ( 'NONE',  #110664 ) ;
#51193=CARTESIAN_POINT ( 'NONE',  ( 19.63708787179688287, 1526.382868172863937, 183.4208852702759316 ) ) ;
#51196=AXIS2_PLACEMENT_3D ( 'NONE', #1654, #61019, #10031 ) ;
#51202=CARTESIAN_POINT ( 'NONE',  ( 29.75841426814800528, 1525.320827368874461, 222.0114972872726469 ) ) ;
#51208=CARTESIAN_POINT ( 'NONE',  ( 20.70484064406403846, 1525.907212628473644, 233.2025904124105580 ) ) ;
#51216=VERTEX_POINT ( 'NONE', #43783 ) ;
#51219=CARTESIAN_POINT ( 'NONE',  ( 32.02808312589922224, 1512.187213306747481, 220.9649204700462235 ) ) ;
#51230=CARTESIAN_POINT ( 'NONE',  ( -21.83181799873807805, 1524.739563915922190, 184.6224812385471523 ) ) ;
#51238=CARTESIAN_POINT ( 'NONE',  ( -33.23571934791680604, 1512.187213306747481, 198.7594255952499793 ) ) ;
#51268=( GEOMETRIC_REPRESENTATION_CONTEXT ( 3 ) GLOBAL_UNCERTAINTY_ASSIGNED_CONTEXT ( ( #88268 ) ) GLOBAL_UNIT_ASSIGNED_CONTEXT ( ( #2428, #77452, #53367 ) ) REPRESENTATION_CONTEXT ( 'NONE', 'WORKASPACE' ) );
#51285=DIRECTION ( 'NONE',  ( -1.000000000000000000, 0.000000000000000000, 0.000000000000000000 ) ) ;
#51312=AXIS2_PLACEMENT_3D ( 'NONE', #50962, #74520, #49861 ) ;
#51314=CARTESIAN_POINT ( 'NONE',  ( -16.66936639845609491, 1523.382868172864164, 237.7608804993221838 ) ) ;
#51327=CARTESIAN_POINT ( 'NONE',  ( -16.52275697106984609, 1525.042337199239910, 237.2696949994484328 ) ) ;
#51344=CARTESIAN_POINT ( 'NONE',  ( 2.472529913803020563, 1523.678648413191695, 175.3762130535718597 ) ) ;
#51360=AXIS2_PLACEMENT_3D ( 'NONE', #49413, #76808, #84093 ) ;
#51365=DIRECTION ( 'NONE',  ( -0.1070030146457375958, 0.000000000000000000, -0.9942586961433750314 ) ) ;
#51368=EDGE_CURVE ( 'NONE', #84088, #109192, #78761, .T. ) ;
#51381=ORIENTED_EDGE ( 'NONE', *, *, #67201, .F. ) ;
#51393=CARTESIAN_POINT ( 'NONE',  ( 21.38516915557965703, 1522.382868172863937, 180.3939891059721106 ) ) ;
#51399=CIRCLE ( 'NONE', #97830, 30.13701971169416183 ) ;
#51406=DIRECTION ( 'NONE',  ( 0.000000000000000000, 0.000000000000000000, -1.000000000000000000 ) ) ;
#51436=DIRECTION ( 'NONE',  ( -0.000000000000000000, -1.000000000000000000, -0.000000000000000000 ) ) ;
#51489=ADVANCED_FACE ( 'NONE', ( #33997 ), #85354, .F. ) ;
#51517=CARTESIAN_POINT ( 'NONE',  ( -31.92299894892000722, 1524.776010967693992, 216.6640755986756517 ) ) ;
#51519=ORIENTED_EDGE ( 'NONE', *, *, #101280, .F. ) ;
#51523=CARTESIAN_POINT ( 'NONE',  ( -16.71509328323223187, 1526.382868172864391, 183.8816066442305726 ) ) ;
#51526=AXIS2_PLACEMENT_3D ( 'NONE', #28560, #46487, #21220 ) ;
#51540=VERTEX_POINT ( 'NONE', #89913 ) ;
#51543=DIRECTION ( 'NONE',  ( 0.03006000153037601333, -0.4884709562387480331, 0.8720622232496927362 ) ) ;
#51558=CARTESIAN_POINT ( 'NONE',  ( -31.79838993233234490, 1525.159177407156449, 216.1507442378014332 ) ) ;
#51560=CIRCLE ( 'NONE', #62305, 1.000000000000001554 ) ;
#51624=CARTESIAN_POINT ( 'NONE',  ( -20.72500064278883158, 1525.697947650517563, 233.5887215935848644 ) ) ;
#51630=DIRECTION ( 'NONE',  ( -0.8672669759446596238, 0.000000000000000000, 0.4978433412588795792 ) ) ;
#51631=ADVANCED_FACE ( 'NONE', ( #67500 ), #77541, .T. ) ;
#51652=CARTESIAN_POINT ( 'NONE',  ( -32.30068554584597962, 1526.382868172863937, 220.2363794648147746 ) ) ;
#51667=CARTESIAN_POINT ( 'NONE',  ( -31.32995031131208918, 1523.678648413191695, 196.3423562208917588 ) ) ;
#51668=AXIS2_PLACEMENT_3D ( 'NONE', #21665, #55872, #82142 ) ;
#51675=EDGE_CURVE ( 'NONE', #44415, #50505, #84809, .T. ) ;
#51677=CARTESIAN_POINT ( 'NONE',  ( 33.23571934791667104, 1511.187213306747708, 198.7594255952494962 ) ) ;
#51678=FACE_OUTER_BOUND ( 'NONE', #72130, .T. ) ;
#51681=CARTESIAN_POINT ( 'NONE',  ( -22.08622291482368283, 1512.187213306747481, 184.4183880513178337 ) ) ;
#51685=CARTESIAN_POINT ( 'NONE',  ( 17.29393938232457728, 1523.621879633028811, 180.8572348224458324 ) ) ;
#51687=CARTESIAN_POINT ( 'NONE',  ( 17.17241001986506888, 1518.913060387330006, 238.6251415217915337 ) ) ;
#51700=SURFACE_SIDE_STYLE ('',( #86390 ) ) ;
#51716=( BOUNDED_SURFACE ( )  B_SPLINE_SURFACE ( 3, 2, ( 
 ( #10301, #19803, #87010 ),
 ( #80280, #36614, #36074 ),
 ( #70259, #104367, #28212 ),
 ( #98163, #89222, #45596 ),
 ( #104927, #97084, #12517 ),
 ( #27663, #79738, #3046 ) ),
 .UNSPECIFIED., .F., .F., .T. ) 
 B_SPLINE_SURFACE_WITH_KNOTS ( ( 4, 2, 4 ),
 ( 3, 3 ),
 ( -2.103352214621878602E-17, 0.001312027981647337967, 0.002624055963294697185 ),
 ( 0.000000000000000000, 1.000000000000000000 ),
 .UNSPECIFIED. ) 
 GEOMETRIC_REPRESENTATION_ITEM ( )  RATIONAL_B_SPLINE_SURFACE ( (
 ( 1.000000000000000000, 0.9376006582765896713, 1.000000000000000000),
 ( 1.000000000000000000, 0.9569320108030433536, 1.000000000000000000),
 ( 1.000000000000000000, 0.9725743441608392104, 1.000000000000000000),
 ( 1.000000000000000000, 0.9942095667146111371, 1.000000000000000000),
 ( 1.000000000000000000, 1.000043666449921265, 1.000000000000000000),
 ( 1.000000000000000000, 1.000000000000000000, 1.000000000000000000) ) ) 
 REPRESENTATION_ITEM ( '' )  SURFACE ( )  );
#51731=ORIENTED_EDGE ( 'NONE', *, *, #67624, .F. ) ;
#51745=ORIENTED_EDGE ( 'NONE', *, *, #79451, .F. ) ;
#51763=CARTESIAN_POINT ( 'NONE',  ( 21.91520783698931751, 1524.538768545234007, 184.5727256433340244 ) ) ;
#51784=CIRCLE ( 'NONE', #82134, 33.13701971169416538 ) ;
#51788=DIRECTION ( 'NONE',  ( 0.000000000000000000, 0.000000000000000000, 1.000000000000000000 ) ) ;
#51793=EDGE_CURVE ( 'NONE', #29992, #12956, #2514, .T. ) ;
#51796=ORIENTED_EDGE ( 'NONE', *, *, #91968, .F. ) ;
#51811=EDGE_CURVE ( 'NONE', #41235, #49802, #49426, .T. ) ;
#51826=B_SPLINE_CURVE_WITH_KNOTS ( 'NONE', 3,
 ( #73462, #107593, #4595, #38729 ),
 .UNSPECIFIED., .F., .F.,
 ( 4, 4 ),
 ( 0.000000000000000000, 0.0002960034161023842431 ),
 .UNSPECIFIED. ) ;
#51830=CARTESIAN_POINT ( 'NONE',  ( -2.582675909241389345, 1526.178928173327677, 242.3428666835333445 ) ) ;
#51844=CARTESIAN_POINT ( 'NONE',  ( -32.32093690483954163, 1524.075000532257718, 202.1437793362934485 ) ) ;
#51853=ORIENTED_EDGE ( 'NONE', *, *, #93471, .F. ) ;
#51863=ORIENTED_EDGE ( 'NONE', *, *, #93209, .T. ) ;
#51864=DIRECTION ( 'NONE',  ( -0.9942586961433749204, 0.000000000000000000, 0.1070030146457375819 ) ) ;
#51878=CARTESIAN_POINT ( 'NONE',  ( -31.23437356469455040, 1511.187213306747708, 197.3468678195118287 ) ) ;
#51886=CARTESIAN_POINT ( 'NONE',  ( -29.75840146891882654, 1525.320849883639312, 222.0114828297162717 ) ) ;
#51909=ORIENTED_EDGE ( 'NONE', *, *, #92101, .F. ) ;
#51914=CARTESIAN_POINT ( 'NONE',  ( -31.95643112690961019, 1526.329757971584968, 201.5629546934959251 ) ) ;
#51915=CARTESIAN_POINT ( 'NONE',  ( -21.80961351509205670, 1523.919943579690425, 234.9115559964644149 ) ) ;
#51928=CARTESIAN_POINT ( 'NONE',  ( -2.385019621457261874, 1526.073429442291854, 177.7124997907143040 ) ) ;
#51931=CARTESIAN_POINT ( 'NONE',  ( 28.97303002314154696, 1526.186458717542791, 220.8123550170068654 ) ) ;
#51942=AXIS2_PLACEMENT_3D ( 'NONE', #45850, #36871, #71065 ) ;
#51947=ORIENTED_EDGE ( 'NONE', *, *, #45039, .T. ) ;
#51970=CARTESIAN_POINT ( 'NONE',  ( 2.038847259689231084, 1501.977400791986611, 173.3106345060153046 ) ) ;
#51988=FACE_OUTER_BOUND ( 'NONE', #84873, .T. ) ;
#51993=CARTESIAN_POINT ( 'NONE',  ( -2.485146179491022345, 1524.547395018738143, 175.7094276205802146 ) ) ;
#51997=DIRECTION ( 'NONE',  ( 0.000000000000000000, -0.07593562622321022026, -0.9971127221483482295 ) ) ;
#52015=ADVANCED_FACE ( 'NONE', ( #27138 ), #98492, .T. ) ;
#52037=CARTESIAN_POINT ( 'NONE',  ( 31.25789155968564970, 1523.954914175594922, 196.3501112485169813 ) ) ;
#52045=AXIS2_PLACEMENT_3D ( 'NONE', #46904, #75403, #15452 ) ;
#52063=AXIS2_PLACEMENT_3D ( 'NONE', #65004, #22961, #6727 ) ;
#52077=VECTOR ( 'NONE', #44348, 999.9999999999998863 ) ;
#52098=CIRCLE ( 'NONE', #19941, 0.9999999999999952260 ) ;
#52106=DIRECTION ( 'NONE',  ( 0.000000000000000000, -0.8724564897876576630, -0.4886917979948086077 ) ) ;
#52115=EDGE_CURVE ( 'NONE', #109511, #95178, #44907, .T. ) ;
#52118=EDGE_CURVE ( 'NONE', #2574, #31132, #50250, .T. ) ;
#52119=CARTESIAN_POINT ( 'NONE',  ( -31.29224604902359985, 1525.661275128775969, 216.2849134033308758 ) ) ;
#52147=DIRECTION ( 'NONE',  ( 0.8090169943749465631, 0.000000000000000000, -0.5877852522924742473 ) ) ;
#52152=CARTESIAN_POINT ( 'NONE',  ( 30.25425994617009096, 1526.382868172863937, 218.9520509131588994 ) ) ;
#52153=EDGE_CURVE ( 'NONE', #23737, #83466, #18085, .T. ) ;
#52155=DIRECTION ( 'NONE',  ( -0.9125304618753966590, 0.000000000000000000, 0.4090087482554319309 ) ) ;
#52169=( BOUNDED_SURFACE ( )  B_SPLINE_SURFACE ( 3, 2, ( 
 ( #38676, #30827, #63913 ),
 ( #3460, #98029, #39226 ),
 ( #105909, #55505, #89634 ),
 ( #65003, #81773, #12921 ),
 ( #54962, #108082, #31377 ),
 ( #37587, #63379, #47101 ),
 ( #89089, #97495, #20763 ),
 ( #90732, #57168, #56598 ),
 ( #81227, #30274, #12376 ),
 ( #4007, #38132, #4542 ) ),
 .UNSPECIFIED., .F., .F., .F. ) 
 B_SPLINE_SURFACE_WITH_KNOTS ( ( 4, 2, 2, 2, 4 ),
 ( 3, 3 ),
 ( 0.000000000000000000, 0.3926990816987241395, 0.7853981633974482790, 1.178097245096172418, 1.570796326794896558 ),
 ( 0.000000000000000000, 1.000000000000000000 ),
 .UNSPECIFIED. ) 
 GEOMETRIC_REPRESENTATION_ITEM ( )  RATIONAL_B_SPLINE_SURFACE ( (
 ( 1.000000000000000000, 0.7763623250684332788, 1.000000000000000000),
 ( 1.000000000000000000, 0.7763684247032729413, 1.000000000000000000),
 ( 1.000000000000000000, 0.7746454561800525385, 1.000000000000000000),
 ( 1.000000000000000000, 0.7679730451969956073, 1.000000000000000000),
 ( 1.000000000000000000, 0.7630177051944824207, 1.000000000000000000),
 ( 1.000000000000000000, 0.7504512394530151731, 1.000000000000000000),
 ( 1.000000000000000000, 0.7428408967932995655, 1.000000000000000000),
 ( 1.000000000000000000, 0.7259222650904413321, 1.000000000000000000),
 ( 1.000000000000000000, 0.7166207884824116192, 1.000000000000000000),
 ( 1.000000000000000000, 0.7071067811865867636, 1.000000000000000000) ) ) 
 REPRESENTATION_ITEM ( '' )  SURFACE ( )  );
#52194=DIRECTION ( 'NONE',  ( 0.4978433412588811335, 0.000000000000000000, 0.8672669759446587356 ) ) ;
#52202=EDGE_CURVE ( 'NONE', #90117, #71856, #37765, .T. ) ;
#52210=EDGE_CURVE ( 'NONE', #43597, #9501, #29170, .T. ) ;
#52214=CARTESIAN_POINT ( 'NONE',  ( 17.22845782853287488, 1525.848196786131211, 236.4819750992561467 ) ) ;
#52229=CARTESIAN_POINT ( 'NONE',  ( -30.29139560038384360, 1523.843271061948826, 195.7510757303778064 ) ) ;
#52230=CARTESIAN_POINT ( 'NONE',  ( 32.86802468386284914, 1523.481610426287716, 201.0396662540042030 ) ) ;
#52234=CARTESIAN_POINT ( 'NONE',  ( -0.4151546846821903003, 1522.382868172863937, 242.9330574173806951 ) ) ;
#52243=CARTESIAN_POINT ( 'NONE',  ( -156.6846457583342840, 1524.382868172863937, 340.9912860285748479 ) ) ;
#52265=AXIS2_PLACEMENT_3D ( 'NONE', #50259, #18267, #59209 ) ;
#52269=VERTEX_POINT ( 'NONE', #52628 ) ;
#52281=DIRECTION ( 'NONE',  ( 0.000000000000000000, 0.000000000000000000, 1.000000000000000000 ) ) ;
#52293=ORIENTED_EDGE ( 'NONE', *, *, #37818, .T. ) ;
#52305=ORIENTED_EDGE ( 'NONE', *, *, #100694, .T. ) ;
#52318=CARTESIAN_POINT ( 'NONE',  ( -2.407253779970412566, 1523.313115944345554, 175.0653106450178882 ) ) ;
#52322=CARTESIAN_POINT ( 'NONE',  ( 21.38516915557964282, 1522.382868172863937, 180.3939891059721106 ) ) ;
#52349=AXIS2_PLACEMENT_3D ( 'NONE', #6596, #91700, #15522 ) ;
#52350=CARTESIAN_POINT ( 'NONE',  ( 28.62254820377552278, 1526.345556099435726, 198.0531334975491973 ) ) ;
#52354=CARTESIAN_POINT ( 'NONE',  ( 22.75273496409577945, 1518.913060387330006, 183.6728937936772184 ) ) ;
#52371=CARTESIAN_POINT ( 'NONE',  ( -33.82780500856058836, 1523.429859730330463, 197.6825146852533237 ) ) ;
#52374=CARTESIAN_POINT ( 'NONE',  ( -31.23437356469425907, 1512.187213306747481, 222.8968241038848248 ) ) ;
#52380=ORIENTED_EDGE ( 'NONE', *, *, #9651, .F. ) ;
#52381=( BOUNDED_SURFACE ( )  B_SPLINE_SURFACE ( 3, 2, ( 
 ( #72807, #45951, #97445 ),
 ( #98534, #71741, #89033 ),
 ( #106396, #64959, #21245 ),
 ( #12323, #46512, #89586 ),
 ( #106935, #108033, #22352 ),
 ( #90682, #30223, #21802 ) ),
 .UNSPECIFIED., .F., .F., .T. ) 
 B_SPLINE_SURFACE_WITH_KNOTS ( ( 4, 2, 4 ),
 ( 3, 3 ),
 ( -6.440160904563896338E-17, 0.001312027981647337100, 0.002624055963294738385 ),
 ( 0.000000000000000000, 1.000000000000000000 ),
 .UNSPECIFIED. ) 
 GEOMETRIC_REPRESENTATION_ITEM ( )  RATIONAL_B_SPLINE_SURFACE ( (
 ( 1.000000000000000000, 0.9376006582765872288, 1.000000000000000000),
 ( 1.000000000000000000, 0.9569320108031740268, 1.000000000000000000),
 ( 1.000000000000000000, 0.9725743441606660156, 1.000000000000000000),
 ( 1.000000000000000000, 0.9942095667147807792, 1.000000000000000000),
 ( 1.000000000000000000, 1.000043666449794921, 1.000000000000000000),
 ( 1.000000000000000000, 1.000000000000000000, 1.000000000000000000) ) ) 
 REPRESENTATION_ITEM ( '' )  SURFACE ( )  );
#52382=CARTESIAN_POINT ( 'NONE',  ( 30.31940284292409515, 1523.382868172864164, 195.7503880523414352 ) ) ;
#52401=CARTESIAN_POINT ( 'NONE',  ( 19.53786426059039982, 1512.187213306747481, 236.7197124308265188 ) ) ;
#52407=CARTESIAN_POINT ( 'NONE',  ( -49.24962907673571522, 1524.382868172863937, 407.9033880519289710 ) ) ;
#52418=CARTESIAN_POINT ( 'NONE',  ( -22.75273496409559826, 1512.187213306747481, 234.5707981297189235 ) ) ;
#52427=ADVANCED_FACE ( 'NONE', ( #7173 ), #29769, .T. ) ;
#52429=EDGE_CURVE ( 'NONE', #108583, #101705, #91469, .T. ) ;
#52438=LINE ( 'NONE', #24981, #9116 ) ;
#52469=ORIENTED_EDGE ( 'NONE', *, *, #93178, .F. ) ;
#52472=EDGE_CURVE ( 'NONE', #38412, #91781, #27135, .T. ) ;
#52475=CARTESIAN_POINT ( 'NONE',  ( -29.30029655192939586, 1525.907212628473872, 196.8717316207790589 ) ) ;
#52505=ORIENTED_EDGE ( 'NONE', *, *, #63780, .F. ) ;
#52521=DIRECTION ( 'NONE',  ( 0.4978433412588638141, 0.000000000000000000, -0.8672669759446687276 ) ) ;
#52529=FACE_OUTER_BOUND ( 'NONE', #56396, .T. ) ;
#52531=CARTESIAN_POINT ( 'NONE',  ( -28.27139721233033143, 1526.382868172863937, 219.5606225550389752 ) ) ;
#52537=ORIENTED_EDGE ( 'NONE', *, *, #84884, .T. ) ;
#52539=CIRCLE ( 'NONE', #109743, 0.9999999999999952260 ) ;
#52545=AXIS2_PLACEMENT_3D ( 'NONE', #37696, #3024, #89747 ) ;
#52559=AXIS2_PLACEMENT_3D ( 'NONE', #100594, #40700, #23875 ) ;
#52568=DIRECTION ( 'NONE',  ( 0.000000000000000000, -1.000000000000000000, 0.000000000000000000 ) ) ;
#52579=B_SPLINE_CURVE_WITH_KNOTS ( 'NONE', 3,
 ( #44701, #104587, #78850, #70466 ),
 .UNSPECIFIED., .F., .F.,
 ( 4, 4 ),
 ( 0.000000000000000000, 0.0002960034161023844057 ),
 .UNSPECIFIED. ) ;
#52585=DIRECTION ( 'NONE',  ( 0.000000000000000000, 1.000000000000000000, 0.000000000000000000 ) ) ;
#52606=CARTESIAN_POINT ( 'NONE',  ( -28.44698416550318498, 1526.373507135059299, 198.3684985826631930 ) ) ;
#52615=CARTESIAN_POINT ( 'NONE',  ( 33.28034951413933129, 1522.382868172863937, 217.4407153818819722 ) ) ;
#52628=CARTESIAN_POINT ( 'NONE',  ( 20.49599333844834348, 1525.960063244517187, 184.3798832129035077 ) ) ;
#52641=DIRECTION ( 'NONE',  ( 0.000000000000000000, 1.000000000000000000, 0.000000000000000000 ) ) ;
#52657=CARTESIAN_POINT ( 'NONE',  ( -29.78220350812331674, 1526.382868172863937, 221.7347658002328501 ) ) ;
#52663=CARTESIAN_POINT ( 'NONE',  ( -30.25425994616995240, 1526.382868172863937, 218.9520509131593258 ) ) ;
#52667=LINE ( 'NONE', #89002, #60812 ) ;
#52669=CARTESIAN_POINT ( 'NONE',  ( -30.90487439922522483, 1525.907212628473872, 216.4335774778785151 ) ) ;
#52681=CARTESIAN_POINT ( 'NONE',  ( -17.84338787571961049, 1523.382868172864164, 180.3600277896300383 ) ) ;
#52685=LINE ( 'NONE', #59990, #92049 ) ;
#52694=ORIENTED_EDGE ( 'NONE', *, *, #91235, .T. ) ;
#52714=CYLINDRICAL_SURFACE ( 'NONE', #103582, 1.999999999999995559 ) ;
#52717=CARTESIAN_POINT ( 'NONE',  ( 17.17241001986506888, 1512.187213306747481, 237.6251415217915337 ) ) ;
#52721=CARTESIAN_POINT ( 'NONE',  ( 32.38601544705589674, 1523.530935881284904, 216.1237228173871472 ) ) ;
#52734=CARTESIAN_POINT ( 'NONE',  ( -21.37469332459370008, 1525.408327360777776, 233.4084527748692892 ) ) ;
#52735=AXIS2_PLACEMENT_3D ( 'NONE', #108152, #31441, #102490 ) ;
#52739=ORIENTED_EDGE ( 'NONE', *, *, #15689, .T. ) ;
#52754=CARTESIAN_POINT ( 'NONE',  ( -34.31402925621615196, 1524.244163922423695, 218.0340858097422085 ) ) ;
#52774=CARTESIAN_POINT ( 'NONE',  ( -30.44070839969640829, 1525.425665131968344, 196.7701875139011634 ) ) ;
#52798=CARTESIAN_POINT ( 'NONE',  ( 19.39983987834424539, 1522.861859112239017, 239.2921289694150460 ) ) ;
#52818=CARTESIAN_POINT ( 'NONE',  ( 22.07691418024165486, 1523.843271061949054, 184.4448120176447503 ) ) ;
#52819=ORIENTED_EDGE ( 'NONE', *, *, #28685, .F. ) ;
#52840=ORIENTED_EDGE ( 'NONE', *, *, #1710, .F. ) ;
#52841=ORIENTED_EDGE ( 'NONE', *, *, #73472, .F. ) ;
#52857=B_SPLINE_CURVE_WITH_KNOTS ( 'NONE', 3,
 ( #101157, #6018, #100614, #65400 ),
 .UNSPECIFIED., .F., .F.,
 ( 4, 4 ),
 ( 0.000000000000000000, 0.0002960034161023850563 ),
 .UNSPECIFIED. ) ;
#52868=CARTESIAN_POINT ( 'NONE',  ( 20.38673671613194216, 1525.878013734320803, 182.1228282333742072 ) ) ;
#52878=CARTESIAN_POINT ( 'NONE',  ( 31.16641183314581554, 1524.201816949777367, 221.8713787598176737 ) ) ;
#52899=DIRECTION ( 'NONE',  ( -2.664535259100376091E-15, 0.000000000000000000, -1.000000000000000000 ) ) ;
#52900=CARTESIAN_POINT ( 'NONE',  ( -18.66420869458026388, 1526.382868172863937, 232.7837831374280881 ) ) ;
#52905=FACE_OUTER_BOUND ( 'NONE', #81528, .T. ) ;
#52909=ORIENTED_EDGE ( 'NONE', *, *, #50445, .T. ) ;
#52910=CARTESIAN_POINT ( 'NONE',  ( 20.70484064406359437, 1525.907212628473872, 185.0411015109854134 ) ) ;
#52911=CARTESIAN_POINT ( 'NONE',  ( -22.08622291482367217, 1523.456872492435195, 184.4183880513178053 ) ) ;
#52915=CARTESIAN_POINT ( 'NONE',  ( -33.42844755917201383, 1522.382868172863709, 196.1165140606795489 ) ) ;
#52921=EDGE_CURVE ( 'NONE', #83491, #17784, #86677, .T. ) ;
#52925=EDGE_CURVE ( 'NONE', #22416, #31153, #46596, .T. ) ;
#52928=FACE_OUTER_BOUND ( 'NONE', #3001, .T. ) ;
#52930=CARTESIAN_POINT ( 'NONE',  ( -21.83550407203883736, 1523.678648413191695, 234.9693198511254195 ) ) ;
#52948=CARTESIAN_POINT ( 'NONE',  ( 32.28466283162151029, 1512.187213306747481, 199.0684425896244250 ) ) ;
#52970=EDGE_CURVE ( 'NONE', #21237, #967, #50448, .T. ) ;
#53013=ADVANCED_FACE ( 'NONE', ( #56443 ), #73239, .T. ) ;
#53026=CARTESIAN_POINT ( 'NONE',  ( -32.77044109517588311, 1525.581535527370306, 199.0807904155091990 ) ) ;
#53030=CARTESIAN_POINT ( 'NONE',  ( 32.66476241579314177, 1526.382868172863937, 199.1278258474837060 ) ) ;
#53041=CARTESIAN_POINT ( 'NONE',  ( 30.90487439922560498, 1525.907212628473644, 216.4335774778780035 ) ) ;
#53043=CARTESIAN_POINT ( 'NONE',  ( 29.86461515634911024, 1525.960063244517187, 220.9690070206020778 ) ) ;
#53046=CIRCLE ( 'NONE', #47681, 1.999999999999998668 ) ;
#53050=CARTESIAN_POINT ( 'NONE',  ( 3.448830483803564828, 1512.187213306747481, 243.0842028158767789 ) ) ;
#53053=ORIENTED_EDGE ( 'NONE', *, *, #19333, .F. ) ;
#53067=EDGE_CURVE ( 'NONE', #43885, #101252, #27067, .T. ) ;
#53078=ORIENTED_EDGE ( 'NONE', *, *, #89051, .F. ) ;
#53093=ORIENTED_EDGE ( 'NONE', *, *, #72638, .F. ) ;
#53102=DIRECTION ( 'NONE',  ( -4.857225732735055447E-14, 0.000000000000000000, 1.000000000000000000 ) ) ;
#53106=DIRECTION ( 'NONE',  ( 0.9125304618754024322, 0.000000000000000000, 0.4090087482554191078 ) ) ;
#53119=ORIENTED_EDGE ( 'NONE', *, *, #73891, .F. ) ;
#53122=CARTESIAN_POINT ( 'NONE',  ( 31.23437356469446868, 1512.187213306747481, 222.8968241038843701 ) ) ;
#53147=AXIS2_PLACEMENT_3D ( 'NONE', #11289, #104231, #79054 ) ;
#53151=CARTESIAN_POINT ( 'NONE',  ( 3.351183042480982976, 1524.075000532256581, 242.0172247929413629 ) ) ;
#53154=CARTESIAN_POINT ( 'NONE',  ( 21.38516915558662035, 1522.906561336852974, 237.8497028174188586 ) ) ;
#53156=CARTESIAN_POINT ( 'NONE',  ( 33.93019615848946557, 1522.382868172863937, 197.6607374645996060 ) ) ;
#53157=FACE_OUTER_BOUND ( 'NONE', #53959, .T. ) ;
#53167=AXIS2_PLACEMENT_3D ( 'NONE', #100089, #96939, #71773 ) ;
#53168=DIRECTION ( 'NONE',  ( 0.000000000000000000, 0.000000000000000000, 1.000000000000000000 ) ) ;
#53169=CARTESIAN_POINT ( 'NONE',  ( -2.273033093151333617, 1525.821544997590763, 240.9339456143065092 ) ) ;
#53174=CARTESIAN_POINT ( 'NONE',  ( 30.51231035492521571, 1524.382868172863937, 218.1578534183718432 ) ) ;
#53186=CARTESIAN_POINT ( 'NONE',  ( 32.02808312589922224, 1512.187213306747481, 219.9649204700462235 ) ) ;
#53189=EDGE_LOOP ( 'NONE', ( #78593, #109434, #17073, #41854 ) ) ;
#53197=AXIS2_PLACEMENT_3D ( 'NONE', #66530, #23920, #91695 ) ;
#53202=CARTESIAN_POINT ( 'NONE',  ( -32.85805783624314813, 1523.678648413191695, 201.0453875934059340 ) ) ;
#53205=ADVANCED_FACE ( 'NONE', ( #46956 ), #57597, .F. ) ;
#53206=DIRECTION ( 'NONE',  ( 0.000000000000000000, 0.000000000000000000, 1.000000000000000000 ) ) ;
#53210=LINE ( 'NONE', #85678, #80169 ) ;
#53225=AXIS2_PLACEMENT_3D ( 'NONE', #69716, #34967, #51788 ) ;
#53230=ORIENTED_EDGE ( 'NONE', *, *, #88332, .T. ) ;
#53231=FACE_OUTER_BOUND ( 'NONE', #99987, .T. ) ;
#53250=ORIENTED_EDGE ( 'NONE', *, *, #1467, .F. ) ;
#53252=CIRCLE ( 'NONE', #74746, 33.13701971169416538 ) ;
#53272=ORIENTED_EDGE ( 'NONE', *, *, #97593, .T. ) ;
#53292=CARTESIAN_POINT ( 'NONE',  ( -3.451191875628176753, 1523.678648413191695, 175.1707361340005207 ) ) ;
#53313=CARTESIAN_POINT ( 'NONE',  ( -30.51231035492510557, 1526.382868172863937, 218.1578534183722979 ) ) ;
#53326=ORIENTED_EDGE ( 'NONE', *, *, #24716, .F. ) ;
#53347=CARTESIAN_POINT ( 'NONE',  ( 19.53786426059019021, 1512.187213306747481, 180.5239794925693388 ) ) ;
#53350=CARTESIAN_POINT ( 'NONE',  ( -16.16632277704816900, 1512.187213306747481, 181.3470724465437627 ) ) ;
#53366=DIRECTION ( 'NONE',  ( -0.5877852522924820189, 0.000000000000000000, -0.8090169943749410120 ) ) ;
#53367=( NAMED_UNIT ( * ) SI_UNIT ( $, .STERADIAN. ) SOLID_ANGLE_UNIT ( ) );
#53373=CARTESIAN_POINT ( 'NONE',  ( 21.08704007906474942, 1525.317349363550420, 184.4717524171098546 ) ) ;
#53391=VERTEX_POINT ( 'NONE', #76955 ) ;
#53418=CARTESIAN_POINT ( 'NONE',  ( -0.8350686643532190256, 1526.382868172863937, 240.9330574173806951 ) ) ;
#53424=CARTESIAN_POINT ( 'NONE',  ( -31.41104781486814090, 1511.187213306747708, 215.9140555522426723 ) ) ;
#53426=VECTOR ( 'NONE', #48885, 1000.000000000000114 ) ;
#53428=EDGE_CURVE ( 'NONE', #101252, #101260, #43358, .T. ) ;
#53430=EDGE_CURVE ( 'NONE', #5750, #39868, #42242, .T. ) ;
#53436=B_SPLINE_CURVE_WITH_KNOTS ( 'NONE', 3,
 ( #77511, #103229, #26539, #27655, #61841, #19222, #87576, #55086, #108210, #14143 ),
 .UNSPECIFIED., .F., .F.,
 ( 4, 2, 2, 2, 4 ),
 ( 3.925231146709437917E-17, 0.0007406479101619153297, 0.001481295820323791411, 0.002221943730485667710, 0.002962591640647543791 ),
 .UNSPECIFIED. ) ;
#53455=ADVANCED_FACE ( 'NONE', ( #84774 ), #75575, .T. ) ;
#53464=ORIENTED_EDGE ( 'NONE', *, *, #107488, .F. ) ;
#53498=CIRCLE ( 'NONE', #5201, 30.13701971169416183 ) ;
#53502=ORIENTED_EDGE ( 'NONE', *, *, #86300, .F. ) ;
#53512=DIRECTION ( 'NONE',  ( 0.7454942576402798782, 5.172905559738552453E-15, 0.6665120492724555534 ) ) ;
#53518=VERTEX_POINT ( 'NONE', #53418 ) ;
#53537=CARTESIAN_POINT ( 'NONE',  ( -28.27139721233033143, 1526.382868172863937, 219.5606225550389752 ) ) ;
#53550=CIRCLE ( 'NONE', #19539, 2.000000000000001776 ) ;
#53563=CARTESIAN_POINT ( 'NONE',  ( 22.08622291488258327, 1523.456924617339155, 233.8253038720255574 ) ) ;
#53566=PRODUCT_DEFINITION_SHAPE ( 'NONE', 'NONE',  #21967 ) ;
#53570=DIRECTION ( 'NONE',  ( 0.000000000000000000, 0.000000000000000000, -1.000000000000000000 ) ) ;
#53579=CARTESIAN_POINT ( 'NONE',  ( -20.49599333844893678, 1525.960063244516959, 184.3798832129038203 ) ) ;
#53601=ADVANCED_FACE ( 'NONE', ( #91808 ), #38274, .F. ) ;
#53608=CARTESIAN_POINT ( 'NONE',  ( 29.36007807473284359, 1526.208281990542673, 220.5288989449384189 ) ) ;
#53618=ORIENTED_EDGE ( 'NONE', *, *, #35110, .F. ) ;
#53648=CIRCLE ( 'NONE', #82216, 1.000000000000000000 ) ;
#53657=AXIS2_PLACEMENT_3D ( 'NONE', #47045, #38615, #28018 ) ;
#53667=DIRECTION ( 'NONE',  ( -0.000000000000000000, -1.000000000000000000, -0.000000000000000000 ) ) ;
#53670=CARTESIAN_POINT ( 'NONE',  ( -2.494564929293782818, 1524.201670966335769, 175.5409631904079788 ) ) ;
#53671=CARTESIAN_POINT ( 'NONE',  ( -29.36007807473230713, 1526.208281990539035, 197.7147929784467806 ) ) ;
#53691=AXIS2_PLACEMENT_3D ( 'NONE', #34861, #23695, #100946 ) ;
#53700=ORIENTED_EDGE ( 'NONE', *, *, #54340, .F. ) ;
#53706=EDGE_CURVE ( 'NONE', #9501, #68723, #27927, .T. ) ;
#53710=ADVANCED_FACE ( 'NONE', ( #4780 ), #75344, .T. ) ;
#53722=ORIENTED_EDGE ( 'NONE', *, *, #65817, .F. ) ;
#53723=DIRECTION ( 'NONE',  ( -0.2054769195713318786, 0.000000000000000000, 0.9786619618251628516 ) ) ;
#53724=CARTESIAN_POINT ( 'NONE',  ( 22.66254714602126441, 1523.342713519622748, 236.8145175431291989 ) ) ;
#53729=CARTESIAN_POINT ( 'NONE',  ( -32.86802468386279941, 1501.977400791986611, 217.2040256693919957 ) ) ;
#53740=EDGE_CURVE ( 'NONE', #100597, #23737, #75425, .T. ) ;
#53746=EDGE_CURVE ( 'NONE', #15491, #90688, #74226, .T. ) ;
#53761=CARTESIAN_POINT ( 'NONE',  ( -32.35345263957390216, 1524.872178180564333, 217.0491086732562280 ) ) ;
#53766=DIRECTION ( 'NONE',  ( 0.000000000000000000, 1.000000000000000000, 0.000000000000000000 ) ) ;
#53767=CARTESIAN_POINT ( 'NONE',  ( -16.66231036550682987, 1523.604703353109699, 237.7554842931448036 ) ) ;
#53774=LINE ( 'NONE', #11736, #37205 ) ;
#53780=VERTEX_POINT ( 'NONE', #109467 ) ;
#53796=CARTESIAN_POINT ( 'NONE',  ( 22.08327125186944428, 1523.604703353109699, 233.8169256665487694 ) ) ;
#53799=VERTEX_POINT ( 'NONE', #32745 ) ;
#53830=ORIENTED_EDGE ( 'NONE', *, *, #35983, .F. ) ;
#53837=ORIENTED_EDGE ( 'NONE', *, *, #20664, .F. ) ;
#53862=CARTESIAN_POINT ( 'NONE',  ( -16.87900699709440033, 1524.382868172804365, 181.2327155136482020 ) ) ;
#53878=B_SPLINE_CURVE_WITH_KNOTS ( 'NONE', 3,
 ( #71192, #52721, #11271, #78465 ),
 .UNSPECIFIED., .F., .F.,
 ( 4, 4 ),
 ( 0.000000000000000000, 0.0002220129587134773411 ),
 .UNSPECIFIED. ) ;
#53902=CARTESIAN_POINT ( 'NONE',  ( 33.82780500856040362, 1523.429859730330463, 197.6825146852528974 ) ) ;
#53904=DIRECTION ( 'NONE',  ( 0.000000000000000000, 0.000000000000000000, 1.000000000000000000 ) ) ;
#53906=CARTESIAN_POINT ( 'NONE',  ( -30.25946001110623129, 1524.776010967693765, 196.4597699223641314 ) ) ;
#53908=CARTESIAN_POINT ( 'NONE',  ( 18.98249322453000332, 1526.382868172864164, 232.9711420821685692 ) ) ;
#53959=EDGE_LOOP ( 'NONE', ( #17205, #109508, #83375, #44297 ) ) ;
#53961=DIRECTION ( 'NONE',  ( -0.1070030146457386366, 0.000000000000000000, -0.9942586961433749204 ) ) ;
#53965=DIRECTION ( 'NONE',  ( 0.1070030146457317810, 0.000000000000000000, -0.9942586961433755866 ) ) ;
#53998=DIRECTION ( 'NONE',  ( 0.1010290445074205484, 0.000000000000000000, 0.9948834766775040972 ) ) ;
#54004=ORIENTED_EDGE ( 'NONE', *, *, #53067, .F. ) ;
#54005=CARTESIAN_POINT ( 'NONE',  ( -17.19739463999614060, 1525.960063244517187, 236.2603809477411119 ) ) ;
#54017=ORIENTED_EDGE ( 'NONE', *, *, #107194, .F. ) ;
#54025=CIRCLE ( 'NONE', #68316, 1.000000000000001332 ) ;
#54028=CARTESIAN_POINT ( 'NONE',  ( -30.31940284292398857, 1523.382868172864164, 222.4933038710547919 ) ) ;
#54029=DIRECTION ( 'NONE',  ( 0.000000000000000000, 0.000000000000000000, -1.000000000000000000 ) ) ;
#54031=CARTESIAN_POINT ( 'NONE',  ( -21.53712143570596638, 1523.621879633029039, 183.9400870382965820 ) ) ;
#54033=ORIENTED_EDGE ( 'NONE', *, *, #100830, .T. ) ;
#54047=AXIS2_PLACEMENT_3D ( 'NONE', #4858, #89969, #73180 ) ;
#54071=DIRECTION ( 'NONE',  ( -0.3090169943749383474, 0.000000000000000000, 0.9510565162951566398 ) ) ;
#54078=ADVANCED_FACE ( 'NONE', ( #85908 ), #17009, .T. ) ;
#54086=DIRECTION ( 'NONE',  ( 0.000000000000000000, 0.000000000000000000, -1.000000000000000000 ) ) ;
#54087=CARTESIAN_POINT ( 'NONE',  ( 20.72500163403594797, 1525.697946996619521, 233.5887219448511303 ) ) ;
#54133=ORIENTED_EDGE ( 'NONE', *, *, #65951, .F. ) ;
#54146=DIRECTION ( 'NONE',  ( -0.000000000000000000, -1.000000000000000000, -0.000000000000000000 ) ) ;
#54150=CARTESIAN_POINT ( 'NONE',  ( 2.057041824812614106, 1523.342713519622521, 244.8463988825301385 ) ) ;
#54158=CARTESIAN_POINT ( 'NONE',  ( 1.191524307911315805, 1526.382868172863937, 239.2353018730792087 ) ) ;
#54159=CARTESIAN_POINT ( 'NONE',  ( -2.273033093151334061, 1525.821544997590763, 240.9339456143064808 ) ) ;
#54176=CARTESIAN_POINT ( 'NONE',  ( 31.32995031131198616, 1523.678648413191695, 221.9013357025044115 ) ) ;
#54192=DIRECTION ( 'NONE',  ( 0.000000000000000000, 0.000000000000000000, 1.000000000000000000 ) ) ;
#54202=EDGE_CURVE ( 'NONE', #4434, #69831, #31731, .T. ) ;
#54211=ORIENTED_EDGE ( 'NONE', *, *, #6871, .F. ) ;
#54220=ORIENTED_EDGE ( 'NONE', *, *, #30691, .F. ) ;
#54225=EDGE_CURVE ( 'NONE', #64661, #5750, #50402, .T. ) ;
#54231=CYLINDRICAL_SURFACE ( 'NONE', #46530, 23.69926344187880929 ) ;
#54235=EDGE_CURVE ( 'NONE', #73756, #103878, #48340, .T. ) ;
#54267=CARTESIAN_POINT ( 'NONE',  ( 21.92916355573715492, 1523.390106123591067, 235.1782814742748258 ) ) ;
#54275=CARTESIAN_POINT ( 'NONE',  ( -29.13504683812242035, 1526.073434386619283, 197.1475439643201355 ) ) ;
#54276=CARTESIAN_POINT ( 'NONE',  ( -31.22294729666610280, 1523.678648413191695, 222.8955943986482282 ) ) ;
#54282=LINE ( 'NONE', #54825, #98419 ) ;
#54290=CARTESIAN_POINT ( 'NONE',  ( -17.19739463999618678, 1525.960063244516959, 236.2603809477411971 ) ) ;
#54310=CIRCLE ( 'NONE', #6001, 29.51505616007316135 ) ;
#54321=VERTEX_POINT ( 'NONE', #9609 ) ;
#54323=( BOUNDED_CURVE ( )  B_SPLINE_CURVE ( 3, ( #33458, #58150, #98057, #66013 ),
 .UNSPECIFIED., .F., .F. ) 
 B_SPLINE_CURVE_WITH_KNOTS ( ( 4, 4 ),
 ( 2.436781329611978464, 3.141592653589793116 ),
 .UNSPECIFIED. ) 
 CURVE ( )  GEOMETRIC_REPRESENTATION_ITEM ( )  RATIONAL_B_SPLINE_CURVE ( ( 1.000000000000000000, 0.9590300661663082593, 0.9590300661663082593, 1.000000000000000000 ) ) 
 REPRESENTATION_ITEM ( '' )  );
#54330=CARTESIAN_POINT ( 'NONE',  ( 31.56779946216476418, 1525.408327360769590, 202.0372978226081102 ) ) ;
#54340=EDGE_CURVE ( 'NONE', #11785, #66900, #43282, .T. ) ;
#54347=CARTESIAN_POINT ( 'NONE',  ( -19.53786426058999481, 1512.187213306747481, 236.7197124308268030 ) ) ;
#54357=EDGE_CURVE ( 'NONE', #8168, #12203, #17435, .T. ) ;
#54392=CIRCLE ( 'NONE', #95449, 23.69926344187880929 ) ;
#54432=CARTESIAN_POINT ( 'NONE',  ( -32.38845791999504797, 1518.913060387330006, 202.1182848005516348 ) ) ;
#54450=CARTESIAN_POINT ( 'NONE',  ( 20.70484064406395674, 1525.907212628473644, 233.2025904124104443 ) ) ;
#54476=AXIS2_PLACEMENT_3D ( 'NONE', #45103, #55704, #89825 ) ;
#54484=AXIS2_PLACEMENT_3D ( 'NONE', #45759, #37337, #989 ) ;
#54503=DIRECTION ( 'NONE',  ( 0.9983395709201744461, 0.05760296116452706672, 0.000000000000000000 ) ) ;
#54515=AXIS2_PLACEMENT_3D ( 'NONE', #95484, #12030, #80345 ) ;
#54525=ORIENTED_EDGE ( 'NONE', *, *, #55623, .F. ) ;
#54536=CARTESIAN_POINT ( 'NONE',  ( -2.472529913803023227, 1523.678648413191695, 175.3762130535718597 ) ) ;
#54543=CARTESIAN_POINT ( 'NONE',  ( -32.39779788405879657, 1524.816846803860926, 217.0524034676090537 ) ) ;
#54548=CARTESIAN_POINT ( 'NONE',  ( -34.68852446352935459, 1501.977400791986611, 218.2490599186011764 ) ) ;
#54567=VECTOR ( 'NONE', #107405, 1000.000000000000227 ) ;
#54573=DIRECTION ( 'NONE',  ( 0.000000000000000000, 1.000000000000000000, 0.000000000000000000 ) ) ;
#54582=CARTESIAN_POINT ( 'NONE',  ( -30.80549360313099072, 1524.130440953581001, 196.3987987232749219 ) ) ;
#54592=EDGE_CURVE ( 'NONE', #71185, #64042, #9302, .T. ) ;
#54596=CIRCLE ( 'NONE', #2719, 1.000000000000000888 ) ;
#54621=ADVANCED_FACE ( 'NONE', ( #58247 ), #100238, .T. ) ;
#54623=DIRECTION ( 'NONE',  ( -0.6709778558543766369, 0.000000000000000000, -0.7414773880254632576 ) ) ;
#54630=CARTESIAN_POINT ( 'NONE',  ( 21.35005939118691032, 1525.163457223744672, 234.4064223797113868 ) ) ;
#54635=CARTESIAN_POINT ( 'NONE',  ( 32.38114538885255200, 1523.604703353109699, 216.1203639561429100 ) ) ;
#54639=VERTEX_POINT ( 'NONE', #5069 ) ;
#54652=ORIENTED_EDGE ( 'NONE', *, *, #110431, .F. ) ;
#54686=ORIENTED_EDGE ( 'NONE', *, *, #20041, .F. ) ;
#54687=DIRECTION ( 'NONE',  ( 0.1010290445074209786, 0.000000000000000000, 0.9948834766775040972 ) ) ;
#54698=CYLINDRICAL_SURFACE ( 'NONE', #19675, 4.000000000000007994 ) ;
#54700=CARTESIAN_POINT ( 'NONE',  ( 2.425477467415915189, 1523.390106123591067, 243.0915840373823471 ) ) ;
#54701=VERTEX_POINT ( 'NONE', #32489 ) ;
#54704=CARTESIAN_POINT ( 'NONE',  ( -3.448830483803564828, 1512.187213306747481, 243.0842028158767789 ) ) ;
#54707=CARTESIAN_POINT ( 'NONE',  ( 29.00779973304137371, 1526.382868172863937, 217.2942086403122914 ) ) ;
#54724=VERTEX_POINT ( 'NONE', #15642 ) ;
#54730=LINE ( 'NONE', #12142, #41163 ) ;
#54767=ORIENTED_EDGE ( 'NONE', *, *, #1464, .T. ) ;
#54801=CARTESIAN_POINT ( 'NONE',  ( 2.692976938448822466, 1524.059547553519224, 242.0866667222398121 ) ) ;
#54806=TOROIDAL_SURFACE ( 'NONE', #6508, 1.000000000000000000, 1.000000000000000000 ) ;
#54811=EDGE_CURVE ( 'NONE', #8029, #41235, #37932, .T. ) ;
#54820=EDGE_CURVE ( 'NONE', #14716, #13288, #89785, .T. ) ;
#54825=CARTESIAN_POINT ( 'NONE',  ( -18.19590854888185660, 1512.187213306747481, 180.0410247165186490 ) ) ;
#54869=CARTESIAN_POINT ( 'NONE',  ( -29.99620953741478502, 1526.382868172863937, 219.7462484079463252 ) ) ;
#54871=CARTESIAN_POINT ( 'NONE',  ( 31.31962989724480551, 1525.556089352344543, 201.5436831772797746 ) ) ;
#54877=CARTESIAN_POINT ( 'NONE',  ( -2.485517042439642221, 1524.599984580802357, 175.7312637537736748 ) ) ;
#54878=CARTESIAN_POINT ( 'NONE',  ( 30.68434753602730680, 1526.000688113718297, 201.3936004808388702 ) ) ;
#54879=LINE ( 'NONE', #79523, #17566 ) ;
#54893=EDGE_LOOP ( 'NONE', ( #69096, #27917, #17284, #102576 ) ) ;
#54909=FACE_OUTER_BOUND ( 'NONE', #77529, .T. ) ;
#54921=CARTESIAN_POINT ( 'NONE',  ( 2.792392588003544507, 1524.382868172863937, 176.8996806668726549 ) ) ;
#54939=LINE ( 'NONE', #28061, #42607 ) ;
#54952=CARTESIAN_POINT ( 'NONE',  ( -76.99707197885180676, 1524.382868172863937, 19.35599459046246551 ) ) ;
#54962=CARTESIAN_POINT ( 'NONE',  ( -20.98221433428902927, 1524.841055067849538, 237.1519650095371503 ) ) ;
#54969=EDGE_CURVE ( 'NONE', #48513, #20620, #89709, .T. ) ;
#54973=( BOUNDED_CURVE ( )  B_SPLINE_CURVE ( 3, ( #104818, #19129, #103711, #95316 ),
 .UNSPECIFIED., .F., .F. ) 
 B_SPLINE_CURVE_WITH_KNOTS ( ( 4, 4 ),
 ( 3.141592653589793116, 4.712388980384695891 ),
 .UNSPECIFIED. ) 
 CURVE ( )  GEOMETRIC_REPRESENTATION_ITEM ( )  RATIONAL_B_SPLINE_CURVE ( ( 1.000000000000000000, 0.8047378541243634942, 0.8047378541243634942, 1.000000000000000000 ) ) 
 REPRESENTATION_ITEM ( '' )  );
#54983=ORIENTED_EDGE ( 'NONE', *, *, #23454, .T. ) ;
#54986=CARTESIAN_POINT ( 'NONE',  ( 32.78250617288038171, 1511.187213306747708, 199.9357095655690841 ) ) ;
#54987=ADVANCED_FACE ( 'NONE', ( #68189 ), #59359, .T. ) ;
#55019=AXIS2_PLACEMENT_3D ( 'NONE', #83163, #65277, #23239 ) ;
#55034=DIRECTION ( 'NONE',  ( 0.000000000000000000, 1.000000000000000000, 0.000000000000000000 ) ) ;
#55047=ORIENTED_EDGE ( 'NONE', *, *, #59635, .T. ) ;
#55064=VERTEX_POINT ( 'NONE', #16609 ) ;
#55066=EDGE_CURVE ( 'NONE', #96612, #83385, #64143, .T. ) ;
#55075=EDGE_CURVE ( 'NONE', #967, #42994, #72998, .T. ) ;
#55086=CARTESIAN_POINT ( 'NONE',  ( 31.18494820112223209, 1524.152444737676660, 221.8763663153084167 ) ) ;
#55099=CARTESIAN_POINT ( 'NONE',  ( 16.81611548245179222, 1526.382868172864164, 183.6985842798745523 ) ) ;
#55103=CYLINDRICAL_SURFACE ( 'NONE', #76560, 1.000000000000009548 ) ;
#55108=TOROIDAL_SURFACE ( 'NONE', #46393, 1.000000000000000000, 1.000000000000000000 ) ;
#55111=AXIS2_PLACEMENT_3D ( 'NONE', #27141, #9236, #25999 ) ;
#55120=DIRECTION ( 'NONE',  ( 0.9774101051267759521, 0.000000000000000000, 0.2113515706023137153 ) ) ;
#55123=( BOUNDED_SURFACE ( )  B_SPLINE_SURFACE ( 3, 2, ( 
 ( #67034, #90550, #83260 ),
 ( #82712, #84359, #100600 ),
 ( #40153, #64839, #74877 ),
 ( #109028, #32310, #16032 ),
 ( #22770, #66494, #58076 ),
 ( #92754, #14384, #41261 ) ),
 .UNSPECIFIED., .F., .F., .F. ) 
 B_SPLINE_SURFACE_WITH_KNOTS ( ( 4, 2, 4 ),
 ( 3, 3 ),
 ( -3.252606517456513302E-18, 0.001312027981647327559, 0.002624055963294658154 ),
 ( 0.000000000000000000, 1.000000000000000000 ),
 .UNSPECIFIED. ) 
 GEOMETRIC_REPRESENTATION_ITEM ( )  RATIONAL_B_SPLINE_SURFACE ( (
 ( 1.000000000000000000, 0.9376006582765876729, 1.000000000000000000),
 ( 1.000000000000000000, 0.9569320108031822425, 1.000000000000000000),
 ( 1.000000000000000000, 0.9725743441606675699, 1.000000000000000000),
 ( 1.000000000000000000, 0.9942095667147810012, 1.000000000000000000),
 ( 1.000000000000000000, 1.000043666449794255, 1.000000000000000000),
 ( 1.000000000000000000, 1.000000000000000000, 1.000000000000000000) ) ) 
 REPRESENTATION_ITEM ( '' )  SURFACE ( )  );
#55124=ORIENTED_EDGE ( 'NONE', *, *, #53706, .T. ) ;
#55177=DIRECTION ( 'NONE',  ( 0.000000000000000000, 1.000000000000000000, 0.000000000000000000 ) ) ;
#55178=CARTESIAN_POINT ( 'NONE',  ( 20.68299495989132808, 1525.856064936158418, 233.9549337258506227 ) ) ;
#55181=ORIENTED_EDGE ( 'NONE', *, *, #40174, .F. ) ;
#55191=CIRCLE ( 'NONE', #35567, 1.000000000000015099 ) ;
#55207=DIRECTION ( 'NONE',  ( 0.000000000000000000, 1.000000000000000000, 0.000000000000000000 ) ) ;
#55215=B_SPLINE_CURVE_WITH_KNOTS ( 'NONE', 3,
 ( #102693, #87597, #52350, #9763, #103831, #25988 ),
 .UNSPECIFIED., .F., .F.,
 ( 4, 2, 4 ),
 ( -1.131363979618622308E-05, 0.001067788114096023932, 0.002146889867988234155 ),
 .UNSPECIFIED. ) ;
#55220=CARTESIAN_POINT ( 'NONE',  ( -29.00779973304124937, 1526.382868172863937, 217.2942086403127178 ) ) ;
#55232=ADVANCED_FACE ( 'NONE', ( #82350 ), #23599, .T. ) ;
#55237=DIRECTION ( 'NONE',  ( -0.000000000000000000, -1.000000000000000000, -0.000000000000000000 ) ) ;
#55244=CARTESIAN_POINT ( 'NONE',  ( 0.5770119038902318254, 1525.581535527370534, 243.3912443123664673 ) ) ;
#55250=CARTESIAN_POINT ( 'NONE',  ( -17.78793234590467875, 1523.919934424249959, 237.8334813054144661 ) ) ;
#55254=CARTESIAN_POINT ( 'NONE',  ( -2.458491834123362807, 1524.872178180562969, 242.3414668159568066 ) ) ;
#55256=EDGE_CURVE ( 'NONE', #42516, #89999, #98656, .T. ) ;
#55259=TOROIDAL_SURFACE ( 'NONE', #10472, 1.000000000000000000, 1.000000000000000000 ) ;
#55265=EDGE_CURVE ( 'NONE', #81551, #50617, #54025, .T. ) ;
#55290=ORIENTED_EDGE ( 'NONE', *, *, #23434, .F. ) ;
#55307=CARTESIAN_POINT ( 'NONE',  ( -33.23571934791657867, 1512.187213306747481, 219.4842663281467026 ) ) ;
#55319=VERTEX_POINT ( 'NONE', #5651 ) ;
#55333=AXIS2_PLACEMENT_3D ( 'NONE', #45506, #28675, #18044 ) ;
#55350=CARTESIAN_POINT ( 'NONE',  ( -1.393816646507353596, 1512.187213306747481, 175.1051575864439656 ) ) ;
#55352=FACE_OUTER_BOUND ( 'NONE', #5429, .T. ) ;
#55371=ORIENTED_EDGE ( 'NONE', *, *, #109623, .F. ) ;
#55372=B_SPLINE_CURVE_WITH_KNOTS ( 'NONE', 3,
 ( #47544, #81664, #4969, #39114, #73294, #104417 ),
 .UNSPECIFIED., .F., .F.,
 ( 4, 2, 4 ),
 ( -1.285435071109504191E-05, 0.001079388306740602238, 0.002171630964192299267 ),
 .UNSPECIFIED. ) ;
#55377=CARTESIAN_POINT ( 'NONE',  ( -16.77192111137985364, 1526.333389948038530, 234.9129815758640802 ) ) ;
#55384=CARTESIAN_POINT ( 'NONE',  ( -0.4151546846821903003, 1501.977400791986611, 242.9330574173806951 ) ) ;
#55398=AXIS2_PLACEMENT_3D ( 'NONE', #191, #68494, #94207 ) ;
#55400=DIRECTION ( 'NONE',  ( -0.3090169943749382919, 0.000000000000000000, 0.9510565162951565288 ) ) ;
#55410=CARTESIAN_POINT ( 'NONE',  ( 18.88880210473057275, 1524.667648926078527, 238.8296805722605427 ) ) ;
#55425=B_SPLINE_CURVE_WITH_KNOTS ( 'NONE', 3,
 ( #17836, #60444, #92915, #16188, #103516, #25143, #85603, #59347, #93456, #8904, #35219, #1093 ),
 .UNSPECIFIED., .F., .F.,
 ( 4, 2, 2, 2, 2, 4 ),
 ( 0.000000000000000000, 0.0007194225121804019834, 0.001079133768270288231, 0.001438845024360174262, 0.002158267536539345676, 0.002877690048718516656 ),
 .UNSPECIFIED. ) ;
#55431=ORIENTED_EDGE ( 'NONE', *, *, #12235, .F. ) ;
#55436=EDGE_CURVE ( 'NONE', #89438, #4434, #50419, .T. ) ;
#55438=AXIS2_PLACEMENT_3D ( 'NONE', #39848, #85691, #67818 ) ;
#55441=EDGE_CURVE ( 'NONE', #98871, #45131, #100497, .T. ) ;
#55442=EDGE_CURVE ( 'NONE', #52269, #98270, #31520, .T. ) ;
#55454=ORIENTED_EDGE ( 'NONE', *, *, #12755, .T. ) ;
#55462=CARTESIAN_POINT ( 'NONE',  ( 0.000000000000000000, 1523.051704408389696, 209.1218459616979999 ) ) ;
#55464=EDGE_LOOP ( 'NONE', ( #67726, #88657, #12171, #80779 ) ) ;
#55466=CIRCLE ( 'NONE', #84057, 30.13701971169416183 ) ;
#55470=CARTESIAN_POINT ( 'NONE',  ( 2.127574403380531720, 1524.244163922423695, 173.7332312662435925 ) ) ;
#55489=AXIS2_PLACEMENT_3D ( 'NONE', #64370, #99584, #5550 ) ;
#55495=ORIENTED_EDGE ( 'NONE', *, *, #80254, .T. ) ;
#55505=CARTESIAN_POINT ( 'NONE',  ( -22.66254714601714326, 1523.342713519622748, 236.8145175431329221 ) ) ;
#55515=DIRECTION ( 'NONE',  ( -0.000000000000000000, -1.000000000000000000, -0.000000000000000000 ) ) ;
#55521=CARTESIAN_POINT ( 'NONE',  ( 20.37381179411471877, 1524.397344074318880, 180.2832293763214579 ) ) ;
#55545=CARTESIAN_POINT ( 'NONE',  ( -3.350338079455597917, 1523.604703353109699, 176.1628856388066708 ) ) ;
#55552=AXIS2_PLACEMENT_3D ( 'NONE', #26051, #53512, #44547 ) ;
#55554=CARTESIAN_POINT ( 'NONE',  ( 32.02808312589916540, 1511.187213306747708, 198.2787714533495489 ) ) ;
#55559=DIRECTION ( 'NONE',  ( -0.1070030146457249254, 0.000000000000000000, 0.9942586961433763637 ) ) ;
#55563=CARTESIAN_POINT ( 'NONE',  ( 16.69343462643233877, 1526.373507135059526, 234.5422045024349984 ) ) ;
#55567=ADVANCED_FACE ( 'NONE', ( #59924 ), #35811, .T. ) ;
#55570=CIRCLE ( 'NONE', #30447, 1.000000000000000888 ) ;
#55582=CARTESIAN_POINT ( 'NONE',  ( 33.93019615848946557, 1501.977400791986611, 197.6607374645996060 ) ) ;
#55594=ORIENTED_EDGE ( 'NONE', *, *, #64856, .F. ) ;
#55597=EDGE_LOOP ( 'NONE', ( #41198, #35370, #60569, #88764 ) ) ;
#55603=AXIS2_PLACEMENT_3D ( 'NONE', #28623, #104227, #105892 ) ;
#55613=VERTEX_POINT ( 'NONE', #98457 ) ;
#55619=EDGE_LOOP ( 'NONE', ( #14995, #4831, #71179, #88213 ) ) ;
#55620=CARTESIAN_POINT ( 'NONE',  ( -17.83486663330526767, 1523.678648413191695, 180.3677388339002334 ) ) ;
#55623=EDGE_CURVE ( 'NONE', #97990, #84088, #41440, .T. ) ;
#55630=CARTESIAN_POINT ( 'NONE',  ( -22.03465957474402259, 1522.644714754858796, 182.8300405912373492 ) ) ;
#55634=ADVANCED_FACE ( 'NONE', ( #90607 ), #30427, .F. ) ;
#55644=CARTESIAN_POINT ( 'NONE',  ( -1.912903644476058096, 1526.104292489130557, 177.3592290664108759 ) ) ;
#55657=AXIS2_PLACEMENT_3D ( 'NONE', #91406, #65662, #14683 ) ;
#55663=DIRECTION ( 'NONE',  ( 0.4035202328300511176, 0.000000000000000000, 0.9149707217702551798 ) ) ;
#55669=CARTESIAN_POINT ( 'NONE',  ( 0.000000000000000000, 1523.382868172864164, 209.1218459616979999 ) ) ;
#55670=VECTOR ( 'NONE', #79755, 999.9999999999998863 ) ;
#55675=CIRCLE ( 'NONE', #7370, 2.000000000000001776 ) ;
#55683=CARTESIAN_POINT ( 'NONE',  ( 30.90487439922549484, 1525.907212628473644, 216.4335774778779466 ) ) ;
#55686=VECTOR ( 'NONE', #29762, 999.9999999999998863 ) ;
#55690=ORIENTED_EDGE ( 'NONE', *, *, #52210, .T. ) ;
#55699=CARTESIAN_POINT ( 'NONE',  ( -30.30080019752890053, 1526.189892541618974, 201.5450448376013810 ) ) ;
#55704=DIRECTION ( 'NONE',  ( -0.000000000000000000, -1.000000000000000000, -0.000000000000000000 ) ) ;
#55710=ORIENTED_EDGE ( 'NONE', *, *, #91022, .T. ) ;
#55729=CARTESIAN_POINT ( 'NONE',  ( 20.92528168611880091, 1525.790286462510039, 233.2531892700154685 ) ) ;
#55732=ADVANCED_FACE ( 'NONE', ( #18300 ), #33443, .T. ) ;
#55736=CARTESIAN_POINT ( 'NONE',  ( -28.49879435372614722, 1526.382868172571079, 198.4011524119066507 ) ) ;
#55740=EDGE_CURVE ( 'NONE', #9564, #42097, #73749, .T. ) ;
#55741=ORIENTED_EDGE ( 'NONE', *, *, #23070, .F. ) ;
#55759=AXIS2_PLACEMENT_3D ( 'NONE', #94619, #7316, #101902 ) ;
#55766=FACE_OUTER_BOUND ( 'NONE', #72888, .T. ) ;
#55773=VERTEX_POINT ( 'NONE', #84421 ) ;
#55777=( BOUNDED_SURFACE ( )  B_SPLINE_SURFACE ( 3, 2, ( 
 ( #96402, #92659, #35949 ),
 ( #33299, #70135, #76419 ),
 ( #110573, #93745, #16480 ),
 ( #93211, #52754, #19110 ),
 ( #78499, #101597, #1813 ),
 ( #19679, #24882, #104798 ),
 ( #104247, #87455, #79068 ),
 ( #27537, #61720, #95842 ),
 ( #70685, #59089, #28086 ),
 ( #53313, #50670, #15934 ) ),
 .UNSPECIFIED., .F., .F., .T. ) 
 B_SPLINE_SURFACE_WITH_KNOTS ( ( 4, 2, 2, 2, 4 ),
 ( 3, 3 ),
 ( 0.000000000000000000, 0.3926990816987241395, 0.7853981633974482790, 1.178097245096172418, 1.570796326794896558 ),
 ( 0.000000000000000000, 1.000000000000000000 ),
 .UNSPECIFIED. ) 
 GEOMETRIC_REPRESENTATION_ITEM ( )  RATIONAL_B_SPLINE_SURFACE ( (
 ( 1.000000000000000000, 0.7763623250684352772, 1.000000000000000000),
 ( 1.000000000000000000, 0.7763684247034601249, 1.000000000000000000),
 ( 1.000000000000000000, 0.7746454561798020721, 1.000000000000000000),
 ( 1.000000000000000000, 0.7679730451972409666, 1.000000000000000000),
 ( 1.000000000000000000, 0.7630177051947608646, 1.000000000000000000),
 ( 1.000000000000000000, 0.7504512394527353969, 1.000000000000000000),
 ( 1.000000000000000000, 0.7428408967928123996, 1.000000000000000000),
 ( 1.000000000000000000, 0.7259222650909311625, 1.000000000000000000),
 ( 1.000000000000000000, 0.7166207884820420260, 1.000000000000000000),
 ( 1.000000000000000000, 0.7071067811865825448, 1.000000000000000000) ) ) 
 REPRESENTATION_ITEM ( '' )  SURFACE ( )  );
#55802=DIRECTION ( 'NONE',  ( 0.3090169943749582204, 0.000000000000000000, 0.9510565162951500895 ) ) ;
#55810=CARTESIAN_POINT ( 'NONE',  ( -2.744860007232919674, 1525.790287071781449, 240.9440838819185160 ) ) ;
#55830=CIRCLE ( 'NONE', #7529, 2.000000000000000000 ) ;
#55839=CARTESIAN_POINT ( 'NONE',  ( 33.45065857238096640, 1524.841055067849084, 198.7780394437808127 ) ) ;
#55841=ORIENTED_EDGE ( 'NONE', *, *, #41460, .F. ) ;
#55861=ORIENTED_EDGE ( 'NONE', *, *, #94562, .T. ) ;
#55872=DIRECTION ( 'NONE',  ( 0.8672669759446586246, -1.225281874271768203E-16, -0.4978433412588814111 ) ) ;
#55896=ORIENTED_EDGE ( 'NONE', *, *, #106249, .T. ) ;
#55902=CARTESIAN_POINT ( 'NONE',  ( 0.000000000000000000, 1526.382868172863937, 177.3106345060153046 ) ) ;
#55904=CARTESIAN_POINT ( 'NONE',  ( 31.33756686635661026, 1523.580204110582372, 221.9021554030050538 ) ) ;
#55930=( BOUNDED_SURFACE ( )  B_SPLINE_SURFACE ( 3, 2, ( 
 ( #109355, #41592, #32635 ),
 ( #24210, #75747, #81922 ),
 ( #109891, #67361, #24747 ),
 ( #93076, #16351, #5227 ) ),
 .UNSPECIFIED., .F., .F., .F. ) 
 B_SPLINE_SURFACE_WITH_KNOTS ( ( 4, 4 ),
 ( 3, 3 ),
 ( 0.000000000000000000, 0.0002960034161023851105 ),
 ( 0.000000000000000000, 1.000000000000000000 ),
 .UNSPECIFIED. ) 
 GEOMETRIC_REPRESENTATION_ITEM ( )  RATIONAL_B_SPLINE_SURFACE ( (
 ( 1.000000000000000000, 0.8072480644198088973, 1.000000000000000000),
 ( 1.000000000000000000, 0.8072480346917787486, 1.000000000000000000),
 ( 1.000000000000000000, 0.8071723757218290940, 1.000000000000000000),
 ( 1.000000000000000000, 0.8070209408750043112, 1.000000000000000000) ) ) 
 REPRESENTATION_ITEM ( '' )  SURFACE ( )  );
#55935=CARTESIAN_POINT ( 'NONE',  ( 31.79839622030615587, 1525.159196711359755, 216.1507387728551066 ) ) ;
#55936=EDGE_LOOP ( 'NONE', ( #15669, #16950, #4808, #51519, #16947 ) ) ;
#55940=CARTESIAN_POINT ( 'NONE',  ( -31.79806488007560361, 1525.506916460679349, 217.0230655909559800 ) ) ;
#55947=CARTESIAN_POINT ( 'NONE',  ( -2.372478608332516892, 1512.187213306747481, 174.8996806668726549 ) ) ;
#55955=DIRECTION ( 'NONE',  ( 0.9786619618251657382, 0.000000000000000000, 0.2054769195713180285 ) ) ;
#55958=CARTESIAN_POINT ( 'NONE',  ( 18.72690275719072517, 1526.278758871496393, 236.1309272327557949 ) ) ;
#55995=ORIENTED_EDGE ( 'NONE', *, *, #6290, .F. ) ;
#56013=CARTESIAN_POINT ( 'NONE',  ( 2.397475438394585989, 1525.713797967456685, 175.0187375749330272 ) ) ;
#56035=VERTEX_POINT ( 'NONE', #12252 ) ;
#56043=CARTESIAN_POINT ( 'NONE',  ( 0.000000000000000000, 1512.187213306747481, 243.9330574173806951 ) ) ;
#56045=CARTESIAN_POINT ( 'NONE',  ( -32.80316127680809757, 1523.919934424249959, 201.0769002502127023 ) ) ;
#56060=CARTESIAN_POINT ( 'NONE',  ( 18.10570579382015310, 1525.713797967457140, 180.1226510103675196 ) ) ;
#56065=ORIENTED_EDGE ( 'NONE', *, *, #37244, .T. ) ;
#56073=FACE_OUTER_BOUND ( 'NONE', #3352, .T. ) ;
#56082=CARTESIAN_POINT ( 'NONE',  ( 2.596261494520243573, 1525.907212628473644, 177.4701144822248011 ) ) ;
#56126=AXIS2_PLACEMENT_3D ( 'NONE', #64547, #90813, #14656 ) ;
#56148=LINE ( 'NONE', #74065, #25721 ) ;
#56155=ADVANCED_FACE ( 'NONE', ( #96833 ), #84430, .T. ) ;
#56159=LINE ( 'NONE', #47761, #53426 ) ;
#56164=CARTESIAN_POINT ( 'NONE',  ( -1.191524307911311809, 1526.382868172863937, 179.0083900503167911 ) ) ;
#56173=CARTESIAN_POINT ( 'NONE',  ( 16.56816485275348683, 1526.186458717539153, 182.6341057012125191 ) ) ;
#56186=EDGE_CURVE ( 'NONE', #30404, #76248, #3888, .T. ) ;
#56205=CARTESIAN_POINT ( 'NONE',  ( -21.12212911286992068, 1511.187213306747708, 235.8226600804187285 ) ) ;
#56206=DIRECTION ( 'NONE',  ( 0.000000000000000000, 1.000000000000000000, 0.000000000000000000 ) ) ;
#56209=CIRCLE ( 'NONE', #106313, 24.69926344187880929 ) ;
#56213=CARTESIAN_POINT ( 'NONE',  ( 32.16567119605107195, 1524.523992613102564, 216.1007008506254579 ) ) ;
#56256=ORIENTED_EDGE ( 'NONE', *, *, #15827, .F. ) ;
#56264=CARTESIAN_POINT ( 'NONE',  ( -28.54794148642340090, 1526.382868172864164, 198.4382598900959351 ) ) ;
#56267=ORIENTED_EDGE ( 'NONE', *, *, #34587, .T. ) ;
#56288=AXIS2_PLACEMENT_3D ( 'NONE', #109335, #48333, #57836 ) ;
#56304=CARTESIAN_POINT ( 'NONE',  ( 31.32995031131192931, 1523.678648413191695, 196.3423562208913324 ) ) ;
#56311=CARTESIAN_POINT ( 'NONE',  ( 21.54116136303176532, 1523.462669333491021, 183.9310736449011188 ) ) ;
#56313=CARTESIAN_POINT ( 'NONE',  ( 33.42844755915471211, 1522.861859112238790, 222.1271778627165929 ) ) ;
#56317=EDGE_LOOP ( 'NONE', ( #69669, #67825, #8952, #100834 ) ) ;
#56318=DIRECTION ( 'NONE',  ( -0.000000000000000000, -1.000000000000000000, -0.000000000000000000 ) ) ;
#56334=AXIS2_PLACEMENT_3D ( 'NONE', #100724, #8325, #110795 ) ;
#56336=ORIENTED_EDGE ( 'NONE', *, *, #33687, .T. ) ;
#56365=EDGE_CURVE ( 'NONE', #50617, #53780, #32374, .T. ) ;
#56370=CARTESIAN_POINT ( 'NONE',  ( -0.4681535437661810684, 1524.397344074319335, 244.4282029790937827 ) ) ;
#56372=EDGE_CURVE ( 'NONE', #30502, #106529, #67097, .T. ) ;
#56378=ORIENTED_EDGE ( 'NONE', *, *, #75055, .T. ) ;
#56389=CARTESIAN_POINT ( 'NONE',  ( -2.470168521978398424, 1523.382868172864164, 175.3649660270905315 ) ) ;
#56393=ORIENTED_EDGE ( 'NONE', *, *, #54357, .F. ) ;
#56396=EDGE_LOOP ( 'NONE', ( #3549, #4851, #1452, #93135, #12878 ) ) ;
#56418=VERTEX_POINT ( 'NONE', #109092 ) ;
#56443=FACE_OUTER_BOUND ( 'NONE', #68217, .T. ) ;
#56450=CARTESIAN_POINT ( 'NONE',  ( 31.22294729666630531, 1523.678648413191695, 222.8955943986478019 ) ) ;
#56451=CYLINDRICAL_SURFACE ( 'NONE', #80591, 1.000000000000000888 ) ;
#56455=CARTESIAN_POINT ( 'NONE',  ( -21.38516915558007270, 1522.382868172863937, 180.3939891059723664 ) ) ;
#56459=CARTESIAN_POINT ( 'NONE',  ( -22.08327125186962192, 1523.604703353109699, 184.4267662568473725 ) ) ;
#56483=EDGE_LOOP ( 'NONE', ( #36420, #86482, #103461, #60978 ) ) ;
#56487=FACE_OUTER_BOUND ( 'NONE', #63137, .T. ) ;
#56488=VERTEX_POINT ( 'NONE', #90340 ) ;
#56490=ORIENTED_EDGE ( 'NONE', *, *, #65041, .T. ) ;
#56505=CARTESIAN_POINT ( 'NONE',  ( 20.71343476517535365, 1524.726013923371511, 238.3377464195763764 ) ) ;
#56515=CARTESIAN_POINT ( 'NONE',  ( -31.81407709659898941, 1522.644714754857659, 221.9534378623325210 ) ) ;
#56521=CARTESIAN_POINT ( 'NONE',  ( 3.351013500467394213, 1524.082740465118604, 176.2279750478597862 ) ) ;
#56540=EDGE_LOOP ( 'NONE', ( #80515, #10383, #91899, #2305 ) ) ;
#56579=ORIENTED_EDGE ( 'NONE', *, *, #45387, .T. ) ;
#56594=DIRECTION ( 'NONE',  ( -0.4978433412588795792, 0.000000000000000000, -0.8672669759446596238 ) ) ;
#56598=CARTESIAN_POINT ( 'NONE',  ( -21.41758936356487908, 1524.330813522192102, 234.0369194964266626 ) ) ;
#56601=DIRECTION ( 'NONE',  ( 0.000000000000000000, 1.000000000000000000, 0.000000000000000000 ) ) ;
#56605=CARTESIAN_POINT ( 'NONE',  ( 20.69714284706258312, 1525.848196786131666, 184.2818640063567557 ) ) ;
#56606=EDGE_CURVE ( 'NONE', #38713, #35962, #13620, .T. ) ;
#56619=ORIENTED_EDGE ( 'NONE', *, *, #106908, .F. ) ;
#56624=DIRECTION ( 'NONE',  ( -0.000000000000000000, -1.000000000000000000, -0.000000000000000000 ) ) ;
#56631=FACE_OUTER_BOUND ( 'NONE', #15069, .T. ) ;
#56640=EDGE_CURVE ( 'NONE', #21777, #38998, #996, .T. ) ;
#56654=CARTESIAN_POINT ( 'NONE',  ( 16.65100080374359237, 1526.335487865669847, 234.8974115816864128 ) ) ;
#56660=DIRECTION ( 'NONE',  ( 0.000000000000000000, 0.8286769424886156754, -0.5597271880011900347 ) ) ;
#56684=CARTESIAN_POINT ( 'NONE',  ( 31.34491295179421400, 1525.848198008145346, 217.0523385987458482 ) ) ;
#56689=CARTESIAN_POINT ( 'NONE',  ( -2.470168521978409970, 1523.382868172864164, 242.8787258963054398 ) ) ;
#56708=CARTESIAN_POINT ( 'NONE',  ( 16.50400130224750583, 1525.907212628473644, 181.9890130758377040 ) ) ;
#56711=CARTESIAN_POINT ( 'NONE',  ( -20.98221433428875216, 1524.841055067848174, 181.0917269138568884 ) ) ;
#56715=TOROIDAL_SURFACE ( 'NONE', #35273, 1.000000000000000000, 1.000000000000000000 ) ;
#56744=EDGE_CURVE ( 'NONE', #36172, #101207, #39278, .T. ) ;
#56748=B_SPLINE_CURVE_WITH_KNOTS ( 'NONE', 3,
 ( #99179, #22459, #82411, #39850, #67820, #68378, #51008, #51558, #85141, #52119, #8429, #52669 ),
 .UNSPECIFIED., .F., .F.,
 ( 4, 2, 2, 2, 2, 4 ),
 ( 0.000000000000000000, 0.0007194225121792416702, 0.001079133768269177141, 0.001438845024359112828, 0.002158267536538995262, 0.002877690048718877912 ),
 .UNSPECIFIED. ) ;
#56752=EDGE_CURVE ( 'NONE', #40624, #98891, #30321, .T. ) ;
#56762=DIRECTION ( 'NONE',  ( -0.000000000000000000, -1.000000000000000000, -0.000000000000000000 ) ) ;
#56763=CARTESIAN_POINT ( 'NONE',  ( 1.336192060408132321, 1526.382868172863937, 239.5677422944788475 ) ) ;
#56765=CARTESIAN_POINT ( 'NONE',  ( -30.17514222261029744, 1525.712835404586031, 221.2664189270033432 ) ) ;
#56769=CARTESIAN_POINT ( 'NONE',  ( 31.79805362023550330, 1525.506926151470907, 217.0230659451404733 ) ) ;
#56780=CARTESIAN_POINT ( 'NONE',  ( 16.66231036550726685, 1523.604703353109699, 237.7554842931445478 ) ) ;
#56804=DIRECTION ( 'NONE',  ( 0.000000000000000000, 1.000000000000000000, 0.000000000000000000 ) ) ;
#56810=CYLINDRICAL_SURFACE ( 'NONE', #33948, 1.999999999999995559 ) ;
#56811=CARTESIAN_POINT ( 'NONE',  ( -22.75273496409615603, 1518.913060387330006, 183.6728937936775310 ) ) ;
#56813=EDGE_LOOP ( 'NONE', ( #102002, #103346, #70912, #63141 ) ) ;
#56819=CARTESIAN_POINT ( 'NONE',  ( -33.28034951413935971, 1512.187213306747481, 200.8029765415142549 ) ) ;
#56836=CARTESIAN_POINT ( 'NONE',  ( -30.87183381296014062, 1524.816846803860926, 196.4948539558456844 ) ) ;
#56840=AXIS2_PLACEMENT_3D ( 'NONE', #2387, #43804, #105929 ) ;
#56853=EDGE_CURVE ( 'NONE', #8029, #57810, #23164, .T. ) ;
#56864=CARTESIAN_POINT ( 'NONE',  ( -19.37374569213963582, 1526.382868172863937, 183.8768763279542213 ) ) ;
#56870=EDGE_LOOP ( 'NONE', ( #87828, #96666, #9519, #75278 ) ) ;
#56888=ORIENTED_EDGE ( 'NONE', *, *, #51811, .T. ) ;
#56896=LINE ( 'NONE', #108393, #84254 ) ;
#56899=DIRECTION ( 'NONE',  ( 0.000000000000000000, 1.000000000000000000, 0.000000000000000000 ) ) ;
#56903=ORIENTED_EDGE ( 'NONE', *, *, #97593, .F. ) ;
#56925=VECTOR ( 'NONE', #104809, 1000.000000000000000 ) ;
#56936=CARTESIAN_POINT ( 'NONE',  ( -21.38516915557943321, 1501.977400791986611, 237.8497028174240313 ) ) ;
#56972=ORIENTED_EDGE ( 'NONE', *, *, #7034, .T. ) ;
#56981=ADVANCED_FACE ( 'NONE', ( #99573 ), #40789, .F. ) ;
#57023=CARTESIAN_POINT ( 'NONE',  ( -21.54116136303384721, 1523.462669333493295, 183.9310736449068884 ) ) ;
#57026=CARTESIAN_POINT ( 'NONE',  ( 33.36586802512172767, 1518.913060387330006, 201.9069332299488622 ) ) ;
#57043=ADVANCED_FACE ( 'NONE', ( #74418 ), #108544, .T. ) ;
#57047=EDGE_LOOP ( 'NONE', ( #87804, #50655, #64904, #60828 ) ) ;
#57053=ORIENTED_EDGE ( 'NONE', *, *, #95934, .T. ) ;
#57061=APPLICATION_CONTEXT ( 'automotive_design' ) ;
#57068=DIRECTION ( 'NONE',  ( 0.000000000000000000, 1.000000000000000000, 0.000000000000000000 ) ) ;
#57088=CARTESIAN_POINT ( 'NONE',  ( 30.45769963431402871, 1526.208281990536307, 201.0929247824067829 ) ) ;
#57111=EDGE_CURVE ( 'NONE', #40948, #17784, #41033, .T. ) ;
#57139=CARTESIAN_POINT ( 'NONE',  ( 30.36938634820355176, 1525.506926151471134, 196.8236402350184449 ) ) ;
#57164=TOROIDAL_SURFACE ( 'NONE', #87610, 1.000000000000000000, 1.000000000000000000 ) ;
#57168=CARTESIAN_POINT ( 'NONE',  ( -21.61625474793734369, 1526.178928173327904, 234.4801574852453996 ) ) ;
#57176=CARTESIAN_POINT ( 'NONE',  ( -2.792392588003332232, 1526.382868172863937, 176.8996806668727118 ) ) ;
#57181=ORIENTED_EDGE ( 'NONE', *, *, #101059, .T. ) ;
#57188=CARTESIAN_POINT ( 'NONE',  ( -16.55384015340527526, 1524.739915903632664, 180.7880258469990338 ) ) ;
#57189=CARTESIAN_POINT ( 'NONE',  ( -33.36586802512182715, 1511.187213306747708, 201.9069332299493169 ) ) ;
#57206=ORIENTED_EDGE ( 'NONE', *, *, #82268, .F. ) ;
#57213=AXIS2_PLACEMENT_3D ( 'NONE', #70420, #104538, #35123 ) ;
#57235=DIRECTION ( 'NONE',  ( 0.2054769195713296581, -0.000000000000000000, 0.9786619618251632957 ) ) ;
#57254=ORIENTED_EDGE ( 'NONE', *, *, #105505, .T. ) ;
#57261=AXIS2_PLACEMENT_3D ( 'NONE', #1882, #60685, #52281 ) ;
#57299=ADVANCED_FACE ( 'NONE', ( #99442 ), #10479, .T. ) ;
#57338=CARTESIAN_POINT ( 'NONE',  ( -30.47385413848724411, 1525.394081235439444, 221.5015873865095841 ) ) ;
#57342=CARTESIAN_POINT ( 'NONE',  ( 31.81429855202634727, 1524.964158026965833, 216.6572713097424128 ) ) ;
#57345=B_SPLINE_CURVE_WITH_KNOTS ( 'NONE', 3,
 ( #79841, #106133, #105032, #87692, #28878, #88236 ),
 .UNSPECIFIED., .F., .F.,
 ( 4, 2, 4 ),
 ( 2.081668171172168513E-17, 0.001087661325621749582, 0.002175322651243478348 ),
 .UNSPECIFIED. ) ;
#57354=CARTESIAN_POINT ( 'NONE',  ( 16.99775931995016620, 1524.964230758899930, 237.0504197537864286 ) ) ;
#57372=CARTESIAN_POINT ( 'NONE',  ( -31.34137657934027388, 1512.187213306747481, 196.3411265156551906 ) ) ;
#57403=CIRCLE ( 'NONE', #39318, 30.13701971169416183 ) ;
#57418=FACE_OUTER_BOUND ( 'NONE', #71593, .T. ) ;
#57443=CYLINDRICAL_SURFACE ( 'NONE', #48209, 33.13701971169416538 ) ;
#57457=ORIENTED_EDGE ( 'NONE', *, *, #58975, .F. ) ;
#57460=CARTESIAN_POINT ( 'NONE',  ( -17.83486663330464950, 1523.678648413191695, 237.8759530894961074 ) ) ;
#57472=ORIENTED_EDGE ( 'NONE', *, *, #95210, .F. ) ;
#57491=CARTESIAN_POINT ( 'NONE',  ( 34.68852446352943986, 1522.382868172864164, 199.9946320047951076 ) ) ;
#57494=ORIENTED_EDGE ( 'NONE', *, *, #89809, .T. ) ;
#57501=CARTESIAN_POINT ( 'NONE',  ( 3.614223185718036913, 1512.187213306747481, 237.6097657867469195 ) ) ;
#57502=CARTESIAN_POINT ( 'NONE',  ( 0.4151546846821903003, 1512.187213306747481, 244.9330574173806951 ) ) ;
#57530=CARTESIAN_POINT ( 'NONE',  ( 30.87201549882245644, 1524.816548299036640, 196.4947534715130644 ) ) ;
#57546=ORIENTED_EDGE ( 'NONE', *, *, #20664, .T. ) ;
#57551=CARTESIAN_POINT ( 'NONE',  ( -2.857353854284550021, 1525.661275128775742, 241.0960500474518255 ) ) ;
#57569=DIRECTION ( 'NONE',  ( -0.9125304618754027652, 0.000000000000000000, -0.4090087482554184417 ) ) ;
#57571=CARTESIAN_POINT ( 'NONE',  ( -31.50799703744288749, 1526.382868172863937, 201.8203724569134749 ) ) ;
#57583=FACE_OUTER_BOUND ( 'NONE', #103037, .T. ) ;
#57584=TOROIDAL_SURFACE ( 'NONE', #32303, 1.000000000000000000, 1.000000000000000000 ) ;
#57597=( BOUNDED_SURFACE ( )  B_SPLINE_SURFACE ( 3, 2, ( 
 ( #14408, #74361, #81076 ),
 ( #4392, #106821, #108489 ),
 ( #30112, #21699, #55904 ),
 ( #2032, #34934, #103806 ) ),
 .UNSPECIFIED., .F., .F., .T. ) 
 B_SPLINE_SURFACE_WITH_KNOTS ( ( 4, 4 ),
 ( 3, 3 ),
 ( 0.000000000000000000, 0.0002960034161023845684 ),
 ( 0.000000000000000000, 1.000000000000000000 ),
 .UNSPECIFIED. ) 
 GEOMETRIC_REPRESENTATION_ITEM ( )  RATIONAL_B_SPLINE_SURFACE ( (
 ( 1.000000000000000000, 0.8072480644198078981, 1.000000000000000000),
 ( 1.000000000000000000, 0.8072480346917859650, 1.000000000000000000),
 ( 1.000000000000000000, 0.8071723757218217665, 1.000000000000000000),
 ( 1.000000000000000000, 0.8070209408750090851, 1.000000000000000000) ) ) 
 REPRESENTATION_ITEM ( '' )  SURFACE ( )  );
#57599=EDGE_CURVE ( 'NONE', #23656, #21237, #101507, .T. ) ;
#57608=ORIENTED_EDGE ( 'NONE', *, *, #74787, .F. ) ;
#57609=ORIENTED_EDGE ( 'NONE', *, *, #50453, .F. ) ;
#57616=B_SPLINE_CURVE_WITH_KNOTS ( 'NONE', 3,
 ( #23619, #79889, #30009, #11575 ),
 .UNSPECIFIED., .F., .F.,
 ( 4, 4 ),
 ( 0.000000000000000000, 0.0002220129587134777476 ),
 .UNSPECIFIED. ) ;
#57634=CARTESIAN_POINT ( 'NONE',  ( 31.32995031131189378, 1523.678648413191695, 196.3423562208913324 ) ) ;
#57642=EDGE_CURVE ( 'NONE', #13824, #50505, #78620, .T. ) ;
#57645=CARTESIAN_POINT ( 'NONE',  ( 29.00779973304118542, 1526.382868172864164, 200.9494832830835378 ) ) ;
#57653=CARTESIAN_POINT ( 'NONE',  ( -2.121003584631406813, 1512.187213306747481, 239.6750300321239138 ) ) ;
#57676=ADVANCED_FACE ( 'NONE', ( #42186 ), #76336, .T. ) ;
#57696=ADVANCED_FACE ( 'NONE', ( #97404 ), #39365, .T. ) ;
#57701=TOROIDAL_SURFACE ( 'NONE', #52349, 30.13701971169416538, 3.000000000000000000 ) ;
#57702=CARTESIAN_POINT ( 'NONE',  ( 31.41104781486818354, 1511.187213306747708, 202.3296363711535264 ) ) ;
#57709=EDGE_CURVE ( 'NONE', #71433, #91018, #7147, .T. ) ;
#57725=CARTESIAN_POINT ( 'NONE',  ( -2.792392588003544507, 1524.382868172863937, 176.8996806668726549 ) ) ;
#57739=CARTESIAN_POINT ( 'NONE',  ( -17.53704155054333214, 1524.872178180564788, 180.8015429009317074 ) ) ;
#57750=CARTESIAN_POINT ( 'NONE',  ( -18.00465857450842933, 1523.390106123591067, 238.0296012445041072 ) ) ;
#57758=ORIENTED_EDGE ( 'NONE', *, *, #96690, .T. ) ;
#57779=VERTEX_POINT ( 'NONE', #32413 ) ;
#57810=VERTEX_POINT ( 'NONE', #48680 ) ;
#57836=DIRECTION ( 'NONE',  ( 0.000000000000000000, 0.000000000000000000, 1.000000000000000000 ) ) ;
#57868=EDGE_CURVE ( 'NONE', #108592, #84410, #100159, .T. ) ;
#57879=CARTESIAN_POINT ( 'NONE',  ( 32.32093690483868187, 1524.075000532257491, 216.0999125871069850 ) ) ;
#57891=CARTESIAN_POINT ( 'NONE',  ( 17.62867182259785181, 1524.547873515805350, 237.6135799091316585 ) ) ;
#57904=EDGE_LOOP ( 'NONE', ( #107437, #28447, #3395, #44099, #53837 ) ) ;
#57925=EDGE_LOOP ( 'NONE', ( #36795, #46467, #93192, #88809 ) ) ;
#57959=CARTESIAN_POINT ( 'NONE',  ( -21.10561344245444815, 1525.661275128775742, 233.3100099925564450 ) ) ;
#57967=DIRECTION ( 'NONE',  ( 0.000000000000000000, 1.000000000000000000, 0.000000000000000000 ) ) ;
#57974=CYLINDRICAL_SURFACE ( 'NONE', #26272, 2.000000000000007550 ) ;
#57981=CIRCLE ( 'NONE', #90077, 1.000000000000001332 ) ;
#58019=FACE_OUTER_BOUND ( 'NONE', #104728, .T. ) ;
#58040=EDGE_CURVE ( 'NONE', #73515, #4626, #19181, .T. ) ;
#58046=CYLINDRICAL_SURFACE ( 'NONE', #41503, 1.000000000000000888 ) ;
#58052=EDGE_LOOP ( 'NONE', ( #1999, #13136, #50208, #27233, #53119 ) ) ;
#58057=AXIS2_PLACEMENT_3D ( 'NONE', #21844, #56594, #14011 ) ;
#58074=ORIENTED_EDGE ( 'NONE', *, *, #100969, .F. ) ;
#58076=CARTESIAN_POINT ( 'NONE',  ( -28.44964981546823779, 1526.382868172864164, 219.8796466721389606 ) ) ;
#58090=AXIS2_PLACEMENT_3D ( 'NONE', #74074, #16323, #75721 ) ;
#58093=CARTESIAN_POINT ( 'NONE',  ( -29.35073940689260752, 1526.211523310372058, 197.7230717947574306 ) ) ;
#58112=CARTESIAN_POINT ( 'NONE',  ( 2.478617600774434049, 1524.659802833172535, 175.7713138579284475 ) ) ;
#58123=ORIENTED_EDGE ( 'NONE', *, *, #37818, .F. ) ;
#58133=CARTESIAN_POINT ( 'NONE',  ( 19.67623451925446076, 1525.581535527372807, 181.0581612215006260 ) ) ;
#58142=CARTESIAN_POINT ( 'NONE',  ( 33.28034951413137321, 1522.644714754858796, 217.4407153818774248 ) ) ;
#58150=CARTESIAN_POINT ( 'NONE',  ( 18.07041998555279960, 1523.313115944345554, 180.1545818505811667 ) ) ;
#58163=ORIENTED_EDGE ( 'NONE', *, *, #96530, .T. ) ;
#58164=CIRCLE ( 'NONE', #15203, 2.000000000000001776 ) ;
#58165=CARTESIAN_POINT ( 'NONE',  ( 18.02257621027596812, 1526.382868172863937, 235.3484976865586589 ) ) ;
#58183=VERTEX_POINT ( 'NONE', #99309 ) ;
#58198=ORIENTED_EDGE ( 'NONE', *, *, #60466, .T. ) ;
#58201=ORIENTED_EDGE ( 'NONE', *, *, #48262, .F. ) ;
#58242=( BOUNDED_SURFACE ( )  B_SPLINE_SURFACE ( 3, 2, ( 
 ( #101334, #31953, #92959 ),
 ( #16232, #93502, #14595 ),
 ( #50436, #67784, #48785 ),
 ( #100796, #76718, #76168 ) ),
 .UNSPECIFIED., .F., .F., .T. ) 
 B_SPLINE_SURFACE_WITH_KNOTS ( ( 4, 4 ),
 ( 3, 3 ),
 ( 0.000000000000000000, 0.0002960034161023854899 ),
 ( 0.000000000000000000, 1.000000000000000000 ),
 .UNSPECIFIED. ) 
 GEOMETRIC_REPRESENTATION_ITEM ( )  RATIONAL_B_SPLINE_SURFACE ( (
 ( 1.000000000000000000, 0.8072480644198084532, 1.000000000000000000),
 ( 1.000000000000000000, 0.8072480346917723093, 1.000000000000000000),
 ( 1.000000000000000000, 0.8071723757218308704, 1.000000000000000000),
 ( 1.000000000000000000, 0.8070209408749940971, 1.000000000000000000) ) ) 
 REPRESENTATION_ITEM ( '' )  SURFACE ( )  );
#58247=FACE_OUTER_BOUND ( 'NONE', #40985, .T. ) ;
#58254=ADVANCED_FACE ( 'NONE', ( #43845 ), #77992, .T. ) ;
#58269=CARTESIAN_POINT ( 'NONE',  ( 2.596261494520241353, 1525.907212628473644, 177.4701144822246874 ) ) ;
#58274=CARTESIAN_POINT ( 'NONE',  ( -17.83486663330525346, 1523.678648413191695, 180.3677388339002334 ) ) ;
#58294=VECTOR ( 'NONE', #3917, 1000.000000000000000 ) ;
#58317=AXIS2_PLACEMENT_3D ( 'NONE', #63958, #71832, #20807 ) ;
#58318=FACE_OUTER_BOUND ( 'NONE', #96747, .T. ) ;
#58330=VERTEX_POINT ( 'NONE', #98639 ) ;
#58351=ORIENTED_EDGE ( 'NONE', *, *, #11652, .T. ) ;
#58353=ADVANCED_FACE ( 'NONE', ( #82407 ), #5703, .T. ) ;
#58371=ORIENTED_EDGE ( 'NONE', *, *, #11350, .F. ) ;
#58375=CARTESIAN_POINT ( 'NONE',  ( -21.83550407203881960, 1523.678648413191695, 234.9693198511253911 ) ) ;
#58396=EDGE_CURVE ( 'NONE', #70982, #56035, #11096, .T. ) ;
#58399=CIRCLE ( 'NONE', #36948, 0.9999999999999326095 ) ;
#58413=CARTESIAN_POINT ( 'NONE',  ( 21.19077256501174844, 1525.394081235439444, 234.2786530305002657 ) ) ;
#58428=ORIENTED_EDGE ( 'NONE', *, *, #37201, .F. ) ;
#58438=CARTESIAN_POINT ( 'NONE',  ( 0.000000000000000000, 1511.187213306747708, 209.1218459616979999 ) ) ;
#58453=ORIENTED_EDGE ( 'NONE', *, *, #19366, .F. ) ;
#58463=CARTESIAN_POINT ( 'NONE',  ( 22.03465957474570658, 1512.187213306747481, 235.4136513321629991 ) ) ;
#58471=ADVANCED_FACE ( 'NONE', ( #104705 ), #100176, .T. ) ;
#58472=ORIENTED_EDGE ( 'NONE', *, *, #78189, .F. ) ;
#58473=ORIENTED_EDGE ( 'NONE', *, *, #47380, .F. ) ;
#58486=VERTEX_POINT ( 'NONE', #20678 ) ;
#58489=EDGE_CURVE ( 'NONE', #87976, #108859, #52667, .T. ) ;
#58506=CARTESIAN_POINT ( 'NONE',  ( 21.82415348264087740, 1524.756004293092474, 184.6268171959276287 ) ) ;
#58509=CARTESIAN_POINT ( 'NONE',  ( 17.43549125882616124, 1525.211477436245787, 181.0323534358458062 ) ) ;
#58526=CARTESIAN_POINT ( 'NONE',  ( 33.42844755917196409, 1522.382868172863937, 222.1271778627165929 ) ) ;
#58534=EDGE_CURVE ( 'NONE', #81290, #16271, #75108, .T. ) ;
#58544=CARTESIAN_POINT ( 'NONE',  ( -20.68299495988535242, 1525.856064936169560, 184.2887581975230376 ) ) ;
#58547=DIRECTION ( 'NONE',  ( 0.000000000000000000, 0.000000000000000000, 1.000000000000000000 ) ) ;
#58552=VECTOR ( 'NONE', #65151, 1000.000000000000000 ) ;
#58563=DIRECTION ( 'NONE',  ( -0.000000000000000000, -1.000000000000000000, -0.000000000000000000 ) ) ;
#58567=DIRECTION ( 'NONE',  ( 0.5877852522924673639, 0.000000000000000000, -0.8090169943749514481 ) ) ;
#58590=CARTESIAN_POINT ( 'NONE',  ( 1.439851189671822240, 1526.382868172864164, 239.5034140466408417 ) ) ;
#58598=ORIENTED_EDGE ( 'NONE', *, *, #72638, .T. ) ;
#58608=CIRCLE ( 'NONE', #105120, 1.000000000000000888 ) ;
#58627=CIRCLE ( 'NONE', #94400, 33.13701971169416538 ) ;
#58632=CARTESIAN_POINT ( 'NONE',  ( 20.92767404034498924, 1511.187213306747708, 182.8548762971663848 ) ) ;
#58637=DIRECTION ( 'NONE',  ( -0.8090169943749507819, 0.000000000000000000, -0.5877852522924685852 ) ) ;
#58639=CARTESIAN_POINT ( 'NONE',  ( -3.316380893998936763, 1524.425415513988810, 241.9071459675778613 ) ) ;
#58659=CARTESIAN_POINT ( 'NONE',  ( 2.494575337237918689, 1524.201816949777367, 175.5410045932797516 ) ) ;
#58660=CYLINDRICAL_SURFACE ( 'NONE', #98676, 1.000000000000003775 ) ;
#58673=AXIS2_PLACEMENT_3D ( 'NONE', #20092, #29061, #38543 ) ;
#58677=AXIS2_PLACEMENT_3D ( 'NONE', #52243, #17480, #42723 ) ;
#58682=CARTESIAN_POINT ( 'NONE',  ( 19.07966196791809210, 1524.244163922423695, 179.2412984082194214 ) ) ;
#58690=CARTESIAN_POINT ( 'NONE',  ( 31.47409394596150634, 1526.278758871497985, 218.5859237437351510 ) ) ;
#58694=ORIENTED_EDGE ( 'NONE', *, *, #56372, .F. ) ;
#58699=CARTESIAN_POINT ( 'NONE',  ( -2.472529913803022783, 1523.678648413191695, 242.8674788698241400 ) ) ;
#58730=ORIENTED_EDGE ( 'NONE', *, *, #59060, .T. ) ;
#58737=CARTESIAN_POINT ( 'NONE',  ( -0.4151546846821903003, 1511.187213306747708, 175.3106345060153046 ) ) ;
#58759=ORIENTED_EDGE ( 'NONE', *, *, #8925, .T. ) ;
#58777=B_SPLINE_CURVE_WITH_KNOTS ( 'NONE', 3,
 ( #38957, #73136, #107831, #28931 ),
 .UNSPECIFIED., .F., .F.,
 ( 4, 4 ),
 ( 0.000000000000000000, 0.0002220129587134776663 ),
 .UNSPECIFIED. ) ;
#58782=CARTESIAN_POINT ( 'NONE',  ( -32.38114538885258753, 1523.604703353109699, 202.1233279672532888 ) ) ;
#58788=CARTESIAN_POINT ( 'NONE',  ( -17.17241001986523941, 1518.913060387330006, 179.6185504016045797 ) ) ;
#58795=CARTESIAN_POINT ( 'NONE',  ( -29.00779973304138437, 1526.382868172864164, 200.9494832830839073 ) ) ;
#58799=CARTESIAN_POINT ( 'NONE',  ( 30.31052258194597115, 1523.604703353109699, 222.4930856806589929 ) ) ;
#58814=DIRECTION ( 'NONE',  ( 0.9510565162951566398, 0.000000000000000000, -0.3090169943749382919 ) ) ;
#58820=CARTESIAN_POINT ( 'NONE',  ( -16.57695357294941019, 1524.524650307242837, 180.6873389552785625 ) ) ;
#58823=DIRECTION ( 'NONE',  ( 0.9786619618251632957, -0.000000000000000000, 0.2054769195713296581 ) ) ;
#58832=CARTESIAN_POINT ( 'NONE',  ( -18.19590854887641740, 1522.644714754858796, 238.2026672068733433 ) ) ;
#58855=CARTESIAN_POINT ( 'NONE',  ( -29.37542415142184993, 1526.382868172864164, 217.2587022579325833 ) ) ;
#58863=ORIENTED_EDGE ( 'NONE', *, *, #52153, .T. ) ;
#58866=DIRECTION ( 'NONE',  ( -0.8672669759446699489, 0.000000000000000000, -0.4978433412588613716 ) ) ;
#58921=VERTEX_POINT ( 'NONE', #14790 ) ;
#58924=CARTESIAN_POINT ( 'NONE',  ( -21.75647715750836753, 1524.201816949742124, 234.8230427201935697 ) ) ;
#58942=AXIS2_PLACEMENT_3D ( 'NONE', #92500, #109331, #35222 ) ;
#58971=DIRECTION ( 'NONE',  ( 0.3090169943749515036, -0.000000000000000000, 0.9510565162951521989 ) ) ;
#58975=EDGE_CURVE ( 'NONE', #40624, #105727, #82886, .T. ) ;
#58979=TOROIDAL_SURFACE ( 'NONE', #80403, 2.000000000000000000, 1.000000000000000000 ) ;
#58988=FACE_OUTER_BOUND ( 'NONE', #78596, .T. ) ;
#58991=CARTESIAN_POINT ( 'NONE',  ( 17.59770716511923894, 1524.659802833172989, 237.5598880769025243 ) ) ;
#58992=CIRCLE ( 'NONE', #7102, 2.000000000000001776 ) ;
#59028=ORIENTED_EDGE ( 'NONE', *, *, #74320, .T. ) ;
#59056=DIRECTION ( 'NONE',  ( 1.040834085586083310E-14, 0.000000000000000000, 1.000000000000000000 ) ) ;
#59057=CARTESIAN_POINT ( 'NONE',  ( 21.92916355573829890, 1523.390106123591067, 183.0654104491179908 ) ) ;
#59060=EDGE_CURVE ( 'NONE', #100304, #34471, #52539, .T. ) ;
#59065=ADVANCED_FACE ( 'NONE', ( #88640 ), #100849, .F. ) ;
#59089=CARTESIAN_POINT ( 'NONE',  ( -31.95643112690575549, 1526.329757971585195, 216.6807372299043095 ) ) ;
#59092=DIRECTION ( 'NONE',  ( 0.9983395709201744461, -0.05760296116452706672, 0.000000000000000000 ) ) ;
#59094=ADVANCED_FACE ( 'NONE', ( #74585 ), #77550, .T. ) ;
#59121=CIRCLE ( 'NONE', #82359, 30.10786454236638576 ) ;
#59143=EDGE_CURVE ( 'NONE', #13894, #75732, #66201, .T. ) ;
#59164=ORIENTED_EDGE ( 'NONE', *, *, #15213, .F. ) ;
#59174=DIRECTION ( 'NONE',  ( 0.03173147633638118831, -0.9969860201949398704, 0.07079540200725417676 ) ) ;
#59192=AXIS2_PLACEMENT_3D ( 'NONE', #101768, #100673, #76589 ) ;
#59202=AXIS2_PLACEMENT_3D ( 'NONE', #69026, #9628, #69583 ) ;
#59209=DIRECTION ( 'NONE',  ( 0.000000000000000000, 0.000000000000000000, 1.000000000000000000 ) ) ;
#59221=CARTESIAN_POINT ( 'NONE',  ( 3.302346719094112260, 1524.524650307243519, 176.3741577287142661 ) ) ;
#59228=CARTESIAN_POINT ( 'NONE',  ( 17.84054674790834127, 1523.580204110584191, 180.3625987835367539 ) ) ;
#59233=CARTESIAN_POINT ( 'NONE',  ( 17.17241001986506888, 1512.187213306747481, 238.6251415217915337 ) ) ;
#59259=CARTESIAN_POINT ( 'NONE',  ( 0.000000000000000000, 1512.187213306747481, 174.3106345060153046 ) ) ;
#59261=CARTESIAN_POINT ( 'NONE',  ( -2.372478608332516892, 1522.382868172863937, 243.3440112565233449 ) ) ;
#59266=DIRECTION ( 'NONE',  ( 0.000000000000000000, 1.000000000000000000, 0.000000000000000000 ) ) ;
#59279=CARTESIAN_POINT ( 'NONE',  ( -21.12212911287051043, 1511.187213306747708, 182.4210318429776976 ) ) ;
#59294=ORIENTED_EDGE ( 'NONE', *, *, #19121, .T. ) ;
#59313=ORIENTED_EDGE ( 'NONE', *, *, #77539, .T. ) ;
#59318=ORIENTED_EDGE ( 'NONE', *, *, #54357, .T. ) ;
#59347=CARTESIAN_POINT ( 'NONE',  ( -16.51112239071575516, 1525.159177407155767, 181.0518290279077576 ) ) ;
#59351=ORIENTED_EDGE ( 'NONE', *, *, #65082, .F. ) ;
#59359=TOROIDAL_SURFACE ( 'NONE', #82606, 1.000000000000000000, 1.000000000000000000 ) ;
#59371=AXIS2_PLACEMENT_3D ( 'NONE', #96089, #10433, #77642 ) ;
#59376=CARTESIAN_POINT ( 'NONE',  ( -2.372478608334043670, 1522.644714754858114, 174.8996806668799024 ) ) ;
#59385=CARTESIAN_POINT ( 'NONE',  ( 22.03465957474570658, 1501.977400791986611, 235.4136513321629991 ) ) ;
#59388=DIRECTION ( 'NONE',  ( -0.7414773880254650340, 0.000000000000000000, 0.6709778558543747495 ) ) ;
#59389=ORIENTED_EDGE ( 'NONE', *, *, #83893, .T. ) ;
#59393=CARTESIAN_POINT ( 'NONE',  ( -16.73628186595857059, 1526.382868172863937, 184.0591879540917546 ) ) ;
#59397=DIRECTION ( 'NONE',  ( -0.000000000000000000, -1.000000000000000000, -0.000000000000000000 ) ) ;
#59400=CARTESIAN_POINT ( 'NONE',  ( -17.61183580542321536, 1523.982201850120191, 237.6741279912556593 ) ) ;
#59406=DIRECTION ( 'NONE',  ( 0.5032920991128559951, -0.8641163480519131745, 0.000000000000000000 ) ) ;
#59413=DIRECTION ( 'NONE',  ( -0.2054769195713296304, 0.000000000000000000, 0.9786619618251631847 ) ) ;
#59426=VERTEX_POINT ( 'NONE', #49246 ) ;
#59437=CARTESIAN_POINT ( 'NONE',  ( 22.04658257820665668, 1524.075000532257263, 233.7649905024729549 ) ) ;
#59464=VERTEX_POINT ( 'NONE', #85567 ) ;
#59484=CARTESIAN_POINT ( 'NONE',  ( -21.30905559963850493, 1524.964230758882877, 233.9180796557699864 ) ) ;
#59491=FACE_OUTER_BOUND ( 'NONE', #51152, .T. ) ;
#59508=DIRECTION ( 'NONE',  ( 0.000000000000000000, 0.000000000000000000, 1.000000000000000000 ) ) ;
#59521=CARTESIAN_POINT ( 'NONE',  ( -3.448830483803564828, 1512.187213306747481, 175.1594891075192209 ) ) ;
#59536=CARTESIAN_POINT ( 'NONE',  ( 17.22627300067414069, 1525.856064936170469, 181.7773026866640862 ) ) ;
#59553=ORIENTED_EDGE ( 'NONE', *, *, #73495, .T. ) ;
#59554=EDGE_LOOP ( 'NONE', ( #14289, #80497, #4429, #17096 ) ) ;
#59557=EDGE_LOOP ( 'NONE', ( #88210, #75887, #67236, #88075 ) ) ;
#59588=ORIENTED_EDGE ( 'NONE', *, *, #60401, .T. ) ;
#59595=ORIENTED_EDGE ( 'NONE', *, *, #43284, .F. ) ;
#59600=CARTESIAN_POINT ( 'NONE',  ( 19.90023153800465749, 1526.278758871497303, 182.9652379492366094 ) ) ;
#59605=ADVANCED_FACE ( 'NONE', ( #100715 ), #26217, .T. ) ;
#59610=CARTESIAN_POINT ( 'NONE',  ( 30.64453888532167269, 1525.163527997505753, 221.6135595047366849 ) ) ;
#59611=EDGE_CURVE ( 'NONE', #83466, #23328, #93424, .T. ) ;
#59635=EDGE_CURVE ( 'NONE', #95178, #7253, #76092, .T. ) ;
#59643=CARTESIAN_POINT ( 'NONE',  ( -20.20959865099510111, 1512.187213306747481, 182.0120230947222524 ) ) ;
#59646=CARTESIAN_POINT ( 'NONE',  ( 0.000000000000000000, 1522.051704408389924, 209.1218459616979999 ) ) ;
#59651=AXIS2_PLACEMENT_3D ( 'NONE', #3623, #97108, #63000 ) ;
#59658=CARTESIAN_POINT ( 'NONE',  ( 0.000000000000000000, 1523.382868172864164, 209.1218459616979999 ) ) ;
#59661=CARTESIAN_POINT ( 'NONE',  ( -32.30068554584621410, 1526.382868172863937, 198.0073124585818789 ) ) ;
#59684=CARTESIAN_POINT ( 'NONE',  ( -31.92108011125358757, 1511.187213306747708, 197.2845127572065849 ) ) ;
#59693=CARTESIAN_POINT ( 'NONE',  ( 1.338895077072648876, 1526.382868172864164, 239.5739613961636110 ) ) ;
#59704=ORIENTED_EDGE ( 'NONE', *, *, #55436, .F. ) ;
#59707=FACE_BOUND ( 'NONE', #69075, .T. ) ;
#59723=ORIENTED_EDGE ( 'NONE', *, *, #101680, .F. ) ;
#59734=FACE_OUTER_BOUND ( 'NONE', #33629, .T. ) ;
#59735=EDGE_CURVE ( 'NONE', #237, #59464, #102605, .T. ) ;
#59738=DIRECTION ( 'NONE',  ( 0.000000000000000000, 0.000000000000000000, 1.000000000000000000 ) ) ;
#59742=CARTESIAN_POINT ( 'NONE',  ( 21.54116136312531893, 1523.382868172863937, 234.3126182787002278 ) ) ;
#59771=DIRECTION ( 'NONE',  ( 0.000000000000000000, 0.000000000000000000, 1.000000000000000000 ) ) ;
#59777=CARTESIAN_POINT ( 'NONE',  ( -3.448830483803573710, 1523.382868172864164, 243.0842028158767505 ) ) ;
#59781=DIRECTION ( 'NONE',  ( 0.000000000000000000, 0.000000000000000000, 1.000000000000000000 ) ) ;
#59799=ORIENTED_EDGE ( 'NONE', *, *, #19692, .F. ) ;
#59826=DIRECTION ( 'NONE',  ( -0.4035202328300226404, 0.000000000000000000, 0.9149707217702675033 ) ) ;
#59846=CARTESIAN_POINT ( 'NONE',  ( -3.237130272123891928, 1524.843178112495480, 176.5219626358610583 ) ) ;
#59852=EDGE_CURVE ( 'NONE', #2574, #39868, #54392, .T. ) ;
#59873=EDGE_LOOP ( 'NONE', ( #1195, #14245, #108169, #11740 ) ) ;
#59876=DIRECTION ( 'NONE',  ( 0.000000000000000000, 1.000000000000000000, 0.000000000000000000 ) ) ;
#59890=CARTESIAN_POINT ( 'NONE',  ( 30.64459234690374956, 1525.163457223743762, 196.6300966631588381 ) ) ;
#59895=CIRCLE ( 'NONE', #106312, 1.000000000000000888 ) ;
#59899=AXIS2_PLACEMENT_3D ( 'NONE', #65027, #99145, #22423 ) ;
#59924=FACE_OUTER_BOUND ( 'NONE', #6241, .T. ) ;
#59929=EDGE_CURVE ( 'NONE', #30213, #911, #102673, .T. ) ;
#59935=DIRECTION ( 'NONE',  ( -0.9942586961433756976, -0.000000000000000000, -0.1070030146457317671 ) ) ;
#59936=DIRECTION ( 'NONE',  ( -0.000000000000000000, -1.000000000000000000, -0.000000000000000000 ) ) ;
#59940=VERTEX_POINT ( 'NONE', #77223 ) ;
#59942=AXIS2_PLACEMENT_3D ( 'NONE', #104165, #95217, #88475 ) ;
#59950=DIRECTION ( 'NONE',  ( 0.000000000000000000, 0.000000000000000000, -1.000000000000000000 ) ) ;
#59959=ORIENTED_EDGE ( 'NONE', *, *, #104861, .F. ) ;
#59960=CARTESIAN_POINT ( 'NONE',  ( -20.20959865099451847, 1522.382868172863937, 236.2316688286741453 ) ) ;
#59978=DIRECTION ( 'NONE',  ( 0.000000000000000000, 0.000000000000000000, 1.000000000000000000 ) ) ;
#59983=VECTOR ( 'NONE', #68087, 1000.000000000000000 ) ;
#59986=CARTESIAN_POINT ( 'NONE',  ( -17.84338787571960339, 1523.481610426287716, 180.3600277896300383 ) ) ;
#59987=CARTESIAN_POINT ( 'NONE',  ( 21.75649307329755899, 1524.201670966335314, 234.8230823334607749 ) ) ;
#59990=CARTESIAN_POINT ( 'NONE',  ( 18.51436573157379328, 1511.187213306747708, 237.1421867457405881 ) ) ;
#60003=DIRECTION ( 'NONE',  ( 0.000000000000000000, 0.000000000000000000, -1.000000000000000000 ) ) ;
#60007=AXIS2_PLACEMENT_3D ( 'NONE', #25031, #75483, #14429 ) ;
#60016=EDGE_LOOP ( 'NONE', ( #74275, #94546, #96762, #66025 ) ) ;
#60022=( BOUNDED_CURVE ( )  B_SPLINE_CURVE ( 3, ( #92862, #86128, #84471, #110219 ),
 .UNSPECIFIED., .F., .F. ) 
 B_SPLINE_CURVE_WITH_KNOTS ( ( 4, 4 ),
 ( 2.436781329611987790, 3.141592653589793116 ),
 .UNSPECIFIED. ) 
 CURVE ( )  GEOMETRIC_REPRESENTATION_ITEM ( )  RATIONAL_B_SPLINE_CURVE ( ( 1.000000000000000000, 0.9590300661663092585, 0.9590300661663092585, 1.000000000000000000 ) ) 
 REPRESENTATION_ITEM ( '' )  );
#60036=DIRECTION ( 'NONE',  ( 0.4978433412588676998, 0.000000000000000000, -0.8672669759446663962 ) ) ;
#60060=B_SPLINE_CURVE_WITH_KNOTS ( 'NONE', 3,
 ( #56389, #83231, #82684, #23311 ),
 .UNSPECIFIED., .F., .F.,
 ( 4, 4 ),
 ( 0.000000000000000000, 0.0002960034161023854899 ),
 .UNSPECIFIED. ) ;
#60063=AXIS2_PLACEMENT_3D ( 'NONE', #4910, #29560, #107371 ) ;
#60096=CARTESIAN_POINT ( 'NONE',  ( 17.53714238134822168, 1524.871836253779975, 180.8013275667260871 ) ) ;
#60116=CARTESIAN_POINT ( 'NONE',  ( 21.08095450301371088, 1525.506916460680713, 184.0391914173981149 ) ) ;
#60122=LINE ( 'NONE', #96467, #48671 ) ;
#60157=LINE ( 'NONE', #75846, #64264 ) ;
#60158=CARTESIAN_POINT ( 'NONE',  ( 21.19880661589004589, 1524.382868172863937, 184.6948938244647991 ) ) ;
#60159=B_SPLINE_CURVE_WITH_KNOTS ( 'NONE', 3,
 ( #93922, #87198, #69315, #44101, #84969, #96146, #78239, #95048 ),
 .UNSPECIFIED., .F., .F.,
 ( 4, 2, 2, 4 ),
 ( 0.000000000000000000, 0.001073044933456263018, 0.001609567400184377722, 0.002146089866912492643 ),
 .UNSPECIFIED. ) ;
#60166=CARTESIAN_POINT ( 'NONE',  ( 22.04555908422425148, 1524.082740465118832, 184.4798216974346872 ) ) ;
#60172=EDGE_LOOP ( 'NONE', ( #79248, #62152, #82111, #15883 ) ) ;
#60183=DIRECTION ( 'NONE',  ( 0.000000000000000000, 0.000000000000000000, -1.000000000000000000 ) ) ;
#60198=CARTESIAN_POINT ( 'NONE',  ( 18.66420869458043441, 1526.382868172864164, 185.4599087859680537 ) ) ;
#60211=AXIS2_PLACEMENT_3D ( 'NONE', #2805, #104682, #78954 ) ;
#60220=ORIENTED_EDGE ( 'NONE', *, *, #106249, .F. ) ;
#60233=CARTESIAN_POINT ( 'NONE',  ( 31.92108011125342770, 1511.187213306747708, 197.2845127572061301 ) ) ;
#60240=DIRECTION ( 'NONE',  ( 0.000000000000000000, 0.000000000000000000, 1.000000000000000000 ) ) ;
#60259=CARTESIAN_POINT ( 'NONE',  ( -21.19077256501192608, 1525.394081235439444, 183.9650388928959615 ) ) ;
#60262=B_SPLINE_CURVE_WITH_KNOTS ( 'NONE', 3,
 ( #98852, #23787, #82044, #99945 ),
 .UNSPECIFIED., .F., .F.,
 ( 4, 4 ),
 ( 0.000000000000000000, 0.0002220129587134776663 ),
 .UNSPECIFIED. ) ;
#60269=DIRECTION ( 'NONE',  ( 0.000000000000000000, 1.000000000000000000, 0.000000000000000000 ) ) ;
#60300=CARTESIAN_POINT ( 'NONE',  ( -22.03465957474591619, 1501.977400791986611, 182.8300405912331144 ) ) ;
#60301=CARTESIAN_POINT ( 'NONE',  ( -32.86802468386297704, 1501.977400791986611, 201.0396662540046577 ) ) ;
#60303=CARTESIAN_POINT ( 'NONE',  ( 21.41971086555102133, 1511.187213306747708, 233.0798096144380906 ) ) ;
#60316=DIRECTION ( 'NONE',  ( -0.9942586961433764747, -2.969930264099993005E-15, -0.1070030146457249115 ) ) ;
#60333=EDGE_CURVE ( 'NONE', #51540, #100609, #13167, .T. ) ;
#60337=CARTESIAN_POINT ( 'NONE',  ( 33.42844755917187882, 1501.977400791986611, 196.1165140606791226 ) ) ;
#60399=CARTESIAN_POINT ( 'NONE',  ( -2.708183792730093131, 1524.374142163904253, 176.2566682395902262 ) ) ;
#60401=EDGE_CURVE ( 'NONE', #83342, #23737, #86565, .T. ) ;
#60402=DIRECTION ( 'NONE',  ( 0.000000000000000000, 0.000000000000000000, -1.000000000000000000 ) ) ;
#60405=ADVANCED_FACE ( 'NONE', ( #36969 ), #67724, .F. ) ;
#60413=ORIENTED_EDGE ( 'NONE', *, *, #82503, .F. ) ;
#60414=EDGE_LOOP ( 'NONE', ( #8473, #110396, #71105, #101256 ) ) ;
#60441=CARTESIAN_POINT ( 'NONE',  ( 31.16645442585767611, 1524.201670966335314, 196.3723102679300894 ) ) ;
#60443=AXIS2_PLACEMENT_3D ( 'NONE', #93356, #16620, #23932 ) ;
#60444=CARTESIAN_POINT ( 'NONE',  ( -16.64685887467744507, 1523.847248782568613, 180.5000237996434578 ) ) ;
#60450=CIRCLE ( 'NONE', #106848, 1.000000000000002442 ) ;
#60453=VECTOR ( 'NONE', #33788, 1000.000000000000000 ) ;
#60466=EDGE_CURVE ( 'NONE', #27462, #94190, #83371, .T. ) ;
#60492=DIRECTION ( 'NONE',  ( 0.000000000000000000, -0.07593562622321022026, -0.9971127221483482295 ) ) ;
#60493=EDGE_CURVE ( 'NONE', #13288, #6825, #50842, .T. ) ;
#60498=CARTESIAN_POINT ( 'NONE',  ( -34.18677586421195258, 1501.977400791986611, 198.4504086008750505 ) ) ;
#60503=EDGE_LOOP ( 'NONE', ( #15315, #50600, #39584, #102509 ) ) ;
#60512=EDGE_CURVE ( 'NONE', #73683, #106220, #40825, .T. ) ;
#60531=ADVANCED_FACE ( 'NONE', ( #82282 ), #65162, .T. ) ;
#60555=ORIENTED_EDGE ( 'NONE', *, *, #104087, .T. ) ;
#60569=ORIENTED_EDGE ( 'NONE', *, *, #55740, .T. ) ;
#60595=CARTESIAN_POINT ( 'NONE',  ( -20.17436656406320594, 1524.841055067849766, 180.5047911526357325 ) ) ;
#60613=AXIS2_PLACEMENT_3D ( 'NONE', #8581, #26484, #84188 ) ;
#60621=CARTESIAN_POINT ( 'NONE',  ( 17.27380372710132406, 1525.712830164893376, 236.6835243611168380 ) ) ;
#60624=DIRECTION ( 'NONE',  ( -0.000000000000000000, -1.000000000000000000, -0.000000000000000000 ) ) ;
#60635=CARTESIAN_POINT ( 'NONE',  ( 29.41145195048112271, 1525.795403383247276, 196.6862061498684113 ) ) ;
#60636=AXIS2_PLACEMENT_3D ( 'NONE', #65923, #14923, #83250 ) ;
#60647=CYLINDRICAL_SURFACE ( 'NONE', #58677, 2.000000000000000000 ) ;
#60654=CARTESIAN_POINT ( 'NONE',  ( 17.36692104388846047, 1525.425686270225242, 181.2365643868851635 ) ) ;
#60668=FILL_AREA_STYLE_COLOUR ( '', #106654 ) ;
#60685=DIRECTION ( 'NONE',  ( -1.000000000000000000, -0.000000000000000000, -0.000000000000000000 ) ) ;
#60717=ORIENTED_EDGE ( 'NONE', *, *, #67242, .F. ) ;
#60722=ORIENTED_EDGE ( 'NONE', *, *, #55442, .F. ) ;
#60733=DIRECTION ( 'NONE',  ( -0.6709778558543689764, 0.000000000000000000, 0.7414773880254701410 ) ) ;
#60737=CARTESIAN_POINT ( 'NONE',  ( 30.04653961079798208, 1524.739915903632891, 222.3142848390757251 ) ) ;
#60756=FACE_OUTER_BOUND ( 'NONE', #54893, .T. ) ;
#60771=CARTESIAN_POINT ( 'NONE',  ( -22.08622291482368638, 1523.382868172864164, 184.4183880513178337 ) ) ;
#60812=VECTOR ( 'NONE', #44269, 1000.000000000000000 ) ;
#60813=CARTESIAN_POINT ( 'NONE',  ( -31.81429855202636858, 1524.964158026965606, 201.5864206136516543 ) ) ;
#60828=ORIENTED_EDGE ( 'NONE', *, *, #15472, .F. ) ;
#60829=FACE_OUTER_BOUND ( 'NONE', #94020, .T. ) ;
#60847=ORIENTED_EDGE ( 'NONE', *, *, #44574, .T. ) ;
#60852=CIRCLE ( 'NONE', #12551, 1.000000000000000888 ) ;
#60886=CARTESIAN_POINT ( 'NONE',  ( -33.45065857237997875, 1524.841055067850220, 198.7780394437810401 ) ) ;
#60887=CARTESIAN_POINT ( 'NONE',  ( -21.63718167644571722, 1524.600389084707103, 234.6742851132877945 ) ) ;
#60890=CARTESIAN_POINT ( 'NONE',  ( 32.02808312589916540, 1512.187213306747481, 198.2787714533495489 ) ) ;
#60915=CARTESIAN_POINT ( 'NONE',  ( 30.31940284292419818, 1523.382868172864164, 222.4933038710543087 ) ) ;
#60921=DIRECTION ( 'NONE',  ( -0.000000000000000000, -1.000000000000000000, -0.000000000000000000 ) ) ;
#60939=CARTESIAN_POINT ( 'NONE',  ( -19.37374569213905318, 1526.382868172863937, 234.3668155954421479 ) ) ;
#60948=CIRCLE ( 'NONE', #50225, 33.13701971169416538 ) ;
#60957=CIRCLE ( 'NONE', #26967, 0.9999999999999865663 ) ;
#60963=LINE ( 'NONE', #36280, #6291 ) ;
#60978=ORIENTED_EDGE ( 'NONE', *, *, #22759, .F. ) ;
#61011=CARTESIAN_POINT ( 'NONE',  ( 2.273033093151271000, 1525.821544997590308, 240.9339456143063387 ) ) ;
#61019=DIRECTION ( 'NONE',  ( -0.5877852522924625900, 0.000000000000000000, 0.8090169943749551118 ) ) ;
#61020=AXIS2_PLACEMENT_3D ( 'NONE', #83003, #64581, #13570 ) ;
#61045=DIRECTION ( 'NONE',  ( 0.8672669759446699489, 0.000000000000000000, 0.4978433412588613716 ) ) ;
#61050=VECTOR ( 'NONE', #109883, 1000.000000000000000 ) ;
#61059=CIRCLE ( 'NONE', #66406, 1.000000000000000888 ) ;
#61072=ORIENTED_EDGE ( 'NONE', *, *, #34587, .F. ) ;
#61075=CARTESIAN_POINT ( 'NONE',  ( -32.02808312589908013, 1512.187213306747481, 219.9649204700466782 ) ) ;
#61077=VERTEX_POINT ( 'NONE', #11553 ) ;
#61084=CARTESIAN_POINT ( 'NONE',  ( -32.74318896774677512, 1524.667648926078300, 222.0534297170888465 ) ) ;
#61124=AXIS2_PLACEMENT_3D ( 'NONE', #86223, #103009, #26306 ) ;
#61142=CARTESIAN_POINT ( 'NONE',  ( -20.20959865099510111, 1501.977400791986611, 182.0120230947222524 ) ) ;
#61143=DIRECTION ( 'NONE',  ( 0.000000000000000000, 0.000000000000000000, -1.000000000000000000 ) ) ;
#61145=CARTESIAN_POINT ( 'NONE',  ( -31.32995031131182628, 1523.678648413191695, 221.9013357025048947 ) ) ;
#61161=CARTESIAN_POINT ( 'NONE',  ( -21.14964295068569200, 1525.231887713368451, 233.8093806080460126 ) ) ;
#61162=ADVANCED_FACE ( 'NONE', ( #65827 ), #7539, .T. ) ;
#61170=EDGE_CURVE ( 'NONE', #102300, #5040, #60262, .T. ) ;
#61187=DIRECTION ( 'NONE',  ( 0.000000000000000000, 1.000000000000000000, 0.000000000000000000 ) ) ;
#61192=DIRECTION ( 'NONE',  ( -0.000000000000000000, -1.000000000000000000, -0.000000000000000000 ) ) ;
#61203=CARTESIAN_POINT ( 'NONE',  ( -30.31052258194604931, 1523.604703353109699, 195.7506062427371774 ) ) ;
#61223=CARTESIAN_POINT ( 'NONE',  ( 16.49279160078992490, 1525.408337840050308, 181.2883413873725260 ) ) ;
#61233=CARTESIAN_POINT ( 'NONE',  ( -30.95751052620457600, 1525.821544997590081, 201.4531494772889459 ) ) ;
#61244=CARTESIAN_POINT ( 'NONE',  ( 21.15382147014735281, 1525.425665131969254, 183.9878842466098376 ) ) ;
#61248=FACE_OUTER_BOUND ( 'NONE', #27982, .T. ) ;
#61261=DIRECTION ( 'NONE',  ( 0.9942586961433749204, 0.000000000000000000, -0.1070030146457386366 ) ) ;
#61279=EDGE_CURVE ( 'NONE', #89888, #54724, #109832, .T. ) ;
#61290=CARTESIAN_POINT ( 'NONE',  ( 22.01290455779290767, 1522.906363951597314, 182.8785777331706015 ) ) ;
#61317=EDGE_CURVE ( 'NONE', #67344, #108102, #11527, .T. ) ;
#61328=FACE_OUTER_BOUND ( 'NONE', #32478, .T. ) ;
#61335=CARTESIAN_POINT ( 'NONE',  ( -32.09235212274882088, 1525.402221411319488, 196.2603058525792790 ) ) ;
#61369=CARTESIAN_POINT ( 'NONE',  ( -31.12456774391179337, 1525.960063244516959, 201.1524202391566405 ) ) ;
#61413=EDGE_LOOP ( 'NONE', ( #12080, #45013 ) ) ;
#61436=CARTESIAN_POINT ( 'NONE',  ( -31.44837959398599736, 1512.187213306747481, 197.3353852117985525 ) ) ;
#61446=DIRECTION ( 'NONE',  ( 0.000000000000000000, -1.000000000000000000, 0.000000000000000000 ) ) ;
#61453=CARTESIAN_POINT ( 'NONE',  ( 21.12212911287033279, 1511.187213306747708, 235.8226600804184443 ) ) ;
#61471=CARTESIAN_POINT ( 'NONE',  ( -32.28466283162165240, 1511.187213306747708, 199.0684425896249081 ) ) ;
#61511=DIRECTION ( 'NONE',  ( 0.2054769195713296304, -0.000000000000000000, 0.9786619618251631847 ) ) ;
#61519=VERTEX_POINT ( 'NONE', #74477 ) ;
#61537=EDGE_LOOP ( 'NONE', ( #65525, #80230, #52293 ) ) ;
#61541=ORIENTED_EDGE ( 'NONE', *, *, #36371, .F. ) ;
#61559=CARTESIAN_POINT ( 'NONE',  ( 22.14913372576120310, 1525.402221411349956, 235.6690521037248232 ) ) ;
#61578=CARTESIAN_POINT ( 'NONE',  ( 33.93019615848955084, 1524.726013923371283, 220.5829544587961095 ) ) ;
#61591=ORIENTED_EDGE ( 'NONE', *, *, #77087, .F. ) ;
#61597=CARTESIAN_POINT ( 'NONE',  ( -16.66700976312892735, 1523.530935881284904, 237.7590780485276127 ) ) ;
#61600=CARTESIAN_POINT ( 'NONE',  ( -17.17241001986462123, 1511.187213306747708, 238.6251415217917895 ) ) ;
#61615=B_SPLINE_CURVE_WITH_KNOTS ( 'NONE', 3,
 ( #68655, #104997, #102756, #1433 ),
 .UNSPECIFIED., .F., .F.,
 ( 4, 4 ),
 ( 0.000000000000000000, 0.0002220129587134779374 ),
 .UNSPECIFIED. ) ;
#61617=CARTESIAN_POINT ( 'NONE',  ( -32.99911596133562597, 1524.244163922424150, 222.0809728102186114 ) ) ;
#61619=CARTESIAN_POINT ( 'NONE',  ( 32.54480841269636926, 1524.547873515804895, 201.1604127401539586 ) ) ;
#61626=CARTESIAN_POINT ( 'NONE',  ( -2.356894939219843721, 1525.394081235439444, 176.3139379204273496 ) ) ;
#61633=ORIENTED_EDGE ( 'NONE', *, *, #27517, .F. ) ;
#61664=AXIS2_PLACEMENT_3D ( 'NONE', #63942, #4567, #106468 ) ;
#61677=ORIENTED_EDGE ( 'NONE', *, *, #870, .T. ) ;
#61699=CARTESIAN_POINT ( 'NONE',  ( -18.37487226820799080, 1526.382868172863937, 182.5038319547590788 ) ) ;
#61711=CIRCLE ( 'NONE', #18734, 2.000000000000001776 ) ;
#61716=DIRECTION ( 'NONE',  ( -0.000000000000000000, -1.000000000000000000, -0.000000000000000000 ) ) ;
#61720=CARTESIAN_POINT ( 'NONE',  ( -32.39315898239540559, 1526.178928173328131, 216.9314351822684728 ) ) ;
#61737=EDGE_CURVE ( 'NONE', #84088, #91565, #75864, .T. ) ;
#61760=DIRECTION ( 'NONE',  ( 0.5877852522924709167, 0.000000000000000000, 0.8090169943749491166 ) ) ;
#61766=CARTESIAN_POINT ( 'NONE',  ( -18.69816095120731347, 1526.382868172863937, 234.8576566410005171 ) ) ;
#61782=CARTESIAN_POINT ( 'NONE',  ( 21.64969004981279355, 1524.547873515805122, 183.5515527622214051 ) ) ;
#61785=CIRCLE ( 'NONE', #102884, 2.000000000000001776 ) ;
#61831=EDGE_CURVE ( 'NONE', #51540, #94625, #22265, .T. ) ;
#61841=CARTESIAN_POINT ( 'NONE',  ( 30.61618914730548724, 1525.211473355384669, 221.5983863950426382 ) ) ;
#61843=AXIS2_PLACEMENT_3D ( 'NONE', #100420, #108269, #65733 ) ;
#61845=CARTESIAN_POINT ( 'NONE',  ( 30.57064947821818635, 1523.844789899200805, 221.8563555303887540 ) ) ;
#61847=ORIENTED_EDGE ( 'NONE', *, *, #74879, .T. ) ;
#61851=DIRECTION ( 'NONE',  ( 0.3090169943749447312, 0.000000000000000000, -0.9510565162951544194 ) ) ;
#61862=EDGE_CURVE ( 'NONE', #101705, #73940, #109906, .T. ) ;
#61883=CARTESIAN_POINT ( 'NONE',  ( -33.42844755916929245, 1522.861859112238335, 196.1165140606796058 ) ) ;
#61884=DIRECTION ( 'NONE',  ( -0.000000000000000000, -1.000000000000000000, -0.000000000000000000 ) ) ;
#61894=VERTEX_POINT ( 'NONE', #40718 ) ;
#61915=AXIS2_PLACEMENT_3D ( 'NONE', #25922, #76912, #16953 ) ;
#61920=CARTESIAN_POINT ( 'NONE',  ( -31.11295621078938467, 1525.790286462509584, 201.8987511033408566 ) ) ;
#61958=CARTESIAN_POINT ( 'NONE',  ( -22.08622291482368638, 1523.382868172864164, 184.4183880513178337 ) ) ;
#61971=ORIENTED_EDGE ( 'NONE', *, *, #98052, .T. ) ;
#61986=CARTESIAN_POINT ( 'NONE',  ( -18.97665094185341772, 1526.382868172863937, 185.2759924068388671 ) ) ;
#61992=CARTESIAN_POINT ( 'NONE',  ( -31.74003925670054116, 1524.382868172804365, 201.6871716353068678 ) ) ;
#62003=DIRECTION ( 'NONE',  ( -0.8672669759446630655, 0.000000000000000000, 0.4978433412588735285 ) ) ;
#62019=DIRECTION ( 'NONE',  ( -0.5877852522924585932, 0.000000000000000000, 0.8090169943749579984 ) ) ;
#62027=CARTESIAN_POINT ( 'NONE',  ( -29.79881796581627640, 1526.748660780343698, 196.6633055964660457 ) ) ;
#62039=CARTESIAN_POINT ( 'NONE',  ( 3.141370515551505260, 1525.159196711359755, 241.5359652250428155 ) ) ;
#62047=CARTESIAN_POINT ( 'NONE',  ( -17.17241001986523941, 1512.187213306747481, 179.6185504016045797 ) ) ;
#62083=EDGE_LOOP ( 'NONE', ( #35637, #26883, #22360, #46926 ) ) ;
#62115=CARTESIAN_POINT ( 'NONE',  ( 2.444993193446221014, 1524.972383263452912, 242.2724965207514174 ) ) ;
#62116=ORIENTED_EDGE ( 'NONE', *, *, #77606, .T. ) ;
#62118=CARTESIAN_POINT ( 'NONE',  ( 21.41758936356528054, 1524.330813522192102, 234.0369194964263784 ) ) ;
#62134=AXIS2_PLACEMENT_3D ( 'NONE', #101042, #102151, #60183 ) ;
#62151=CARTESIAN_POINT ( 'NONE',  ( -32.48417584039620465, 1524.659802833171170, 217.0704217325891250 ) ) ;
#62152=ORIENTED_EDGE ( 'NONE', *, *, #89173, .T. ) ;
#62154=EDGE_LOOP ( 'NONE', ( #107953, #37236, #65792, #57608 ) ) ;
#62161=AXIS2_PLACEMENT_3D ( 'NONE', #15117, #21308, #90177 ) ;
#62172=( BOUNDED_SURFACE ( )  B_SPLINE_SURFACE ( 3, 2, ( 
 ( #56780, #67403, #33214 ),
 ( #65190, #14758, #22576 ),
 ( #101502, #23152, #74143 ),
 ( #49490, #15834, #57891 ),
 ( #48389, #108825, #58991 ),
 ( #31560, #24789, #7467 ),
 ( #91479, #93120, #100424 ),
 ( #99302, #57354, #83613 ),
 ( #48945, #41067, #73596 ),
 ( #50584, #66849, #75245 ),
 ( #40515, #109936, #107725 ),
 ( #109395, #66306, #100959 ),
 ( #82532, #83076, #32671 ),
 ( #32121, #90918, #24255 ) ),
 .UNSPECIFIED., .F., .F., .F. ) 
 B_SPLINE_SURFACE_WITH_KNOTS ( ( 4, 2, 2, 2, 2, 2, 4 ),
 ( 3, 3 ),
 ( 0.000000000000000000, 0.0009440840677143978732, 0.001416126101571596810, 0.001888168135428795746, 0.002360210169285994683, 0.002832252203143193620, 0.003776336270857591493 ),
 ( 0.000000000000000000, 1.000000000000000000 ),
 .UNSPECIFIED. ) 
 GEOMETRIC_REPRESENTATION_ITEM ( )  RATIONAL_B_SPLINE_SURFACE ( (
 ( 1.000000000000000000, 0.8070209408750101954, 1.000000000000000000),
 ( 1.000000000000000000, 0.8215603905280027819, 1.000000000000000000),
 ( 1.000000000000000000, 0.8340988699066211876, 1.000000000000000000),
 ( 1.000000000000000000, 0.8516751610455791655, 1.000000000000000000),
 ( 1.000000000000000000, 0.8573697395154757928, 1.000000000000000000),
 ( 1.000000000000000000, 0.8683586635661659781, 1.000000000000000000),
 ( 1.000000000000000000, 0.8736518481709149020, 1.000000000000000000),
 ( 1.000000000000000000, 0.8840377753029594610, 1.000000000000000000),
 ( 1.000000000000000000, 0.8891294171303589788, 1.000000000000000000),
 ( 1.000000000000000000, 0.8992456600576572701, 1.000000000000000000),
 ( 1.000000000000000000, 0.9042785869254481579, 1.000000000000000000),
 ( 1.000000000000000000, 0.9189749222835162934, 1.000000000000000000),
 ( 1.000000000000000000, 0.9283978182351000363, 1.000000000000000000),
 ( 1.000000000000000000, 0.9376006582765954445, 1.000000000000000000) ) ) 
 REPRESENTATION_ITEM ( '' )  SURFACE ( )  );
#62191=ORIENTED_EDGE ( 'NONE', *, *, #40063, .F. ) ;
#62210=EDGE_LOOP ( 'NONE', ( #7083, #79570, #68262, #64992, #47223 ) ) ;
#62217=CARTESIAN_POINT ( 'NONE',  ( 17.19739463999647100, 1525.960063244516959, 236.2603809477409982 ) ) ;
#62246=AXIS2_PLACEMENT_3D ( 'NONE', #90613, #82772, #91720 ) ;
#62265=CARTESIAN_POINT ( 'NONE',  ( -34.18677586421173231, 1501.977400791986611, 219.7932833225216882 ) ) ;
#62286=FACE_OUTER_BOUND ( 'NONE', #97872, .T. ) ;
#62300=CARTESIAN_POINT ( 'NONE',  ( 20.28160989826444194, 1526.000688113825163, 233.4099348503541762 ) ) ;
#62305=AXIS2_PLACEMENT_3D ( 'NONE', #25182, #101889, #58814 ) ;
#62320=CARTESIAN_POINT ( 'NONE',  ( -16.16632277704758280, 1511.187213306747708, 236.8966194768525497 ) ) ;
#62321=DIRECTION ( 'NONE',  ( -0.9942586961433765858, 0.000000000000000000, -0.1070030146457237041 ) ) ;
#62324=DIRECTION ( 'NONE',  ( 0.000000000000000000, 0.000000000000000000, 1.000000000000000000 ) ) ;
#62335=ORIENTED_EDGE ( 'NONE', *, *, #104907, .T. ) ;
#62337=CARTESIAN_POINT ( 'NONE',  ( 21.83164632205673072, 1524.739915903617430, 184.6225764830850835 ) ) ;
#62339=CARTESIAN_POINT ( 'NONE',  ( 19.91075572344603017, 1526.211523310372058, 184.7300489233186624 ) ) ;
#62368=ORIENTED_EDGE ( 'NONE', *, *, #68117, .F. ) ;
#62378=LINE ( 'NONE', #37148, #67015 ) ;
#62389=AXIS2_PLACEMENT_3D ( 'NONE', #12153, #87783, #1567 ) ;
#62409=AXIS2_PLACEMENT_3D ( 'NONE', #58737, #51436, #33503 ) ;
#62410=ORIENTED_EDGE ( 'NONE', *, *, #104050, .F. ) ;
#62426=EDGE_CURVE ( 'NONE', #89941, #64661, #106307, .T. ) ;
#62445=EDGE_CURVE ( 'NONE', #15037, #85994, #2760, .T. ) ;
#62447=CIRCLE ( 'NONE', #92848, 1.000000000000000888 ) ;
#62461=VECTOR ( 'NONE', #8016, 1000.000000000000000 ) ;
#62463=DIRECTION ( 'NONE',  ( 0.2054769195713296304, -0.000000000000000000, -0.9786619618251631847 ) ) ;
#62472=ORIENTED_EDGE ( 'NONE', *, *, #18763, .F. ) ;
#62489=EDGE_LOOP ( 'NONE', ( #53722, #94319, #16849, #34889 ) ) ;
#62492=VERTEX_POINT ( 'NONE', #82323 ) ;
#62503=EDGE_CURVE ( 'NONE', #56035, #39464, #97652, .T. ) ;
#62516=ADVANCED_FACE ( 'NONE', ( #50936 ), #11154, .F. ) ;
#62519=VECTOR ( 'NONE', #90020, 1000.000000000000000 ) ;
#62522=CARTESIAN_POINT ( 'NONE',  ( -30.24979188206167180, 1524.075000532257263, 222.4742415268079583 ) ) ;
#62530=ORIENTED_EDGE ( 'NONE', *, *, #57642, .F. ) ;
#62533=EDGE_CURVE ( 'NONE', #32820, #56035, #102766, .T. ) ;
#62537=ADVANCED_FACE ( 'NONE', ( #95691 ), #11681, .T. ) ;
#62545=EDGE_LOOP ( 'NONE', ( #87080, #56579, #46652, #75835, #45750, #87273, #92038, #27968 ) ) ;
#62549=CIRCLE ( 'NONE', #21395, 1.000000000000000888 ) ;
#62552=CARTESIAN_POINT ( 'NONE',  ( -21.83863730836054629, 1523.580203803270933, 183.2673815773256649 ) ) ;
#62556=CARTESIAN_POINT ( 'NONE',  ( -30.11977250498258130, 1524.538768545233779, 195.8653401176965758 ) ) ;
#62560=ADVANCED_FACE ( 'NONE', ( #45858 ), #20523, .T. ) ;
#62562=DIRECTION ( 'NONE',  ( 9.367506770274749475E-14, 0.000000000000000000, 1.000000000000000000 ) ) ;
#62564=DIRECTION ( 'NONE',  ( -0.5877852522924673639, 0.000000000000000000, 0.8090169943749514481 ) ) ;
#62567=ORIENTED_EDGE ( 'NONE', *, *, #98706, .F. ) ;
#62573=AXIS2_PLACEMENT_3D ( 'NONE', #47139, #39829, #82926 ) ;
#62575=CARTESIAN_POINT ( 'NONE',  ( -2.478617600774434049, 1524.659802833172535, 242.4723780654675522 ) ) ;
#62578=CARTESIAN_POINT ( 'NONE',  ( 32.78250617288044566, 1512.187213306747481, 218.3079823578266314 ) ) ;
#62586=DIRECTION ( 'NONE',  ( -8.673617379884027583E-16, 0.000000000000000000, 1.000000000000000000 ) ) ;
#62593=ORIENTED_EDGE ( 'NONE', *, *, #4899, .F. ) ;
#62594=ORIENTED_EDGE ( 'NONE', *, *, #265, .F. ) ;
#62600=EDGE_CURVE ( 'NONE', #65949, #35843, #20605, .T. ) ;
#62609=CARTESIAN_POINT ( 'NONE',  ( -20.39147186913014664, 1526.073429442291854, 185.1130304870873715 ) ) ;
#62611=CARTESIAN_POINT ( 'NONE',  ( 19.53786426059039982, 1512.187213306747481, 238.7197124308265188 ) ) ;
#62652=AXIS2_PLACEMENT_3D ( 'NONE', #80028, #107972, #89521 ) ;
#62661=DIRECTION ( 'NONE',  ( 0.5032920991128611021, 0.8641163480519101769, 0.000000000000000000 ) ) ;
#62665=VECTOR ( 'NONE', #6651, 1000.000000000000114 ) ;
#62678=CARTESIAN_POINT ( 'NONE',  ( 2.664543536380612920, 1524.964158026966061, 241.7076164033512100 ) ) ;
#62681=CARTESIAN_POINT ( 'NONE',  ( 22.52214966618161895, 1524.244163922423468, 236.5012798002490513 ) ) ;
#62683=CARTESIAN_POINT ( 'NONE',  ( -20.79738390328759579, 1512.187213306747481, 181.2030061003473236 ) ) ;
#62689=DIRECTION ( 'NONE',  ( 0.9970203751124364633, -0.07713865185920967815, 0.000000000000000000 ) ) ;
#62704=CARTESIAN_POINT ( 'NONE',  ( -2.596261494520250679, 1525.907212628473644, 240.7735774411711986 ) ) ;
#62706=AXIS2_PLACEMENT_3D ( 'NONE', #26632, #84339, #92735 ) ;
#62721=CARTESIAN_POINT ( 'NONE',  ( -32.06248218119481663, 1524.739915903617430, 216.1098515782979064 ) ) ;
#62731=CARTESIAN_POINT ( 'NONE',  ( 2.470955850358427686, 1523.580204110584191, 242.8749759455148478 ) ) ;
#62738=FACE_OUTER_BOUND ( 'NONE', #110355, .T. ) ;
#62745=AXIS2_PLACEMENT_3D ( 'NONE', #15502, #67604, #84919 ) ;
#62749=CARTESIAN_POINT ( 'NONE',  ( 31.14814639454048262, 1525.697947650488459, 201.5095775078352460 ) ) ;
#62752=DIRECTION ( 'NONE',  ( 0.9970203751124365743, 0.07713865185920996959, 0.000000000000000000 ) ) ;
#62772=ORIENTED_EDGE ( 'NONE', *, *, #16455, .T. ) ;
#62774=CARTESIAN_POINT ( 'NONE',  ( 16.66936639845653900, 1523.382868172864164, 237.7608804993219280 ) ) ;
#62776=ORIENTED_EDGE ( 'NONE', *, *, #63941, .T. ) ;
#62777=ORIENTED_EDGE ( 'NONE', *, *, #81579, .F. ) ;
#62783=LINE ( 'NONE', #20169, #43809 ) ;
#62792=ORIENTED_EDGE ( 'NONE', *, *, #41949, .F. ) ;
#62795=ORIENTED_EDGE ( 'NONE', *, *, #5805, .F. ) ;
#62800=CARTESIAN_POINT ( 'NONE',  ( 31.12456774391174719, 1525.960063244516959, 201.1524202391562710 ) ) ;
#62808=DIRECTION ( 'NONE',  ( -9.020562075079389318E-14, 0.000000000000000000, 1.000000000000000000 ) ) ;
#62834=CARTESIAN_POINT ( 'NONE',  ( -16.16632277704758280, 1512.187213306747481, 236.8966194768525497 ) ) ;
#62839=DIRECTION ( 'NONE',  ( 0.000000000000000000, 0.000000000000000000, -1.000000000000000000 ) ) ;
#62848=AXIS2_PLACEMENT_3D ( 'NONE', #19822, #1385, #54029 ) ;
#62855=( BOUNDED_SURFACE ( )  B_SPLINE_SURFACE ( 3, 2, ( 
 ( #42434, #7728, #8269 ),
 ( #44522, #34035, #101771 ),
 ( #25062, #76592, #100677 ),
 ( #109110, #32390, #52930 ) ),
 .UNSPECIFIED., .F., .F., .T. ) 
 B_SPLINE_SURFACE_WITH_KNOTS ( ( 4, 4 ),
 ( 3, 3 ),
 ( 0.000000000000000000, 0.0002960034161023848936 ),
 ( 0.000000000000000000, 1.000000000000000000 ),
 .UNSPECIFIED. ) 
 GEOMETRIC_REPRESENTATION_ITEM ( )  RATIONAL_B_SPLINE_SURFACE ( (
 ( 1.000000000000000000, 0.8072480644198108957, 1.000000000000000000),
 ( 1.000000000000000000, 0.8072480346917760841, 1.000000000000000000),
 ( 1.000000000000000000, 0.8071723757218336459, 1.000000000000000000),
 ( 1.000000000000000000, 0.8070209408750045332, 1.000000000000000000) ) ) 
 REPRESENTATION_ITEM ( '' )  SURFACE ( )  );
#62868=CARTESIAN_POINT ( 'NONE',  ( 33.14208818188970440, 1524.841055067849311, 197.8283574329067562 ) ) ;
#62877=STYLED_ITEM ( 'NONE', ( #107750 ), #13206 ) ;
#62888=DIRECTION ( 'NONE',  ( 0.7414773880254711402, 0.000000000000000000, 0.6709778558543678662 ) ) ;
#62902=CIRCLE ( 'NONE', #66471, 1.000000000000002442 ) ;
#62925=CARTESIAN_POINT ( 'NONE',  ( 17.16388877745072605, 1523.678648413191695, 238.6174304775213386 ) ) ;
#62930=ORIENTED_EDGE ( 'NONE', *, *, #77871, .F. ) ;
#62933=CARTESIAN_POINT ( 'NONE',  ( 32.85805783624308418, 1523.678648413191695, 217.1983043299902931 ) ) ;
#62961=CARTESIAN_POINT ( 'NONE',  ( -2.469061732649111107, 1524.816846803860926, 242.3846597971397330 ) ) ;
#62969=CARTESIAN_POINT ( 'NONE',  ( -17.59789087267267504, 1524.659148609482827, 237.5602248788992767 ) ) ;
#62975=CIRCLE ( 'NONE', #103996, 1.000000000000000666 ) ;
#62988=AXIS2_PLACEMENT_3D ( 'NONE', #74518, #108649, #73959 ) ;
#62997=( BOUNDED_SURFACE ( )  B_SPLINE_SURFACE ( 3, 2, ( 
 ( #35066, #76517, #2049 ),
 ( #25543, #397, #87130 ),
 ( #77630, #93853, #68694 ),
 ( #10419, #44589, #102798 ),
 ( #51886, #86022, #78734 ),
 ( #70365, #9323, #941 ),
 ( #69247, #103355, #94981 ),
 ( #18249, #9865, #80940 ),
 ( #21556, #28330, #29418 ),
 ( #11535, #87700, #3158 ),
 ( #45709, #89882, #12073 ),
 ( #62522, #4770, #88242 ),
 ( #71481, #28885, #70925 ),
 ( #20454, #13152, #4238 ) ),
 .UNSPECIFIED., .F., .F., .T. ) 
 B_SPLINE_SURFACE_WITH_KNOTS ( ( 4, 2, 2, 2, 2, 2, 4 ),
 ( 3, 3 ),
 ( 2.840609691912021617E-17, 0.0009443072508236019296, 0.001416460876235388746, 0.001888614501647175453, 0.002360768127058962378, 0.002832921752470748868, 0.003777229003294322283 ),
 ( 0.000000000000000000, 1.000000000000000000 ),
 .UNSPECIFIED. ) 
 GEOMETRIC_REPRESENTATION_ITEM ( )  RATIONAL_B_SPLINE_SURFACE ( (
 ( 1.000000000000000000, 0.9376006582765943342, 1.000000000000000000),
 ( 1.000000000000000000, 0.9283977714735285325, 1.000000000000000000),
 ( 1.000000000000000000, 0.9189750060481984839, 1.000000000000000000),
 ( 1.000000000000000000, 0.9042792056126492950, 1.000000000000000000),
 ( 1.000000000000000000, 0.8992469033843993875, 1.000000000000000000),
 ( 1.000000000000000000, 0.8891280264681499235, 1.000000000000000000),
 ( 1.000000000000000000, 0.8840337471677424119, 1.000000000000000000),
 ( 1.000000000000000000, 0.8736395124161377979, 1.000000000000000000),
 ( 1.000000000000000000, 0.8683406746559806377, 1.000000000000000000),
 ( 1.000000000000000000, 0.8573361860700633441, 1.000000000000000000),
 ( 1.000000000000000000, 0.8516508399499709281, 1.000000000000000000),
 ( 1.000000000000000000, 0.8340914917059080169, 1.000000000000000000),
 ( 1.000000000000000000, 0.8215597275867274618, 1.000000000000000000),
 ( 1.000000000000000000, 0.8070209408750123048, 1.000000000000000000) ) ) 
 REPRESENTATION_ITEM ( '' )  SURFACE ( )  );
#63000=DIRECTION ( 'NONE',  ( 0.000000000000000000, 0.000000000000000000, 1.000000000000000000 ) ) ;
#63003=CARTESIAN_POINT ( 'NONE',  ( -30.04822308544846621, 1524.382868172804365, 196.4802968571194413 ) ) ;
#63040=CARTESIAN_POINT ( 'NONE',  ( -30.60461244942492343, 1523.621879633028584, 196.4204177336144141 ) ) ;
#63049=CARTESIAN_POINT ( 'NONE',  ( -16.83198307402317440, 1526.000688113712840, 182.3274564795793253 ) ) ;
#63068=B_SPLINE_CURVE_WITH_KNOTS ( 'NONE', 3,
 ( #45063, #88705, #80298, #95440, #18704, #78079, #3613, #52900 ),
 .UNSPECIFIED., .F., .F.,
 ( 4, 2, 2, 4 ),
 ( 6.938893903907227607E-18, 0.001073044933456168909, 0.001609567400184250003, 0.002146089866912330880 ),
 .UNSPECIFIED. ) ;
#63099=CARTESIAN_POINT ( 'NONE',  ( 21.83550407203902211, 1523.678648413191695, 183.2743720722707224 ) ) ;
#63108=CARTESIAN_POINT ( 'NONE',  ( -18.86688640473561307, 1511.187213306747708, 237.4611898188522332 ) ) ;
#63114=CARTESIAN_POINT ( 'NONE',  ( -19.53786426058999481, 1511.187213306747708, 236.7197124308268030 ) ) ;
#63116=CARTESIAN_POINT ( 'NONE',  ( -30.51231035492510557, 1526.382868172863937, 218.1578534183722979 ) ) ;
#63124=CARTESIAN_POINT ( 'NONE',  ( 29.66215386746311466, 1526.345556099435726, 216.9909811895615235 ) ) ;
#63126=CARTESIAN_POINT ( 'NONE',  ( -2.214868538355918570, 1525.730671215507982, 241.5483252278176565 ) ) ;
#63137=EDGE_LOOP ( 'NONE', ( #64683, #58694, #69214, #19576 ) ) ;
#63141=ORIENTED_EDGE ( 'NONE', *, *, #44818, .F. ) ;
#63169=DIRECTION ( 'NONE',  ( -0.1070030146457303932, 0.000000000000000000, 0.9942586961433758086 ) ) ;
#63178=CARTESIAN_POINT ( 'NONE',  ( -0.4151546846821903003, 1522.382868172863937, 244.9330574173806951 ) ) ;
#63185=( BOUNDED_SURFACE ( )  B_SPLINE_SURFACE ( 3, 2, ( 
 ( #104364, #102276, #54005 ),
 ( #70812, #88137, #45594 ),
 ( #17137, #20347, #19228 ),
 ( #88685, #87582, #10871 ),
 ( #10298, #78619, #27661 ),
 ( #33973, #36072, #79735 ),
 ( #51327, #70257, #25556 ),
 ( #79188, #85462, #3044 ),
 ( #2494, #12514, #71366 ),
 ( #28210, #28767, #62969 ),
 ( #80278, #3592, #97626 ),
 ( #20894, #39918, #13036 ),
 ( #48893, #74087, #30405 ),
 ( #30959, #65684, #32064 ) ),
 .UNSPECIFIED., .F., .F., .T. ) 
 B_SPLINE_SURFACE_WITH_KNOTS ( ( 4, 2, 2, 2, 2, 2, 4 ),
 ( 3, 3 ),
 ( 2.300677010014240409E-16, 0.0009443072508238389362, 0.001416460876235643316, 0.001888614501647447805, 0.002360768127059252076, 0.002832921752471056782, 0.003777229003294665759 ),
 ( 0.000000000000000000, 1.000000000000000000 ),
 .UNSPECIFIED. ) 
 GEOMETRIC_REPRESENTATION_ITEM ( )  RATIONAL_B_SPLINE_SURFACE ( (
 ( 1.000000000000000000, 0.9376006582765984421, 1.000000000000000000),
 ( 1.000000000000000000, 0.9283977714665412329, 1.000000000000000000),
 ( 1.000000000000000000, 0.9189750060575127000, 1.000000000000000000),
 ( 1.000000000000000000, 0.9042792056079913543, 1.000000000000000000),
 ( 1.000000000000000000, 0.8992469033838338399, 1.000000000000000000),
 ( 1.000000000000000000, 0.8891280264687103640, 1.000000000000000000),
 ( 1.000000000000000000, 0.8840337471674056813, 1.000000000000000000),
 ( 1.000000000000000000, 0.8736395124164820780, 1.000000000000000000),
 ( 1.000000000000000000, 0.8683406746559402256, 1.000000000000000000),
 ( 1.000000000000000000, 0.8573361860701106396, 1.000000000000000000),
 ( 1.000000000000000000, 0.8516508399497402237, 1.000000000000000000),
 ( 1.000000000000000000, 0.8340914917063595446, 1.000000000000000000),
 ( 1.000000000000000000, 0.8215597275863861793, 1.000000000000000000),
 ( 1.000000000000000000, 0.8070209408750170788, 1.000000000000000000) ) ) 
 REPRESENTATION_ITEM ( '' )  SURFACE ( )  );
#63186=EDGE_CURVE ( 'NONE', #91380, #7480, #62783, .T. ) ;
#63190=ORIENTED_EDGE ( 'NONE', *, *, #74798, .T. ) ;
#63193=CYLINDRICAL_SURFACE ( 'NONE', #8927, 33.13701971169416538 ) ;
#63227=CARTESIAN_POINT ( 'NONE',  ( 3.317974621678423830, 1524.412455883367784, 241.9116897047633756 ) ) ;
#63228=ORIENTED_EDGE ( 'NONE', *, *, #23624, .F. ) ;
#63231=CARTESIAN_POINT ( 'NONE',  ( 22.01290455779448152, 1522.906363951597314, 235.3651141902282689 ) ) ;
#63236=DIRECTION ( 'NONE',  ( -0.3090169943749515591, 0.000000000000000000, -0.9510565162951523099 ) ) ;
#63246=DIRECTION ( 'NONE',  ( -0.2054769195713296304, 0.000000000000000000, -0.9786619618251631847 ) ) ;
#63249=CARTESIAN_POINT ( 'NONE',  ( -16.53175237173161705, 1526.069472839382115, 235.9420435486929364 ) ) ;
#63256=CARTESIAN_POINT ( 'NONE',  ( 32.36513376976810719, 1523.847233649538339, 216.1093208013068079 ) ) ;
#63261=CARTESIAN_POINT ( 'NONE',  ( -31.62138935264889028, 1525.231887713368678, 216.6630328221493187 ) ) ;
#63312=EDGE_CURVE ( 'NONE', #17148, #94625, #81357, .T. ) ;
#63314=ORIENTED_EDGE ( 'NONE', *, *, #89359, .F. ) ;
#63335=ORIENTED_EDGE ( 'NONE', *, *, #84890, .F. ) ;
#63337=CARTESIAN_POINT ( 'NONE',  ( 0.4681535437661810684, 1524.397344074319335, 173.8154889443022171 ) ) ;
#63345=DIRECTION ( 'NONE',  ( 0.000000000000000000, 0.000000000000000000, 1.000000000000000000 ) ) ;
#63355=ORIENTED_EDGE ( 'NONE', *, *, #67067, .F. ) ;
#63379=CARTESIAN_POINT ( 'NONE',  ( -22.14913372575983175, 1525.402221411349728, 235.6690521037287454 ) ) ;
#63394=CARTESIAN_POINT ( 'NONE',  ( -22.03465957474533354, 1501.977400791986611, 235.4136513321633117 ) ) ;
#63401=CARTESIAN_POINT ( 'NONE',  ( 31.69312280309565821, 1525.713797967456912, 196.3032712708385077 ) ) ;
#63404=DIRECTION ( 'NONE',  ( -0.000000000000000000, -1.000000000000000000, -0.000000000000000000 ) ) ;
#63406=CARTESIAN_POINT ( 'NONE',  ( -30.36939524941901070, 1525.506916460679349, 196.8236333301088337 ) ) ;
#63407=CARTESIAN_POINT ( 'NONE',  ( -16.66701395081226877, 1523.530870145309109, 237.7590812510466947 ) ) ;
#63414=CARTESIAN_POINT ( 'NONE',  ( 1.191524307911310254, 1526.382868172864164, 179.0083900503168479 ) ) ;
#63420=CARTESIAN_POINT ( 'NONE',  ( 16.66936639845630097, 1523.382868172864164, 180.4828114240739296 ) ) ;
#63430=DIRECTION ( 'NONE',  ( 0.000000000000000000, 0.000000000000000000, 1.000000000000000000 ) ) ;
#63441=VERTEX_POINT ( 'NONE', #13406 ) ;
#63453=DIRECTION ( 'NONE',  ( -0.7414773880254760252, 0.000000000000000000, -0.6709778558543624261 ) ) ;
#63477=VECTOR ( 'NONE', #63453, 1000.000000000000114 ) ;
#63478=ORIENTED_EDGE ( 'NONE', *, *, #54969, .F. ) ;
#63483=VERTEX_POINT ( 'NONE', #25118 ) ;
#63494=CARTESIAN_POINT ( 'NONE',  ( -30.31940284292399213, 1512.187213306747481, 222.4933038710547919 ) ) ;
#63496=EDGE_CURVE ( 'NONE', #15990, #81018, #83940, .T. ) ;
#63505=PLANE ( 'NONE',  #88680 ) ;
#63507=EDGE_LOOP ( 'NONE', ( #88645, #93266, #19863, #61591 ) ) ;
#63513=FACE_OUTER_BOUND ( 'NONE', #100026, .T. ) ;
#63523=VECTOR ( 'NONE', #32061, 1000.000000000000000 ) ;
#63528=B_SPLINE_CURVE_WITH_KNOTS ( 'NONE', 3,
 ( #19944, #87730, #62552, #104510 ),
 .UNSPECIFIED., .F., .F.,
 ( 4, 4 ),
 ( 0.000000000000000000, 0.0002960034161023848394 ),
 .UNSPECIFIED. ) ;
#63546=CIRCLE ( 'NONE', #45639, 1.000000000000001554 ) ;
#63577=DIRECTION ( 'NONE',  ( 0.8090169943749465631, 0.000000000000000000, -0.5877852522924742473 ) ) ;
#63585=FACE_OUTER_BOUND ( 'NONE', #27596, .T. ) ;
#63601=EDGE_CURVE ( 'NONE', #23046, #5040, #4489, .T. ) ;
#63627=DIRECTION ( 'NONE',  ( 0.9510565162951566398, 0.000000000000000000, 0.3090169943749382919 ) ) ;
#63659=DIRECTION ( 'NONE',  ( -9.714451465470110893E-14, 0.000000000000000000, 1.000000000000000000 ) ) ;
#63661=CARTESIAN_POINT ( 'NONE',  ( -2.485125933802709852, 1524.547873515805350, 242.5340162392059540 ) ) ;
#63675=EDGE_CURVE ( 'NONE', #73175, #31615, #64806, .T. ) ;
#63681=DIRECTION ( 'NONE',  ( 0.6665120492724808665, 0.000000000000000000, 0.7454942576402571186 ) ) ;
#63694=CARTESIAN_POINT ( 'NONE',  ( 33.17484411121986909, 1525.713797967456685, 200.8635405475196762 ) ) ;
#63707=CARTESIAN_POINT ( 'NONE',  ( -30.24842679174809490, 1524.082582765195411, 222.4736128011820142 ) ) ;
#63731=ORIENTED_EDGE ( 'NONE', *, *, #88704, .F. ) ;
#63736=CARTESIAN_POINT ( 'NONE',  ( -19.37374569213963582, 1524.382868172863937, 183.8768763279542213 ) ) ;
#63759=ORIENTED_EDGE ( 'NONE', *, *, #37278, .T. ) ;
#63766=LINE ( 'NONE', #47504, #99620 ) ;
#63774=CARTESIAN_POINT ( 'NONE',  ( -30.90487439922565116, 1525.907212628473644, 201.8101144455181952 ) ) ;
#63776=CARTESIAN_POINT ( 'NONE',  ( -3.350338079455601026, 1523.604703353109699, 176.1628856388066708 ) ) ;
#63780=EDGE_CURVE ( 'NONE', #32555, #31391, #4267, .T. ) ;
#63784=ADVANCED_FACE ( 'NONE', ( #91110 ), #23347, .T. ) ;
#63785=( BOUNDED_SURFACE ( )  B_SPLINE_SURFACE ( 3, 2, ( 
 ( #80910, #72517, #106645 ),
 ( #55729, #54087, #55178 ),
 ( #79820, #105007, #70337 ),
 ( #104449, #29385, #11506 ),
 ( #71452, #12600, #46778 ),
 ( #64127, #98248, #21518 ),
 ( #13121, #97155, #54630 ),
 ( #88763, #12046, #46229 ),
 ( #80362, #84604, #65223 ),
 ( #107757, #67835, #7896 ),
 ( #17375, #39454, #79 ),
 ( #59437, #90386, #59987 ),
 ( #31040, #5296, #81988 ),
 ( #30493, #85707, #40000 ) ),
 .UNSPECIFIED., .F., .F., .F. ) 
 B_SPLINE_SURFACE_WITH_KNOTS ( ( 4, 2, 2, 2, 2, 2, 4 ),
 ( 3, 3 ),
 ( 2.412349833780247366E-16, 0.0009443072508238468509, 0.001416460876235649605, 0.001888614501647452575, 0.002360768127059255546, 0.002832921752471058083, 0.003777229003294664024 ),
 ( 0.000000000000000000, 1.000000000000000000 ),
 .UNSPECIFIED. ) 
 GEOMETRIC_REPRESENTATION_ITEM ( )  RATIONAL_B_SPLINE_SURFACE ( (
 ( 1.000000000000000000, 0.9376006582765971098, 1.000000000000000000),
 ( 1.000000000000000000, 0.9283977714666437064, 1.000000000000000000),
 ( 1.000000000000000000, 0.9189750060573711465, 1.000000000000000000),
 ( 1.000000000000000000, 0.9042792056080602991, 1.000000000000000000),
 ( 1.000000000000000000, 0.8992469033884697982, 1.000000000000000000),
 ( 1.000000000000000000, 0.8891280264640721853, 1.000000000000000000),
 ( 1.000000000000000000, 0.8840337471674194481, 1.000000000000000000),
 ( 1.000000000000000000, 0.8736395124164607617, 1.000000000000000000),
 ( 1.000000000000000000, 0.8683406746558937073, 1.000000000000000000),
 ( 1.000000000000000000, 0.8573361860701524950, 1.000000000000000000),
 ( 1.000000000000000000, 0.8516508399495845705, 1.000000000000000000),
 ( 1.000000000000000000, 0.8340914917066767353, 1.000000000000000000),
 ( 1.000000000000000000, 0.8215597275861534765, 1.000000000000000000),
 ( 1.000000000000000000, 0.8070209408750069757, 1.000000000000000000) ) ) 
 REPRESENTATION_ITEM ( '' )  SURFACE ( )  );
#63792=VERTEX_POINT ( 'NONE', #78599 ) ;
#63797=EDGE_LOOP ( 'NONE', ( #70368, #101623, #70479, #102254 ) ) ;
#63814=CIRCLE ( 'NONE', #71025, 2.000000000000001776 ) ;
#63816=ORIENTED_EDGE ( 'NONE', *, *, #41240, .F. ) ;
#63818=CARTESIAN_POINT ( 'NONE',  ( 18.15646965371266575, 1522.906363951597314, 238.1669781545271860 ) ) ;
#63819=EDGE_CURVE ( 'NONE', #82691, #96612, #106244, .T. ) ;
#63826=CARTESIAN_POINT ( 'NONE',  ( 32.06248218118899018, 1524.739915903631754, 202.1338403451020440 ) ) ;
#63832=EDGE_CURVE ( 'NONE', #104688, #50508, #56148, .T. ) ;
#63868=EDGE_CURVE ( 'NONE', #98871, #65751, #6292, .T. ) ;
#63871=ORIENTED_EDGE ( 'NONE', *, *, #29636, .F. ) ;
#63875=VERTEX_POINT ( 'NONE', #91945 ) ;
#63876=CARTESIAN_POINT ( 'NONE',  ( 2.534335827540430852, 1523.982201850120191, 175.6705872193752214 ) ) ;
#63913=CARTESIAN_POINT ( 'NONE',  ( -22.03465957474530157, 1522.382868172863937, 235.4136513321633117 ) ) ;
#63914=B_SPLINE_CURVE_WITH_KNOTS ( 'NONE', 3,
 ( #34047, #14476, #109121, #82794, #32400, #66583, #100686, #23970, #6089, #92294 ),
 .UNSPECIFIED., .F., .F.,
 ( 4, 2, 2, 2, 4 ),
 ( 0.000000000000000000, 0.0007189769279725863283, 0.001437953855945172657, 0.002156930783917758877, 0.002875907711890345313 ),
 .UNSPECIFIED. ) ;
#63930=EDGE_CURVE ( 'NONE', #106529, #85718, #86853, .T. ) ;
#63941=EDGE_CURVE ( 'NONE', #8029, #80761, #76216, .T. ) ;
#63942=CARTESIAN_POINT ( 'NONE',  ( 21.05711716160336522, 1526.748660780343471, 233.6123052680174510 ) ) ;
#63946=DIRECTION ( 'NONE',  ( 0.000000000000000000, 1.000000000000000000, 0.000000000000000000 ) ) ;
#63954=CARTESIAN_POINT ( 'NONE',  ( 1.961418762358043022, 1526.143142182266047, 177.8224660300663515 ) ) ;
#63958=CARTESIAN_POINT ( 'NONE',  ( -20.92767404034536938, 1512.187213306747481, 182.8548762971666406 ) ) ;
#63981=AXIS2_PLACEMENT_3D ( 'NONE', #51238, #8666, #42844 ) ;
#64030=CARTESIAN_POINT ( 'NONE',  ( -21.30823923614832083, 1524.382868172804365, 184.4507411017320919 ) ) ;
#64033=AXIS2_PLACEMENT_3D ( 'NONE', #30320, #72893, #21891 ) ;
#64040=CARTESIAN_POINT ( 'NONE',  ( 29.55269881708366597, 1525.821544997590536, 221.1141083160992764 ) ) ;
#64042=VERTEX_POINT ( 'NONE', #49826 ) ;
#64043=CARTESIAN_POINT ( 'NONE',  ( -1.689251544523377779, 1526.344110814223541, 178.4720708657796138 ) ) ;
#64045=FACE_OUTER_BOUND ( 'NONE', #41568, .T. ) ;
#64048=CARTESIAN_POINT ( 'NONE',  ( 16.77192111137855690, 1526.333389947941896, 183.3307103475321185 ) ) ;
#64050=CARTESIAN_POINT ( 'NONE',  ( 18.02257621027576917, 1524.382868172863937, 182.8951942368371988 ) ) ;
#64068=CARTESIAN_POINT ( 'NONE',  ( 20.70484064406359437, 1525.907212628473872, 185.0411015109854134 ) ) ;
#64070=CARTESIAN_POINT ( 'NONE',  ( -32.85805783624297760, 1523.678648413191695, 217.1983043299907763 ) ) ;
#64083=CARTESIAN_POINT ( 'NONE',  ( 31.11295621079038654, 1525.790286462508675, 216.3449408200586106 ) ) ;
#64091=CARTESIAN_POINT ( 'NONE',  ( -19.29374783221095768, 1526.349684470114653, 233.1524122426512236 ) ) ;
#64096=TOROIDAL_SURFACE ( 'NONE', #92676, 1.000000000000000000, 1.000000000000000000 ) ;
#64107=EDGE_LOOP ( 'NONE', ( #33669, #30588, #16970, #55495 ) ) ;
#64117=CARTESIAN_POINT ( 'NONE',  ( -30.31940284289330734, 1523.456924617338245, 195.7503880522716315 ) ) ;
#64126=DIRECTION ( 'NONE',  ( -0.5877852522924629231, 0.000000000000000000, 0.8090169943749548898 ) ) ;
#64127=CARTESIAN_POINT ( 'NONE',  ( 21.59934095315572478, 1525.137881624885267, 233.5034356062079155 ) ) ;
#64131=FACE_OUTER_BOUND ( 'NONE', #36794, .T. ) ;
#64143=( BOUNDED_CURVE ( )  B_SPLINE_CURVE ( 3, ( #70957, #53030, #2084, #88273 ),
 .UNSPECIFIED., .F., .T. ) 
 B_SPLINE_CURVE_WITH_KNOTS ( ( 4, 4 ),
 ( 4.712388980384689674, 6.283185307179586232 ),
 .UNSPECIFIED. ) 
 CURVE ( )  GEOMETRIC_REPRESENTATION_ITEM ( )  RATIONAL_B_SPLINE_CURVE ( ( 1.000000000000000000, 0.8047378541243649375, 0.8047378541243649375, 1.000000000000000000 ) ) 
 REPRESENTATION_ITEM ( '' )  );
#64168=ORIENTED_EDGE ( 'NONE', *, *, #81541, .T. ) ;
#64178=FACE_OUTER_BOUND ( 'NONE', #56870, .T. ) ;
#64196=CARTESIAN_POINT ( 'NONE',  ( 2.534335827540424191, 1523.982201850120191, 242.5731047040208068 ) ) ;
#64204=CARTESIAN_POINT ( 'NONE',  ( -2.472529913803020563, 1523.678648413191695, 242.8674788698241400 ) ) ;
#64207=DIRECTION ( 'NONE',  ( -0.1010290445074239624, 0.000000000000000000, 0.9948834766775036531 ) ) ;
#64211=ADVANCED_FACE ( 'NONE', ( #72161 ), #45295, .T. ) ;
#64229=CARTESIAN_POINT ( 'NONE',  ( 2.470168521978398424, 1523.382868172864164, 242.8787258963054683 ) ) ;
#64233=CARTESIAN_POINT ( 'NONE',  ( -2.057041824809119568, 1523.342713519622521, 244.8463988825372724 ) ) ;
#64239=CARTESIAN_POINT ( 'NONE',  ( 30.51231035492520149, 1526.382868172863937, 200.0858385050239008 ) ) ;
#64242=ORIENTED_EDGE ( 'NONE', *, *, #75729, .T. ) ;
#64247=DIRECTION ( 'NONE',  ( 0.1070030146457371656, 0.000000000000000000, -0.9942586961433751425 ) ) ;
#64250=DIRECTION ( 'NONE',  ( 0.000000000000000000, 0.000000000000000000, 1.000000000000000000 ) ) ;
#64264=VECTOR ( 'NONE', #9195, 999.9999999999998863 ) ;
#64271=AXIS2_PLACEMENT_3D ( 'NONE', #17912, #75656, #50458 ) ;
#64285=AXIS2_PLACEMENT_3D ( 'NONE', #107815, #28912, #54687 ) ;
#64289=CIRCLE ( 'NONE', #28462, 2.000000000000003109 ) ;
#64309=CIRCLE ( 'NONE', #14162, 0.9999999999999326095 ) ;
#64316=DIRECTION ( 'NONE',  ( -0.9942586961433764747, 2.969930264099993005E-15, -0.1070030146457249115 ) ) ;
#64329=LINE ( 'NONE', #4943, #90789 ) ;
#64333=CARTESIAN_POINT ( 'NONE',  ( -16.73628186595805545, 1526.382868172864164, 234.1845039693045862 ) ) ;
#64350=EDGE_LOOP ( 'NONE', ( #51796, #33402, #62795, #30845, #110056 ) ) ;
#64352=CARTESIAN_POINT ( 'NONE',  ( 32.97913964219430483, 1511.187213306747708, 197.9697544589745632 ) ) ;
#64356=DIRECTION ( 'NONE',  ( 0.3090169943749446757, -0.000000000000000000, -0.9510565162951544194 ) ) ;
#64364=CARTESIAN_POINT ( 'NONE',  ( 1.491506560153233352, 1512.187213306747481, 242.6732489767341576 ) ) ;
#64367=CARTESIAN_POINT ( 'NONE',  ( 19.37774363895692886, 1525.878013734321712, 236.8539400710499194 ) ) ;
#64370=CARTESIAN_POINT ( 'NONE',  ( 0.000000000000000000, 1518.913060387330006, 209.1218459616979999 ) ) ;
#64389=ORIENTED_EDGE ( 'NONE', *, *, #81012, .T. ) ;
#64399=EDGE_LOOP ( 'NONE', ( #65660, #69780, #37277, #91761 ) ) ;
#64421=EDGE_CURVE ( 'NONE', #108102, #82322, #29030, .T. ) ;
#64424=ORIENTED_EDGE ( 'NONE', *, *, #33659, .T. ) ;
#64433=AXIS2_PLACEMENT_3D ( 'NONE', #45130, #91519, #89312 ) ;
#64439=CARTESIAN_POINT ( 'NONE',  ( 29.53441971554831724, 1525.651286436460850, 196.5125197345233232 ) ) ;
#64472=EDGE_CURVE ( 'NONE', #92713, #61077, #31103, .T. ) ;
#64506=CARTESIAN_POINT ( 'NONE',  ( -0.4151546846821903003, 1512.187213306747481, 173.3106345060153046 ) ) ;
#64519=DIRECTION ( 'NONE',  ( 0.000000000000000000, 0.000000000000000000, 1.000000000000000000 ) ) ;
#64530=ORIENTED_EDGE ( 'NONE', *, *, #52921, .F. ) ;
#64531=ORIENTED_EDGE ( 'NONE', *, *, #61831, .T. ) ;
#64547=CARTESIAN_POINT ( 'NONE',  ( -31.23437356469455040, 1518.913060387330006, 195.3468678195118287 ) ) ;
#64568=VERTEX_POINT ( 'NONE', #95912 ) ;
#64581=DIRECTION ( 'NONE',  ( 0.5369043659965772042, -0.4884709562386981840, -0.6878443331779838799 ) ) ;
#64582=CARTESIAN_POINT ( 'NONE',  ( -22.52214966618224778, 1524.244163922423695, 181.7424121231434810 ) ) ;
#64607=ORIENTED_EDGE ( 'NONE', *, *, #110208, .F. ) ;
#64611=CARTESIAN_POINT ( 'NONE',  ( 32.02808312589916540, 1512.187213306747481, 196.2787714533495489 ) ) ;
#64621=DIRECTION ( 'NONE',  ( -0.000000000000000000, -1.000000000000000000, -0.000000000000000000 ) ) ;
#64634=CARTESIAN_POINT ( 'NONE',  ( 31.80537271888414352, 1525.137881624894817, 216.1511922624794693 ) ) ;
#64643=DIRECTION ( 'NONE',  ( 0.000000000000000000, 0.000000000000000000, -1.000000000000000000 ) ) ;
#64649=DIRECTION ( 'NONE',  ( 0.9125304618754024322, 0.000000000000000000, 0.4090087482554191078 ) ) ;
#64661=VERTEX_POINT ( 'NONE', #19748 ) ;
#64675=( LENGTH_UNIT ( ) NAMED_UNIT ( * ) SI_UNIT ( .MILLI., .METRE. ) );
#64683=ORIENTED_EDGE ( 'NONE', *, *, #48105, .T. ) ;
#64684=ORIENTED_EDGE ( 'NONE', *, *, #63780, .T. ) ;
#64704=EDGE_CURVE ( 'NONE', #20210, #37975, #57981, .T. ) ;
#64705=CARTESIAN_POINT ( 'NONE',  ( 2.225547318884175230, 1525.712830164893376, 176.6706926612863811 ) ) ;
#64706=ORIENTED_EDGE ( 'NONE', *, *, #59060, .F. ) ;
#64718=CARTESIAN_POINT ( 'NONE',  ( 28.27139721233031722, 1526.382868172864164, 198.6830693683572235 ) ) ;
#64725=EDGE_LOOP ( 'NONE', ( #62410, #42075, #103105 ) ) ;
#64729=CARTESIAN_POINT ( 'NONE',  ( 30.60461244942474224, 1523.621879633028811, 196.4204177336139878 ) ) ;
#64738=CARTESIAN_POINT ( 'NONE',  ( 30.79697748855865669, 1526.178928173327449, 221.8439766881941466 ) ) ;
#64739=EDGE_LOOP ( 'NONE', ( #37789, #99793, #89039, #3821, #92079 ) ) ;
#64747=EDGE_CURVE ( 'NONE', #55319, #31132, #107988, .T. ) ;
#64770=CARTESIAN_POINT ( 'NONE',  ( -33.93019615848939452, 1512.187213306747481, 220.5829544587966211 ) ) ;
#64777=ORIENTED_EDGE ( 'NONE', *, *, #105628, .F. ) ;
#64779=CARTESIAN_POINT ( 'NONE',  ( -16.56942828594061723, 1526.189892541618974, 235.5982591281702980 ) ) ;
#64780=ORIENTED_EDGE ( 'NONE', *, *, #5619, .F. ) ;
#64789=B_SPLINE_CURVE_WITH_KNOTS ( 'NONE', 3,
 ( #43644, #54275, #105207, #35794, #95698, #52606, #95148, #18408 ),
 .UNSPECIFIED., .F., .F.,
 ( 4, 2, 2, 4 ),
 ( 3.103167691559091397E-17, 0.001073044933456083041, 0.001609567400184111442, 0.002146089866912140060 ),
 .UNSPECIFIED. ) ;
#64801=ORIENTED_EDGE ( 'NONE', *, *, #88419, .T. ) ;
#64806=( BOUNDED_CURVE ( )  B_SPLINE_CURVE ( 3, ( #35754, #78303, #88909, #70492 ),
 .UNSPECIFIED., .F., .T. ) 
 B_SPLINE_CURVE_WITH_KNOTS ( ( 4, 4 ),
 ( 0.000000000000000000, 0.7048113239778038830 ),
 .UNSPECIFIED. ) 
 CURVE ( )  GEOMETRIC_REPRESENTATION_ITEM ( )  RATIONAL_B_SPLINE_CURVE ( ( 1.000000000000000000, 0.9590300661663093695, 0.9590300661663093695, 1.000000000000000000 ) ) 
 REPRESENTATION_ITEM ( '' )  );
#64809=AXIS2_PLACEMENT_3D ( 'NONE', #105788, #44784, #37466 ) ;
#64825=CIRCLE ( 'NONE', #88071, 1.999999999999995559 ) ;
#64839=CARTESIAN_POINT ( 'NONE',  ( -29.16136750932859556, 1526.143142182266047, 220.6593063691003920 ) ) ;
#64841=DIRECTION ( 'NONE',  ( -0.4978433412588729179, 0.000000000000000000, -0.8672669759446635096 ) ) ;
#64855=LINE ( 'NONE', #12208, #80644 ) ;
#64856=EDGE_CURVE ( 'NONE', #17784, #28004, #81356, .T. ) ;
#64862=CARTESIAN_POINT ( 'NONE',  ( 31.23437356469446868, 1518.913060387330006, 222.8968241038843701 ) ) ;
#64865=DIRECTION ( 'NONE',  ( 0.000000000000000000, 1.000000000000000000, 0.000000000000000000 ) ) ;
#64885=CARTESIAN_POINT ( 'NONE',  ( -0.4151546846821903003, 1501.977400791986611, 173.3106345060153046 ) ) ;
#64904=ORIENTED_EDGE ( 'NONE', *, *, #37734, .F. ) ;
#64916=DIRECTION ( 'NONE',  ( -0.2054769195713180285, 0.000000000000000000, 0.9786619618251657382 ) ) ;
#64917=ORIENTED_EDGE ( 'NONE', *, *, #38900, .T. ) ;
#64921=FACE_OUTER_BOUND ( 'NONE', #71054, .T. ) ;
#64949=CARTESIAN_POINT ( 'NONE',  ( 16.66701395081591031, 1523.530870145310928, 237.7590812510444493 ) ) ;
#64951=ORIENTED_EDGE ( 'NONE', *, *, #56640, .T. ) ;
#64959=CARTESIAN_POINT ( 'NONE',  ( 16.81049281787637639, 1526.143142182265819, 235.5964692618685774 ) ) ;
#64992=ORIENTED_EDGE ( 'NONE', *, *, #870, .F. ) ;
#65001=AXIS2_PLACEMENT_3D ( 'NONE', #106741, #4307, #21618 ) ;
#65003=CARTESIAN_POINT ( 'NONE',  ( -21.13130013988097389, 1524.397344074317971, 237.4101150494072954 ) ) ;
#65004=CARTESIAN_POINT ( 'NONE',  ( 0.000000000000000000, 1522.382868172863937, 177.3106345060153046 ) ) ;
#65012=FACE_OUTER_BOUND ( 'NONE', #77057, .T. ) ;
#65022=CARTESIAN_POINT ( 'NONE',  ( -16.52275002910772272, 1525.042412244735260, 180.9740555130105122 ) ) ;
#65027=CARTESIAN_POINT ( 'NONE',  ( -0.4151546846821903003, 1501.977400791986611, 175.3106345060153046 ) ) ;
#65031=CARTESIAN_POINT ( 'NONE',  ( 33.36586802512179162, 1512.187213306747481, 216.3367586934468818 ) ) ;
#65036=CARTESIAN_POINT ( 'NONE',  ( 1.912903644477788934, 1526.104292489128966, 177.3592290664105349 ) ) ;
#65041=EDGE_CURVE ( 'NONE', #11721, #88474, #84726, .T. ) ;
#65046=DIRECTION ( 'NONE',  ( 1.000000000000000000, -0.000000000000000000, -0.000000000000000000 ) ) ;
#65051=EDGE_CURVE ( 'NONE', #33454, #67358, #68692, .T. ) ;
#65058=CARTESIAN_POINT ( 'NONE',  ( 16.50400130224771544, 1525.907212628473644, 236.2546788475581820 ) ) ;
#65064=DIRECTION ( 'NONE',  ( 0.9510565162951518658, 0.000000000000000000, -0.3090169943749528914 ) ) ;
#65082=EDGE_CURVE ( 'NONE', #74525, #110178, #69291, .T. ) ;
#65090=EDGE_CURVE ( 'NONE', #42516, #55064, #99078, .T. ) ;
#65107=ORIENTED_EDGE ( 'NONE', *, *, #26227, .F. ) ;
#65119=DIRECTION ( 'NONE',  ( 0.6709778558543747495, 0.000000000000000000, 0.7414773880254650340 ) ) ;
#65120=CARTESIAN_POINT ( 'NONE',  ( -19.37374569213963227, 1526.382868172863937, 183.8768763279542213 ) ) ;
#65142=EDGE_CURVE ( 'NONE', #106529, #74589, #99027, .T. ) ;
#65151=DIRECTION ( 'NONE',  ( 0.9942586961433758086, -0.000000000000000000, 0.1070030146457303932 ) ) ;
#65162=TOROIDAL_SURFACE ( 'NONE', #18606, 2.000000000000000000, 1.000000000000000000 ) ;
#65171=CARTESIAN_POINT ( 'NONE',  ( -31.26701538686457127, 1523.919934424249959, 221.8945625893618683 ) ) ;
#65172=AXIS2_PLACEMENT_3D ( 'NONE', #21356, #22453, #63430 ) ;
#65176=FACE_OUTER_BOUND ( 'NONE', #84001, .T. ) ;
#65180=EDGE_CURVE ( 'NONE', #50505, #92786, #23888, .T. ) ;
#65190=CARTESIAN_POINT ( 'NONE',  ( 16.64711227027034113, 1523.843271061947917, 237.7438619119893133 ) ) ;
#65223=CARTESIAN_POINT ( 'NONE',  ( 21.51513853577893798, 1524.871836253796118, 234.5521809742263883 ) ) ;
#65233=ORIENTED_EDGE ( 'NONE', *, *, #65365, .T. ) ;
#65248=AXIS2_PLACEMENT_3D ( 'NONE', #94021, #53723, #69969 ) ;
#65258=CARTESIAN_POINT ( 'NONE',  ( 28.54794148641478913, 1526.382868172864164, 198.4382598900853623 ) ) ;
#65274=EDGE_CURVE ( 'NONE', #50057, #73846, #9764, .T. ) ;
#65277=DIRECTION ( 'NONE',  ( 0.000000000000000000, 1.000000000000000000, 0.000000000000000000 ) ) ;
#65278=CARTESIAN_POINT ( 'NONE',  ( 30.29630067237538071, 1526.329757971584968, 221.7900933993806802 ) ) ;
#65283=DIRECTION ( 'NONE',  ( -0.000000000000000000, -1.000000000000000000, -0.000000000000000000 ) ) ;
#65296=AXIS2_PLACEMENT_3D ( 'NONE', #48274, #66188, #82418 ) ;
#65301=DIRECTION ( 'NONE',  ( -0.000000000000000000, -1.000000000000000000, -0.000000000000000000 ) ) ;
#65322=DIRECTION ( 'NONE',  ( 0.000000000000000000, 0.000000000000000000, 1.000000000000000000 ) ) ;
#65323=CARTESIAN_POINT ( 'NONE',  ( -19.92151515271962126, 1526.208281990536307, 233.5199663060418516 ) ) ;
#65331=CARTESIAN_POINT ( 'NONE',  ( -18.19590854888121356, 1512.187213306747481, 238.2026672068777202 ) ) ;
#65365=EDGE_CURVE ( 'NONE', #59464, #61894, #16839, .T. ) ;
#65376=CIRCLE ( 'NONE', #20646, 1.000000000000000888 ) ;
#65378=CARTESIAN_POINT ( 'NONE',  ( -33.36586802512168504, 1512.187213306747481, 216.3367586934473366 ) ) ;
#65381=EDGE_LOOP ( 'NONE', ( #65657, #67713, #109060, #108025 ) ) ;
#65383=CARTESIAN_POINT ( 'NONE',  ( 17.84338787571943641, 1512.187213306747481, 237.8836641337660467 ) ) ;
#65385=CARTESIAN_POINT ( 'NONE',  ( 21.84020450222037724, 1512.187213306747481, 183.2638850454218016 ) ) ;
#65390=CARTESIAN_POINT ( 'NONE',  ( -17.17241001986462123, 1512.187213306747481, 238.6251415217917895 ) ) ;
#65400=CARTESIAN_POINT ( 'NONE',  ( -17.83486663330464950, 1523.678648413191695, 237.8759530894961074 ) ) ;
#65407=DIRECTION ( 'NONE',  ( 0.5877852522924820189, 0.000000000000000000, 0.8090169943749410120 ) ) ;
#65416=CARTESIAN_POINT ( 'NONE',  ( -31.23437356469425907, 1518.913060387330006, 222.8968241038848248 ) ) ;
#65433=DIRECTION ( 'NONE',  ( -3.552713678800500929E-15, 0.000000000000000000, 1.000000000000000000 ) ) ;
#65438=CARTESIAN_POINT ( 'NONE',  ( -30.61115703707795177, 1523.542365884050923, 221.8239785241903235 ) ) ;
#65505=VERTEX_POINT ( 'NONE', #8562 ) ;
#65525=ORIENTED_EDGE ( 'NONE', *, *, #27002, .F. ) ;
#65549=ORIENTED_EDGE ( 'NONE', *, *, #108376, .T. ) ;
#65551=CARTESIAN_POINT ( 'NONE',  ( 16.51112239071560950, 1525.159177407155994, 237.1918628954884127 ) ) ;
#65555=CARTESIAN_POINT ( 'NONE',  ( -31.32995031131208918, 1523.678648413191695, 196.3423562208917872 ) ) ;
#65559=CARTESIAN_POINT ( 'NONE',  ( -31.12456774391181469, 1525.960063244516959, 201.1524202391567258 ) ) ;
#65573=CARTESIAN_POINT ( 'NONE',  ( -32.02808312589930040, 1512.187213306747481, 198.2787714533499752 ) ) ;
#65579=CARTESIAN_POINT ( 'NONE',  ( -17.26794000855262112, 1525.730671215512757, 181.5864061050555165 ) ) ;
#65583=DIRECTION ( 'NONE',  ( 0.000000000000000000, -1.000000000000000000, 0.000000000000000000 ) ) ;
#65590=CARTESIAN_POINT ( 'NONE',  ( -18.10570579381957401, 1525.713797967457140, 238.1210409130250127 ) ) ;
#65606=CYLINDRICAL_SURFACE ( 'NONE', #82055, 1.000000000000001332 ) ;
#65637=EDGE_LOOP ( 'NONE', ( #14877, #102635, #30772 ) ) ;
#65647=CIRCLE ( 'NONE', #97757, 0.9999999999999886757 ) ;
#65652=DIRECTION ( 'NONE',  ( -0.9786619618251657382, 0.000000000000000000, -0.2054769195713184449 ) ) ;
#65657=ORIENTED_EDGE ( 'NONE', *, *, #16601, .T. ) ;
#65660=ORIENTED_EDGE ( 'NONE', *, *, #12235, .T. ) ;
#65662=DIRECTION ( 'NONE',  ( -0.000000000000000000, -1.000000000000000000, -0.000000000000000000 ) ) ;
#65668=CARTESIAN_POINT ( 'NONE',  ( -18.51436573157338117, 1512.187213306747481, 237.1421867457408723 ) ) ;
#65673=AXIS2_PLACEMENT_3D ( 'NONE', #28608, #36449, #62808 ) ;
#65676=CARTESIAN_POINT ( 'NONE',  ( 18.66420869458043796, 1526.382868172863937, 185.4599087859680537 ) ) ;
#65681=CARTESIAN_POINT ( 'NONE',  ( -20.71343476517554905, 1512.187213306747481, 179.9059455038197086 ) ) ;
#65684=CARTESIAN_POINT ( 'NONE',  ( -17.29393938232436057, 1523.621879633028811, 237.3864571009502811 ) ) ;
#65697=VERTEX_POINT ( 'NONE', #16937 ) ;
#65725=CARTESIAN_POINT ( 'NONE',  ( 31.97162612954836192, 1524.678541297861102, 216.6706125259247244 ) ) ;
#65733=DIRECTION ( 'NONE',  ( 0.5117323852940359741, 0.8591449038673723004, 0.000000000000000000 ) ) ;
#65747=LINE ( 'NONE', #41638, #9002 ) ;
#65751=VERTEX_POINT ( 'NONE', #102603 ) ;
#65758=( BOUNDED_SURFACE ( )  B_SPLINE_SURFACE ( 3, 2, ( 
 ( #28550, #70582, #37499 ),
 ( #46476, #71705, #27436 ),
 ( #70038, #12282, #19584 ),
 ( #78403, #2279, #61619 ),
 ( #20136, #87925, #36393 ),
 ( #63826, #3923, #44261 ),
 ( #11212, #79515, #95751 ),
 ( #45375, #19015, #87357 ),
 ( #80608, #88459, #80051 ),
 ( #96867, #104699, #10653 ),
 ( #54330, #36938, #71135 ),
 ( #38053, #54871, #105256 ),
 ( #27994, #62749, #3372 ),
 ( #105823, #72230, #29101 ) ),
 .UNSPECIFIED., .F., .F., .F. ) 
 B_SPLINE_SURFACE_WITH_KNOTS ( ( 4, 2, 2, 2, 2, 2, 4 ),
 ( 3, 3 ),
 ( 0.000000000000000000, 0.0009440840677143907175, 0.001416126101571585968, 0.001888168135428781435, 0.002360210169285976468, 0.002832252203143171936, 0.003776336270857562870 ),
 ( 0.000000000000000000, 1.000000000000000000 ),
 .UNSPECIFIED. ) 
 GEOMETRIC_REPRESENTATION_ITEM ( )  RATIONAL_B_SPLINE_SURFACE ( (
 ( 1.000000000000000000, 0.8070209408750022018, 1.000000000000000000),
 ( 1.000000000000000000, 0.8215603905293340503, 1.000000000000000000),
 ( 1.000000000000000000, 0.8340988699048569321, 1.000000000000000000),
 ( 1.000000000000000000, 0.8516751610464702305, 1.000000000000000000),
 ( 1.000000000000000000, 0.8573697395148289768, 1.000000000000000000),
 ( 1.000000000000000000, 0.8683586635668048004, 1.000000000000000000),
 ( 1.000000000000000000, 0.8736518481710696671, 1.000000000000000000),
 ( 1.000000000000000000, 0.8840377753027998109, 1.000000000000000000),
 ( 1.000000000000000000, 0.8891294171305048621, 1.000000000000000000),
 ( 1.000000000000000000, 0.8992456600575216008, 1.000000000000000000),
 ( 1.000000000000000000, 0.9042785869253413544, 1.000000000000000000),
 ( 1.000000000000000000, 0.9189749222837514386, 1.000000000000000000),
 ( 1.000000000000000000, 0.9283978182349121866, 1.000000000000000000),
 ( 1.000000000000000000, 0.9376006582765940012, 1.000000000000000000) ) ) 
 REPRESENTATION_ITEM ( '' )  SURFACE ( )  );
#65772=ORIENTED_EDGE ( 'NONE', *, *, #43284, .T. ) ;
#65780=EDGE_LOOP ( 'NONE', ( #27339, #70613, #34025, #46383 ) ) ;
#65792=ORIENTED_EDGE ( 'NONE', *, *, #75449, .F. ) ;
#65795=AXIS2_PLACEMENT_3D ( 'NONE', #82198, #72190, #63246 ) ;
#65802=CARTESIAN_POINT ( 'NONE',  ( 29.61692403810791419, 1526.104292489129193, 197.4873780791076001 ) ) ;
#65804=VECTOR ( 'NONE', #70776, 1000.000000000000000 ) ;
#65808=EDGE_CURVE ( 'NONE', #22289, #71455, #106555, .T. ) ;
#65817=EDGE_CURVE ( 'NONE', #14716, #46630, #15094, .T. ) ;
#65823=EDGE_CURVE ( 'NONE', #108510, #91781, #105963, .T. ) ;
#65827=FACE_OUTER_BOUND ( 'NONE', #38255, .T. ) ;
#65833=DIRECTION ( 'NONE',  ( -0.000000000000000000, -1.000000000000000000, -0.000000000000000000 ) ) ;
#65836=ADVANCED_FACE ( 'NONE', ( #80750 ), #29784, .T. ) ;
#65844=CARTESIAN_POINT ( 'NONE',  ( 20.70484064406364766, 1525.907212628473872, 185.0411015109854134 ) ) ;
#65850=EDGE_CURVE ( 'NONE', #31132, #55319, #56209, .T. ) ;
#65851=CARTESIAN_POINT ( 'NONE',  ( 31.12456774391174719, 1525.960063244516959, 201.1524202391562710 ) ) ;
#65857=EDGE_CURVE ( 'NONE', #34471, #23280, #51826, .T. ) ;
#65858=CARTESIAN_POINT ( 'NONE',  ( 0.000000000000000000, 1518.913060387330006, 209.1218459616979999 ) ) ;
#65867=ORIENTED_EDGE ( 'NONE', *, *, #99821, .T. ) ;
#65886=CARTESIAN_POINT ( 'NONE',  ( 32.92528853941135480, 1523.611961620354123, 201.0067946816160713 ) ) ;
#65892=TOROIDAL_SURFACE ( 'NONE', #83772, 32.13701971169416538, 1.000000000000000000 ) ;
#65913=CIRCLE ( 'NONE', #47993, 32.13701971169416538 ) ;
#65918=ORIENTED_EDGE ( 'NONE', *, *, #43865, .F. ) ;
#65923=CARTESIAN_POINT ( 'NONE',  ( -32.02808312589908013, 1511.187213306747708, 219.9649204700466782 ) ) ;
#65935=LINE ( 'NONE', #90003, #15294 ) ;
#65949=VERTEX_POINT ( 'NONE', #71988 ) ;
#65950=CARTESIAN_POINT ( 'NONE',  ( -29.61076903484010003, 1526.107876515966609, 197.4926634013643252 ) ) ;
#65951=EDGE_CURVE ( 'NONE', #51216, #94817, #97357, .T. ) ;
#65964=PLANE ( 'NONE',  #53167 ) ;
#65969=CIRCLE ( 'NONE', #14049, 1.999999999999993117 ) ;
#65981=CARTESIAN_POINT ( 'NONE',  ( -22.08523867432538879, 1523.530870145311610, 184.4211813602715893 ) ) ;
#65983=B_SPLINE_CURVE_WITH_KNOTS ( 'NONE', 3,
 ( #40517, #74695, #108827, #55699, #94787, #102067 ),
 .UNSPECIFIED., .F., .F.,
 ( 4, 2, 4 ),
 ( -1.131363979617638733E-05, 0.001067788114096024149, 0.002146889867988224614 ),
 .UNSPECIFIED. ) ;
#65994=CARTESIAN_POINT ( 'NONE',  ( -18.19590854888121356, 1522.382868172863937, 238.2026672068777202 ) ) ;
#65997=CARTESIAN_POINT ( 'NONE',  ( -16.81611548244467258, 1526.382868172864164, 234.5451076435288371 ) ) ;
#66013=CARTESIAN_POINT ( 'NONE',  ( 18.19590854888146580, 1522.382868172863937, 180.0410247165184217 ) ) ;
#66016=FACE_OUTER_BOUND ( 'NONE', #97842, .T. ) ;
#66021=LINE ( 'NONE', #67119, #90822 ) ;
#66023=AXIS2_PLACEMENT_3D ( 'NONE', #110318, #58823, #67241 ) ;
#66025=ORIENTED_EDGE ( 'NONE', *, *, #39427, .F. ) ;
#66031=CARTESIAN_POINT ( 'NONE',  ( -31.81407709660758698, 1522.382868172863937, 221.9534378623334305 ) ) ;
#66047=AXIS2_PLACEMENT_3D ( 'NONE', #73731, #15432, #6500 ) ;
#66052=CARTESIAN_POINT ( 'NONE',  ( -19.53786426058999481, 1511.187213306747708, 236.7197124308268030 ) ) ;
#66055=EDGE_CURVE ( 'NONE', #33528, #55613, #90155, .T. ) ;
#66077=VERTEX_POINT ( 'NONE', #25377 ) ;
#66095=CARTESIAN_POINT ( 'NONE',  ( 22.08622291482331335, 1523.382868172864164, 184.4183880513174927 ) ) ;
#66104=CARTESIAN_POINT ( 'NONE',  ( 31.29224604902393381, 1525.661275128775515, 201.9587785200654650 ) ) ;
#66112=CARTESIAN_POINT ( 'NONE',  ( 16.57542919120497515, 1524.538768545233779, 237.5505425563592041 ) ) ;
#66119=CARTESIAN_POINT ( 'NONE',  ( -29.00779973304138437, 1526.382868172864164, 200.9494832830839073 ) ) ;
#66127=VECTOR ( 'NONE', #158, 1000.000000000000000 ) ;
#66129=CARTESIAN_POINT ( 'NONE',  ( -32.38845791999490586, 1512.187213306747481, 216.1254071228449902 ) ) ;
#66130=CARTESIAN_POINT ( 'NONE',  ( -1.393816646507350487, 1512.187213306747481, 243.1385343369520342 ) ) ;
#66144=ORIENTED_EDGE ( 'NONE', *, *, #59143, .F. ) ;
#66145=CARTESIAN_POINT ( 'NONE',  ( -17.19754479272735637, 1524.059663615499630, 180.8698486848230971 ) ) ;
#66159=EDGE_LOOP ( 'NONE', ( #97913, #73340, #18434, #54983, #99709 ) ) ;
#66171=CARTESIAN_POINT ( 'NONE',  ( -0.4151546846821903003, 1511.187213306747708, 243.9330574173806951 ) ) ;
#66188=DIRECTION ( 'NONE',  ( 0.4090087482554252696, 0.000000000000000000, -0.9125304618753996566 ) ) ;
#66194=AXIS2_PLACEMENT_3D ( 'NONE', #42224, #92069, #16977 ) ;
#66201=LINE ( 'NONE', #109286, #84717 ) ;
#66212=AXIS2_PLACEMENT_3D ( 'NONE', #43440, #11495, #28285 ) ;
#66223=ORIENTED_EDGE ( 'NONE', *, *, #90507, .F. ) ;
#66228=ADVANCED_FACE ( 'NONE', ( #18299 ), #3209, .F. ) ;
#66230=CARTESIAN_POINT ( 'NONE',  ( 0.000000000000000000, 1511.187213306747708, 209.1218459616979999 ) ) ;
#66232=DIRECTION ( 'NONE',  ( 0.8090169943749465631, -0.000000000000000000, -0.5877852522924742473 ) ) ;
#66266=EDGE_LOOP ( 'NONE', ( #88076, #60220, #81080, #99756 ) ) ;
#66294=CARTESIAN_POINT ( 'NONE',  ( 30.95751052620450494, 1525.821544997590081, 216.7905424461071675 ) ) ;
#66306=CARTESIAN_POINT ( 'NONE',  ( 16.88555899345125866, 1525.556089352344316, 236.5668029769053931 ) ) ;
#66308=CARTESIAN_POINT ( 'NONE',  ( 19.37374569213924502, 1524.382868172863937, 183.8768763279539655 ) ) ;
#66309=CIRCLE ( 'NONE', #105618, 2.000000000000001776 ) ;
#66323=VERTEX_POINT ( 'NONE', #86197 ) ;
#66333=SURFACE_SIDE_STYLE ('',( #30486 ) ) ;
#66347=EDGE_LOOP ( 'NONE', ( #71317, #44248, #21369, #91941 ) ) ;
#66379=CARTESIAN_POINT ( 'NONE',  ( 30.61115703708031432, 1523.542365884047740, 196.4197133992099396 ) ) ;
#66389=CARTESIAN_POINT ( 'NONE',  ( 30.31404213106236512, 1524.330813522192102, 221.7920027509178169 ) ) ;
#66405=CARTESIAN_POINT ( 'NONE',  ( 20.07149347155336372, 1526.186458717542791, 185.1794229323649290 ) ) ;
#66406=AXIS2_PLACEMENT_3D ( 'NONE', #96265, #104107, #2236 ) ;
#66416=CARTESIAN_POINT ( 'NONE',  ( -16.66700976312950644, 1523.530935881284904, 180.4846138748687281 ) ) ;
#66442=( GEOMETRIC_REPRESENTATION_CONTEXT ( 3 ) GLOBAL_UNCERTAINTY_ASSIGNED_CONTEXT ( ( #24471 ) ) GLOBAL_UNIT_ASSIGNED_CONTEXT ( ( #64675, #14786, #89842 ) ) REPRESENTATION_CONTEXT ( 'NONE', 'WORKASPACE' ) );
#66471=AXIS2_PLACEMENT_3D ( 'NONE', #95184, #1142, #41480 ) ;
#66473=CARTESIAN_POINT ( 'NONE',  ( 22.03465957474552539, 1522.382868172863937, 182.8300405912328301 ) ) ;
#66482=AXIS2_PLACEMENT_3D ( 'NONE', #15543, #49743, #75501 ) ;
#66492=DIRECTION ( 'NONE',  ( 0.000000000000000000, 0.000000000000000000, 1.000000000000000000 ) ) ;
#66494=CARTESIAN_POINT ( 'NONE',  ( -28.49879435372385572, 1526.382868173645647, 219.8425395114961702 ) ) ;
#66514=CARTESIAN_POINT ( 'NONE',  ( 17.19739463999625784, 1525.960063244516959, 181.9833109756548595 ) ) ;
#66528=DIRECTION ( 'NONE',  ( -0.8672669759446596238, 0.000000000000000000, 0.4978433412588795792 ) ) ;
#66530=CARTESIAN_POINT ( 'NONE',  ( -33.36586802512168504, 1523.382868172864164, 216.3367586934473366 ) ) ;
#66534=CARTESIAN_POINT ( 'NONE',  ( 1.393816646507350709, 1511.187213306747708, 175.1051575864439656 ) ) ;
#66546=EDGE_CURVE ( 'NONE', #43885, #53799, #100114, .T. ) ;
#66550=CARTESIAN_POINT ( 'NONE',  ( 16.68062049856701989, 1524.382868172863937, 181.4122394607862816 ) ) ;
#66558=CARTESIAN_POINT ( 'NONE',  ( 33.52308185467592239, 1525.402221411349501, 217.5800527287148043 ) ) ;
#66583=CARTESIAN_POINT ( 'NONE',  ( -21.83117874278453741, 1524.760046179776054, 184.6256242011980930 ) ) ;
#66621=EDGE_LOOP ( 'NONE', ( #31439, #94692, #93739, #71027, #28415 ) ) ;
#66627=ORIENTED_EDGE ( 'NONE', *, *, #11981, .F. ) ;
#66652=CARTESIAN_POINT ( 'NONE',  ( -30.25425994617014780, 1526.382868172863937, 199.2916410102373277 ) ) ;
#66669=CYLINDRICAL_SURFACE ( 'NONE', #19908, 2.000000000000009770 ) ;
#66673=CARTESIAN_POINT ( 'NONE',  ( -3.246772394788719929, 1512.187213306747481, 241.0944358625217774 ) ) ;
#66675=CARTESIAN_POINT ( 'NONE',  ( -0.6235920161070115375, 1525.878013734321257, 175.2961586039431552 ) ) ;
#66681=CARTESIAN_POINT ( 'NONE',  ( 2.385013337802738498, 1526.073434386619056, 177.7125070007693353 ) ) ;
#66682=EDGE_CURVE ( 'NONE', #109192, #91565, #91862, .T. ) ;
#66699=CARTESIAN_POINT ( 'NONE',  ( -18.88880210472915877, 1524.667648926078755, 238.8296805722607417 ) ) ;
#66704=ORIENTED_EDGE ( 'NONE', *, *, #28127, .F. ) ;
#66712=EDGE_CURVE ( 'NONE', #16710, #92713, #25885, .T. ) ;
#66730=ORIENTED_EDGE ( 'NONE', *, *, #31936, .F. ) ;
#66741=CARTESIAN_POINT ( 'NONE',  ( -31.23437356469425907, 1518.913060387330006, 221.8968241038848248 ) ) ;
#66746=DIRECTION ( 'NONE',  ( -0.000000000000000000, -1.000000000000000000, -0.000000000000000000 ) ) ;
#66763=CARTESIAN_POINT ( 'NONE',  ( 30.24841015875314909, 1524.082740465118832, 222.4736143106622706 ) ) ;
#66791=CARTESIAN_POINT ( 'NONE',  ( -22.04658049762760896, 1524.075132568162417, 233.7649773472511470 ) ) ;
#66794=CARTESIAN_POINT ( 'NONE',  ( -31.81407709660785699, 1501.977400791986611, 196.2902540610632229 ) ) ;
#66796=ORIENTED_EDGE ( 'NONE', *, *, #79151, .T. ) ;
#66812=B_SPLINE_CURVE_WITH_KNOTS ( 'NONE', 3,
 ( #30793, #12335, #4510, #72277, #82852, #90138 ),
 .UNSPECIFIED., .F., .F.,
 ( 4, 2, 4 ),
 ( -1.285435071098408229E-05, 0.001079388306740762700, 0.002171630964192509169 ),
 .UNSPECIFIED. ) ;
#66816=CARTESIAN_POINT ( 'NONE',  ( 2.470168521978398868, 1512.187213306747481, 242.8787258963054683 ) ) ;
#66826=CARTESIAN_POINT ( 'NONE',  ( 20.69714064973412349, 1525.848198008145346, 233.9618268462910180 ) ) ;
#66828=DIRECTION ( 'NONE',  ( 5.204170427930416866E-14, 0.000000000000000000, 1.000000000000000000 ) ) ;
#66830=CARTESIAN_POINT ( 'NONE',  ( 1.909775791882409202, 1526.107880201381477, 240.8769681478140399 ) ) ;
#66842=ORIENTED_EDGE ( 'NONE', *, *, #26404, .F. ) ;
#66849=CARTESIAN_POINT ( 'NONE',  ( 16.94364159994348284, 1525.231887713385731, 236.8652194622064826 ) ) ;
#66855=DIRECTION ( 'NONE',  ( -0.7414773880254650340, -0.000000000000000000, -0.6709778558543747495 ) ) ;
#66871=DIRECTION ( 'NONE',  ( -0.8090169943749422332, 0.000000000000000000, 0.5877852522924802425 ) ) ;
#66895=DIRECTION ( 'NONE',  ( 0.000000000000000000, 0.000000000000000000, -1.000000000000000000 ) ) ;
#66900=VERTEX_POINT ( 'NONE', #77552 ) ;
#66904=CARTESIAN_POINT ( 'NONE',  ( -32.37018134260392088, 1511.187213306747708, 218.0712926453366833 ) ) ;
#66919=CARTESIAN_POINT ( 'NONE',  ( 17.83486663330486621, 1523.678648413191695, 180.3677388339000061 ) ) ;
#66935=CARTESIAN_POINT ( 'NONE',  ( 30.80549360313091967, 1524.130440953581001, 221.8448932001212484 ) ) ;
#66942=CARTESIAN_POINT ( 'NONE',  ( 2.372478608332516892, 1501.977400791986611, 174.8996806668726549 ) ) ;
#66951=B_SPLINE_CURVE_WITH_KNOTS ( 'NONE', 3,
 ( #36462, #80678, #11818, #37571 ),
 .UNSPECIFIED., .F., .F.,
 ( 4, 4 ),
 ( 0.000000000000000000, 0.0002960034161021618732 ),
 .UNSPECIFIED. ) ;
#66952=CARTESIAN_POINT ( 'NONE',  ( 19.30300490008536229, 1526.348417187218274, 185.0858834514518492 ) ) ;
#66953=DIRECTION ( 'NONE',  ( 0.000000000000000000, 1.000000000000000000, 0.000000000000000000 ) ) ;
#66997=CARTESIAN_POINT ( 'NONE',  ( 2.131986625866193030, 1526.000688113870183, 240.6925538244833831 ) ) ;
#67002=B_SPLINE_CURVE_WITH_KNOTS ( 'NONE', 3,
 ( #80686, #4534, #31368, #48752, #66112, #3997, #82332, #65551, #31920, #14007, #89624, #100236 ),
 .UNSPECIFIED., .F., .F.,
 ( 4, 2, 2, 2, 2, 4 ),
 ( 0.000000000000000000, 0.0007194225121803780225, 0.001079133768270252669, 0.001438845024360127425, 0.002158267536539321824, 0.002877690048718516656 ),
 .UNSPECIFIED. ) ;
#67010=VECTOR ( 'NONE', #44195, 1000.000000000000000 ) ;
#67015=VECTOR ( 'NONE', #10852, 1000.000000000000000 ) ;
#67019=AXIS2_PLACEMENT_3D ( 'NONE', #87478, #2394, #14040 ) ;
#67026=DIRECTION ( 'NONE',  ( 2.428612866367527723E-14, 0.000000000000000000, 1.000000000000000000 ) ) ;
#67029=CARTESIAN_POINT ( 'NONE',  ( -17.83486663330527122, 1523.678648413191695, 180.3677388339002050 ) ) ;
#67030=CARTESIAN_POINT ( 'NONE',  ( 21.44521871417756032, 1525.343710797494850, 184.8098458366069394 ) ) ;
#67034=CARTESIAN_POINT ( 'NONE',  ( -29.86461515634909603, 1525.960063244516959, 220.9690070206026178 ) ) ;
#67057=DIRECTION ( 'NONE',  ( -0.000000000000000000, -1.000000000000000000, -0.000000000000000000 ) ) ;
#67063=ORIENTED_EDGE ( 'NONE', *, *, #76848, .F. ) ;
#67067=EDGE_CURVE ( 'NONE', #72816, #71731, #93587, .T. ) ;
#67068=( BOUNDED_CURVE ( )  B_SPLINE_CURVE ( 3, ( #70430, #105104, #19982, #54176 ),
 .UNSPECIFIED., .F., .F. ) 
 B_SPLINE_CURVE_WITH_KNOTS ( ( 4, 4 ),
 ( 0.000000000000000000, 0.7048113239778082129 ),
 .UNSPECIFIED. ) 
 CURVE ( )  GEOMETRIC_REPRESENTATION_ITEM ( )  RATIONAL_B_SPLINE_CURVE ( ( 1.000000000000000000, 0.9590300661663089254, 0.9590300661663089254, 1.000000000000000000 ) ) 
 REPRESENTATION_ITEM ( '' )  );
#67070=CARTESIAN_POINT ( 'NONE',  ( 2.865545859819519148, 1525.651285554128663, 177.1364457139975173 ) ) ;
#67086=DIRECTION ( 'NONE',  ( 0.000000000000000000, 0.000000000000000000, 1.000000000000000000 ) ) ;
#67088=CARTESIAN_POINT ( 'NONE',  ( 2.902322711624676882E-15, 1523.409940573003951, 232.8211094035767985 ) ) ;
#67094=CARTESIAN_POINT ( 'NONE',  ( 19.37774363895821850, 1525.878013734320120, 181.3897518523426982 ) ) ;
#67097=LINE ( 'NONE', #92270, #1737 ) ;
#67119=CARTESIAN_POINT ( 'NONE',  ( 49.24962907673570811, 1526.382868172863937, 10.34030387146701635 ) ) ;
#67123=AXIS2_PLACEMENT_3D ( 'NONE', #59777, #61446, #26699 ) ;
#67158=EDGE_LOOP ( 'NONE', ( #15743, #20586, #108010, #59723 ) ) ;
#67163=VERTEX_POINT ( 'NONE', #39396 ) ;
#67169=CIRCLE ( 'NONE', #18852, 1.000000000000000888 ) ;
#67176=DIRECTION ( 'NONE',  ( -0.000000000000000000, -1.000000000000000000, -0.000000000000000000 ) ) ;
#67192=ORIENTED_EDGE ( 'NONE', *, *, #33566, .T. ) ;
#67195=CARTESIAN_POINT ( 'NONE',  ( 31.10384971727509651, 1525.795403621570813, 201.8948720197292630 ) ) ;
#67197=EDGE_CURVE ( 'NONE', #95247, #10483, #31562, .T. ) ;
#67201=EDGE_CURVE ( 'NONE', #101260, #97990, #79830, .T. ) ;
#67210=TOROIDAL_SURFACE ( 'NONE', #11725, 2.000000000000000000, 1.000000000000000000 ) ;
#67211=( BOUNDED_SURFACE ( )  B_SPLINE_SURFACE ( 3, 2, ( 
 ( #75430, #22763, #92204 ),
 ( #14378, #81584, #82706 ),
 ( #107898, #13821, #82145 ),
 ( #108458, #5444, #67029 ) ),
 .UNSPECIFIED., .F., .F., .F. ) 
 B_SPLINE_SURFACE_WITH_KNOTS ( ( 4, 4 ),
 ( 3, 3 ),
 ( 0.000000000000000000, 0.0002960034161023850021 ),
 ( 0.000000000000000000, 1.000000000000000000 ),
 .UNSPECIFIED. ) 
 GEOMETRIC_REPRESENTATION_ITEM ( )  RATIONAL_B_SPLINE_SURFACE ( (
 ( 1.000000000000000000, 0.8072480644198086752, 1.000000000000000000),
 ( 1.000000000000000000, 0.8072480346917640937, 1.000000000000000000),
 ( 1.000000000000000000, 0.8071723757218238759, 1.000000000000000000),
 ( 1.000000000000000000, 0.8070209408750101954, 1.000000000000000000) ) ) 
 REPRESENTATION_ITEM ( '' )  SURFACE ( )  );
#67217=CARTESIAN_POINT ( 'NONE',  ( 32.85805783624308418, 1523.678648413191695, 217.1983043299902931 ) ) ;
#67220=DIRECTION ( 'NONE',  ( 0.000000000000000000, 0.000000000000000000, 1.000000000000000000 ) ) ;
#67221=DIRECTION ( 'NONE',  ( -0.4090087482554316534, 0.000000000000000000, -0.9125304618753967700 ) ) ;
#67223=CARTESIAN_POINT ( 'NONE',  ( -0.7800921441517267851, 1526.382868172863937, 176.7869413415625388 ) ) ;
#67236=ORIENTED_EDGE ( 'NONE', *, *, #75435, .F. ) ;
#67241=DIRECTION ( 'NONE',  ( 0.2054769195713296304, 0.000000000000000000, -0.9786619618251631847 ) ) ;
#67242=EDGE_CURVE ( 'NONE', #50666, #38471, #718, .T. ) ;
#67249=CARTESIAN_POINT ( 'NONE',  ( -19.39983987834741797, 1522.861859112240154, 239.2921289694189682 ) ) ;
#67259=VECTOR ( 'NONE', #105553, 1000.000000000000000 ) ;
#67275=CARTESIAN_POINT ( 'NONE',  ( 0.000000000000000000, 1523.051704408389696, 209.1218459616979999 ) ) ;
#67279=EDGE_CURVE ( 'NONE', #46630, #38078, #34848, .T. ) ;
#67288=EDGE_CURVE ( 'NONE', #20620, #74525, #28104, .T. ) ;
#67317=ADVANCED_FACE ( 'NONE', ( #36511 ), #68859, .T. ) ;
#67327=LINE ( 'NONE', #91949, #10181 ) ;
#67340=EDGE_CURVE ( 'NONE', #15596, #22899, #54310, .T. ) ;
#67344=VERTEX_POINT ( 'NONE', #9637 ) ;
#67354=EDGE_CURVE ( 'NONE', #30026, #89438, #54973, .T. ) ;
#67358=VERTEX_POINT ( 'NONE', #18577 ) ;
#67361=CARTESIAN_POINT ( 'NONE',  ( -32.23107245337067184, 1523.542365884047285, 216.8383915158452453 ) ) ;
#67377=ADVANCED_FACE ( 'NONE', ( #44377 ), #27556, .T. ) ;
#67384=LINE ( 'NONE', #43272, #11055 ) ;
#67398=CARTESIAN_POINT ( 'NONE',  ( 17.19757137884747777, 1524.059547553518996, 180.8698536207154461 ) ) ;
#67403=CARTESIAN_POINT ( 'NONE',  ( 17.29393938232482952, 1523.621879633028811, 237.3864571009499969 ) ) ;
#67416=ORIENTED_EDGE ( 'NONE', *, *, #78822, .T. ) ;
#67417=ORIENTED_EDGE ( 'NONE', *, *, #16854, .T. ) ;
#67420=ORIENTED_EDGE ( 'NONE', *, *, #66055, .T. ) ;
#67424=CARTESIAN_POINT ( 'NONE',  ( -16.73628186595804479, 1526.382868172863937, 234.1845039693045862 ) ) ;
#67443=AXIS2_PLACEMENT_3D ( 'NONE', #92622, #7526, #41684 ) ;
#67447=CARTESIAN_POINT ( 'NONE',  ( 0.000000000000000000, 1526.382868172863937, 209.1218459616979999 ) ) ;
#67453=CYLINDRICAL_SURFACE ( 'NONE', #107030, 0.9999999999999888978 ) ;
#67466=FACE_OUTER_BOUND ( 'NONE', #5684, .T. ) ;
#67483=AXIS2_PLACEMENT_3D ( 'NONE', #33713, #16346, #41020 ) ;
#67492=ADVANCED_FACE ( 'NONE', ( #41880 ), #30852, .T. ) ;
#67500=FACE_OUTER_BOUND ( 'NONE', #89937, .T. ) ;
#67503=CARTESIAN_POINT ( 'NONE',  ( -21.11881948555236121, 1525.651286436460396, 184.9294397280434623 ) ) ;
#67514=EDGE_CURVE ( 'NONE', #10483, #69831, #102776, .T. ) ;
#67517=DIRECTION ( 'NONE',  ( 0.000000000000000000, 0.000000000000000000, 1.000000000000000000 ) ) ;
#67524=DIRECTION ( 'NONE',  ( 0.000000000000000000, 0.000000000000000000, 1.000000000000000000 ) ) ;
#67546=CARTESIAN_POINT ( 'NONE',  ( -32.38114538885259464, 1523.604703353109699, 202.1233279672532888 ) ) ;
#67562=TOROIDAL_SURFACE ( 'NONE', #60443, 1.000000000000000000, 1.000000000000000000 ) ;
#67570=VERTEX_POINT ( 'NONE', #36242 ) ;
#67571=CYLINDRICAL_SURFACE ( 'NONE', #70761, 1.999999999999996225 ) ;
#67579=CARTESIAN_POINT ( 'NONE',  ( 22.08327125186925954, 1523.604703353109699, 184.4267662568470598 ) ) ;
#67580=ORIENTED_EDGE ( 'NONE', *, *, #101696, .T. ) ;
#67593=ORIENTED_EDGE ( 'NONE', *, *, #52472, .T. ) ;
#67598=CARTESIAN_POINT ( 'NONE',  ( -3.258294392304168507, 1524.756004293092474, 241.7666560717732978 ) ) ;
#67604=DIRECTION ( 'NONE',  ( -0.000000000000000000, -1.000000000000000000, -0.000000000000000000 ) ) ;
#67611=EDGE_LOOP ( 'NONE', ( #9543, #27353, #6216, #72255, #19484 ) ) ;
#67617=DIRECTION ( 'NONE',  ( 0.000000000000000000, 0.000000000000000000, 1.000000000000000000 ) ) ;
#67618=CARTESIAN_POINT ( 'NONE',  ( -29.40443212115401650, 1511.187213306747708, 196.1539082851718661 ) ) ;
#67624=EDGE_CURVE ( 'NONE', #17762, #11785, #457, .T. ) ;
#67634=AXIS2_PLACEMENT_3D ( 'NONE', #57026, #61716, #95838 ) ;
#67643=DIRECTION ( 'NONE',  ( 0.6709778558543728622, 0.000000000000000000, 0.7414773880254666993 ) ) ;
#67652=CARTESIAN_POINT ( 'NONE',  ( 32.92528853941223588, 1523.611961620354123, 217.2368972417801558 ) ) ;
#67660=LINE ( 'NONE', #100672, #17396 ) ;
#67664=FACE_OUTER_BOUND ( 'NONE', #82301, .T. ) ;
#67667=VECTOR ( 'NONE', #490, 1000.000000000000000 ) ;
#67674=ORIENTED_EDGE ( 'NONE', *, *, #50282, .T. ) ;
#67679=DIRECTION ( 'NONE',  ( 0.000000000000000000, 0.000000000000000000, 1.000000000000000000 ) ) ;
#67694=DIRECTION ( 'NONE',  ( 0.000000000000000000, 1.000000000000000000, 0.000000000000000000 ) ) ;
#67710=ORIENTED_EDGE ( 'NONE', *, *, #66055, .F. ) ;
#67711=ORIENTED_EDGE ( 'NONE', *, *, #97988, .T. ) ;
#67713=ORIENTED_EDGE ( 'NONE', *, *, #11712, .F. ) ;
#67717=TOROIDAL_SURFACE ( 'NONE', #30121, 32.13701971169416538, 1.000000000000000000 ) ;
#67724=( BOUNDED_SURFACE ( )  B_SPLINE_SURFACE ( 3, 2, ( 
 ( #62774, #96889, #20159 ),
 ( #13954, #107472, #15593 ),
 ( #64949, #91230, #15051 ),
 ( #22895, #14510, #16156 ) ),
 .UNSPECIFIED., .F., .F., .F. ) 
 B_SPLINE_SURFACE_WITH_KNOTS ( ( 4, 4 ),
 ( 3, 3 ),
 ( 0.000000000000000000, 0.0002960034161023842431 ),
 ( 0.000000000000000000, 1.000000000000000000 ),
 .UNSPECIFIED. ) 
 GEOMETRIC_REPRESENTATION_ITEM ( )  RATIONAL_B_SPLINE_SURFACE ( (
 ( 1.000000000000000000, 0.8072480644198088973, 1.000000000000000000),
 ( 1.000000000000000000, 0.8072480346917659810, 1.000000000000000000),
 ( 1.000000000000000000, 0.8071723757218326467, 1.000000000000000000),
 ( 1.000000000000000000, 0.8070209408750008695, 1.000000000000000000) ) ) 
 REPRESENTATION_ITEM ( '' )  SURFACE ( )  );
#67726=ORIENTED_EDGE ( 'NONE', *, *, #100830, .F. ) ;
#67729=CARTESIAN_POINT ( 'NONE',  ( 31.23437356469446868, 1512.187213306747481, 222.8968241038843701 ) ) ;
#67740=DIRECTION ( 'NONE',  ( -0.000000000000000000, -1.000000000000000000, -0.000000000000000000 ) ) ;
#67743=CARTESIAN_POINT ( 'NONE',  ( 3.143095077906818524, 1525.137881624898682, 241.5427404054744329 ) ) ;
#67757=CARTESIAN_POINT ( 'NONE',  ( -29.71163624023799343, 1526.333389947990554, 201.1407003069400048 ) ) ;
#67773=CARTESIAN_POINT ( 'NONE',  ( -31.81407709660760830, 1522.382868172863937, 221.9534378623334590 ) ) ;
#67775=CARTESIAN_POINT ( 'NONE',  ( 1.800936940629440430, 1526.306647125542668, 178.3505287518698026 ) ) ;
#67784=CARTESIAN_POINT ( 'NONE',  ( 2.621078202466677443, 1523.542365884047285, 176.0837307636417393 ) ) ;
#67790=AXIS2_PLACEMENT_3D ( 'NONE', #4809, #80979, #98320 ) ;
#67801=CARTESIAN_POINT ( 'NONE',  ( -1.191524307911315583, 1526.382868172863937, 239.2353018730792087 ) ) ;
#67818=DIRECTION ( 'NONE',  ( 0.5877852522924673639, 0.000000000000000000, -0.8090169943749514481 ) ) ;
#67820=CARTESIAN_POINT ( 'NONE',  ( -32.15938645527118922, 1524.538768545234007, 216.1010655287031739 ) ) ;
#67825=ORIENTED_EDGE ( 'NONE', *, *, #105132, .T. ) ;
#67835=CARTESIAN_POINT ( 'NONE',  ( 21.48648064083751663, 1524.477587234266366, 234.0869179060386216 ) ) ;
#67838=EDGE_CURVE ( 'NONE', #32890, #58486, #67068, .T. ) ;
#67856=CARTESIAN_POINT ( 'NONE',  ( -31.12456774391181469, 1525.960063244516959, 201.1524202391567258 ) ) ;
#67859=ADVANCED_FACE ( 'NONE', ( #98345 ), #72610, .T. ) ;
#67878=EDGE_CURVE ( 'NONE', #91956, #73515, #98946, .T. ) ;
#67887=VECTOR ( 'NONE', #65583, 1000.000000000000000 ) ;
#67890=CARTESIAN_POINT ( 'NONE',  ( -21.39303731107321127, 1524.776010967693082, 233.9875059046097192 ) ) ;
#67901=CARTESIAN_POINT ( 'NONE',  ( 0.000000000000000000, 1523.382868172864164, 209.1218459616979999 ) ) ;
#67927=ADVANCED_FACE ( 'NONE', ( #52928 ), #26026, .T. ) ;
#67931=CARTESIAN_POINT ( 'NONE',  ( -30.51921334599336788, 1524.059663615499858, 196.3739632444808763 ) ) ;
#67940=CARTESIAN_POINT ( 'NONE',  ( -19.00259723423208769, 1526.382868173645647, 185.3307583834140928 ) ) ;
#67957=CIRCLE ( 'NONE', #3547, 1.000000000000000888 ) ;
#67963=CARTESIAN_POINT ( 'NONE',  ( -30.45769963431186866, 1526.208281990536761, 201.0929247824073229 ) ) ;
#67967=CIRCLE ( 'NONE', #39327, 1.000000000000000888 ) ;
#67992=ORIENTED_EDGE ( 'NONE', *, *, #50445, .F. ) ;
#68004=ORIENTED_EDGE ( 'NONE', *, *, #53740, .T. ) ;
#68013=VERTEX_POINT ( 'NONE', #28819 ) ;
#68019=CARTESIAN_POINT ( 'NONE',  ( 20.60985939166121739, 1525.581535527369397, 181.7364793965037677 ) ) ;
#68026=CARTESIAN_POINT ( 'NONE',  ( -21.59395510246054073, 1525.159177407155539, 233.4989687676688845 ) ) ;
#68032=AXIS2_PLACEMENT_3D ( 'NONE', #11200, #69463, #45364 ) ;
#68058=CARTESIAN_POINT ( 'NONE',  ( -21.46350454714179534, 1524.972383263452912, 183.7395372259029784 ) ) ;
#68069=CARTESIAN_POINT ( 'NONE',  ( 33.34040796508542570, 1523.342713519623203, 196.1259889609349329 ) ) ;
#68080=TOROIDAL_SURFACE ( 'NONE', #94911, 1.000000000000000000, 1.000000000000000000 ) ;
#68087=DIRECTION ( 'NONE',  ( 0.000000000000000000, 1.000000000000000000, 0.000000000000000000 ) ) ;
#68094=CARTESIAN_POINT ( 'NONE',  ( -0.4992773797353681764, 1524.841055067849766, 244.1317247718872920 ) ) ;
#68101=ORIENTED_EDGE ( 'NONE', *, *, #75722, .F. ) ;
#68106=DIRECTION ( 'NONE',  ( 0.9774101051267699569, 0.000000000000000000, -0.2113515706023416929 ) ) ;
#68117=EDGE_CURVE ( 'NONE', #45131, #59426, #32116, .T. ) ;
#68134=LINE ( 'NONE', #103333, #92202 ) ;
#68138=B_SPLINE_CURVE_WITH_KNOTS ( 'NONE', 3,
 ( #53579, #35639, #2073, #70947, #61986, #37311 ),
 .UNSPECIFIED., .F., .F.,
 ( 4, 2, 4 ),
 ( 1.040834085586084103E-17, 0.001087661325621710768, 0.002175322651243411128 ),
 .UNSPECIFIED. ) ;
#68148=DIRECTION ( 'NONE',  ( 0.2054769195713296304, -0.000000000000000000, 0.9786619618251631847 ) ) ;
#68151=EDGE_CURVE ( 'NONE', #58486, #108102, #20851, .T. ) ;
#68189=FACE_OUTER_BOUND ( 'NONE', #66266, .T. ) ;
#68205=CARTESIAN_POINT ( 'NONE',  ( 28.27139721233034919, 1526.382868172864164, 219.5606225550385204 ) ) ;
#68213=CARTESIAN_POINT ( 'NONE',  ( 30.99338347248546555, 1526.382868172863937, 218.3719692838077719 ) ) ;
#68217=EDGE_LOOP ( 'NONE', ( #13035, #89402, #40473, #8738 ) ) ;
#68222=DIRECTION ( 'NONE',  ( 0.000000000000000000, 0.000000000000000000, -1.000000000000000000 ) ) ;
#68225=CARTESIAN_POINT ( 'NONE',  ( -32.38845791999490586, 1523.382868172864164, 216.1254071228449902 ) ) ;
#68237=CARTESIAN_POINT ( 'NONE',  ( 17.06401309437801217, 1526.329757971584513, 237.1783921619710895 ) ) ;
#68249=CIRCLE ( 'NONE', #70010, 2.000000000000001776 ) ;
#68253=LINE ( 'NONE', #77187, #67667 ) ;
#68260=CIRCLE ( 'NONE', #89639, 2.000000000000001776 ) ;
#68262=ORIENTED_EDGE ( 'NONE', *, *, #75677, .F. ) ;
#68265=CARTESIAN_POINT ( 'NONE',  ( -2.664543536381771549, 1524.964158026965606, 176.5360755200448182 ) ) ;
#68272=DIRECTION ( 'NONE',  ( 0.2054769195713296581, 0.000000000000000000, -0.9786619618251632957 ) ) ;
#68273=ORIENTED_EDGE ( 'NONE', *, *, #42536, .T. ) ;
#68307=CARTESIAN_POINT ( 'NONE',  ( 2.385609657812846951, 1525.697946996627479, 241.0978147455549845 ) ) ;
#68315=DIRECTION ( 'NONE',  ( 0.000000000000000000, 0.000000000000000000, -1.000000000000000000 ) ) ;
#68316=AXIS2_PLACEMENT_3D ( 'NONE', #66673, #24610, #15119 ) ;
#68341=CARTESIAN_POINT ( 'NONE',  ( 31.92108011125350231, 1512.187213306747481, 220.9591791661896139 ) ) ;
#68362=CARTESIAN_POINT ( 'NONE',  ( -2.596261494520238688, 1525.907212628473644, 240.7735774411713123 ) ) ;
#68378=CARTESIAN_POINT ( 'NONE',  ( -32.05392771830335619, 1524.756004293092701, 216.1108249500459237 ) ) ;
#68382=CARTESIAN_POINT ( 'NONE',  ( -2.038847259689231084, 1501.977400791986611, 244.9330574173806951 ) ) ;
#68384=EDGE_CURVE ( 'NONE', #85993, #38713, #62447, .T. ) ;
#68404=ORIENTED_EDGE ( 'NONE', *, *, #92115, .T. ) ;
#68466=DIRECTION ( 'NONE',  ( 0.000000000000000000, 1.000000000000000000, 0.000000000000000000 ) ) ;
#68467=DIRECTION ( 'NONE',  ( -0.000000000000000000, -1.000000000000000000, -0.000000000000000000 ) ) ;
#68470=EDGE_CURVE ( 'NONE', #39930, #54321, #78566, .T. ) ;
#68473=DIRECTION ( 'NONE',  ( -0.7414773880254664773, -0.000000000000000000, 0.6709778558543730842 ) ) ;
#68494=DIRECTION ( 'NONE',  ( -0.8090169943749385695, 0.000000000000000000, 0.5877852522924854606 ) ) ;
#68498=CARTESIAN_POINT ( 'NONE',  ( 16.92737646175363508, 1525.317359687841190, 181.4495904955261665 ) ) ;
#68517=ORIENTED_EDGE ( 'NONE', *, *, #71381, .F. ) ;
#68519=CARTESIAN_POINT ( 'NONE',  ( 21.26059330700248040, 1525.055427061254932, 184.3612831740845479 ) ) ;
#68537=EDGE_LOOP ( 'NONE', ( #108725, #95194, #24012, #76860 ) ) ;
#68553=DIRECTION ( 'NONE',  ( 0.000000000000000000, 1.000000000000000000, 0.000000000000000000 ) ) ;
#68565=CARTESIAN_POINT ( 'NONE',  ( 21.19880661588985404, 1526.382868172863937, 184.6948938244646854 ) ) ;
#68574=EDGE_LOOP ( 'NONE', ( #93155, #16890, #74312 ) ) ;
#68602=CARTESIAN_POINT ( 'NONE',  ( -21.60845823726274872, 1524.659148609483054, 183.5973147963038059 ) ) ;
#68613=CARTESIAN_POINT ( 'NONE',  ( 32.99911596133222247, 1524.244163922423922, 196.1627191131775874 ) ) ;
#68616=CARTESIAN_POINT ( 'NONE',  ( -16.78480385485708481, 1526.748660780343471, 181.5273693450638746 ) ) ;
#68617=EDGE_CURVE ( 'NONE', #4488, #39734, #73999, .T. ) ;
#68625=ADVANCED_FACE ( 'NONE', ( #108130 ), #65606, .T. ) ;
#68629=ORIENTED_EDGE ( 'NONE', *, *, #50135, .T. ) ;
#68639=CARTESIAN_POINT ( 'NONE',  ( -2.534335827540430852, 1523.982201850120191, 242.5731047040207784 ) ) ;
#68655=CARTESIAN_POINT ( 'NONE',  ( 16.66936639845652834, 1523.382868172864164, 237.7608804993219280 ) ) ;
#68666=EDGE_LOOP ( 'NONE', ( #77755, #19360, #86393, #7680 ) ) ;
#68668=CARTESIAN_POINT ( 'NONE',  ( -21.38516915557943321, 1512.187213306747481, 237.8497028174240313 ) ) ;
#68692=CIRCLE ( 'NONE', #43657, 1.000000000000000888 ) ;
#68694=CARTESIAN_POINT ( 'NONE',  ( -30.15498091547243575, 1525.730671948510917, 221.2486426791599001 ) ) ;
#68710=ADVANCED_FACE ( 'NONE', ( #84034 ), #42756, .T. ) ;
#68721=AXIS2_PLACEMENT_3D ( 'NONE', #92739, #61261, #53961 ) ;
#68723=VERTEX_POINT ( 'NONE', #41496 ) ;
#68725=FACE_OUTER_BOUND ( 'NONE', #6286, .T. ) ;
#68726=CARTESIAN_POINT ( 'NONE',  ( 2.700443415718799312, 1524.678872986499300, 176.3824881451254782 ) ) ;
#68729=CARTESIAN_POINT ( 'NONE',  ( -21.76694865736933693, 1524.152444737676660, 234.8391306143355166 ) ) ;
#68731=DIRECTION ( 'NONE',  ( 0.000000000000000000, 1.000000000000000000, 0.000000000000000000 ) ) ;
#68749=ADVANCED_FACE ( 'NONE', ( #25209 ), #68925, .T. ) ;
#68761=ORIENTED_EDGE ( 'NONE', *, *, #25557, .T. ) ;
#68765=CARTESIAN_POINT ( 'NONE',  ( -31.64580750758060645, 1523.313115944345327, 196.3083633854965626 ) ) ;
#68767=DIRECTION ( 'NONE',  ( 0.7454942576402815435, 0.000000000000000000, 0.6665120492724536660 ) ) ;
#68776=CARTESIAN_POINT ( 'NONE',  ( 16.78480385485652704, 1526.748660780343471, 181.5273693450637040 ) ) ;
#68788=CARTESIAN_POINT ( 'NONE',  ( 3.687149994097108433E-15, 1522.051704408389924, 239.2297105040643714 ) ) ;
#68807=VERTEX_POINT ( 'NONE', #101922 ) ;
#68809=CARTESIAN_POINT ( 'NONE',  ( -2.385609657825171315, 1525.697946996622932, 177.1458771778526398 ) ) ;
#68854=LINE ( 'NONE', #102958, #28298 ) ;
#68859=TOROIDAL_SURFACE ( 'NONE', #102536, 32.13701971169416538, 1.000000000000000000 ) ;
#68897=CARTESIAN_POINT ( 'NONE',  ( -32.05679137160737469, 1524.478200376968744, 216.6895106740730625 ) ) ;
#68904=CARTESIAN_POINT ( 'NONE',  ( -21.96543842109140954, 1523.313115944345100, 235.2592135320311399 ) ) ;
#68911=EDGE_CURVE ( 'NONE', #80799, #4488, #105589, .T. ) ;
#68913=CYLINDRICAL_SURFACE ( 'NONE', #68032, 1.000000000000000888 ) ;
#68914=ORIENTED_EDGE ( 'NONE', *, *, #63819, .T. ) ;
#68920=ADVANCED_FACE ( 'NONE', ( #43697 ), #32060, .T. ) ;
#68924=DIRECTION ( 'NONE',  ( -0.000000000000000000, -1.000000000000000000, -0.000000000000000000 ) ) ;
#68925=CYLINDRICAL_SURFACE ( 'NONE', #9012, 0.9999999999999880096 ) ;
#68928=DIRECTION ( 'NONE',  ( 0.000000000000000000, 1.000000000000000000, 0.000000000000000000 ) ) ;
#68963=DIRECTION ( 'NONE',  ( 0.000000000000000000, -0.8724564897876813108, -0.4886917979947663637 ) ) ;
#68978=ORIENTED_EDGE ( 'NONE', *, *, #105169, .T. ) ;
#69000=FACE_OUTER_BOUND ( 'NONE', #1685, .T. ) ;
#69008=CARTESIAN_POINT ( 'NONE',  ( -1.191524307911315583, 1526.382868172863937, 239.2353018730792087 ) ) ;
#69026=CARTESIAN_POINT ( 'NONE',  ( 3.024787391539412425E-15, 1523.051704408389696, 184.4225825198192013 ) ) ;
#69039=CARTESIAN_POINT ( 'NONE',  ( -30.24977872777067844, 1524.075132568165145, 195.7694483101574008 ) ) ;
#69040=CARTESIAN_POINT ( 'NONE',  ( 32.86470158750937998, 1523.580203803270933, 201.0415738342970542 ) ) ;
#69057=CARTESIAN_POINT ( 'NONE',  ( 16.66231036550701461, 1523.604703353109926, 180.4882076302513099 ) ) ;
#69071=DIRECTION ( 'NONE',  ( -0.8090169943749422332, -0.000000000000000000, 0.5877852522924802425 ) ) ;
#69075=EDGE_LOOP ( 'NONE', ( #4962, #25698 ) ) ;
#69096=ORIENTED_EDGE ( 'NONE', *, *, #13827, .F. ) ;
#69107=EDGE_LOOP ( 'NONE', ( #71073, #30315, #4025, #24637 ) ) ;
#69114=LINE ( 'NONE', #66904, #23068 ) ;
#69129=CARTESIAN_POINT ( 'NONE',  ( 30.38265071698929276, 1524.478200376951008, 221.8419858056983571 ) ) ;
#69149=CARTESIAN_POINT ( 'NONE',  ( 0.000000000000000000, 1526.382868172863937, 209.1218459616979999 ) ) ;
#69161=CARTESIAN_POINT ( 'NONE',  ( -22.08327125186962192, 1523.604703353109699, 184.4267662568474009 ) ) ;
#69165=CARTESIAN_POINT ( 'NONE',  ( 32.41382812665797530, 1525.581535527371216, 197.9832485531609905 ) ) ;
#69169=AXIS2_PLACEMENT_3D ( 'NONE', #81380, #56762, #90900 ) ;
#69170=DIRECTION ( 'NONE',  ( 0.000000000000000000, 1.000000000000000000, 0.000000000000000000 ) ) ;
#69179=VERTEX_POINT ( 'NONE', #50864 ) ;
#69213=ORIENTED_EDGE ( 'NONE', *, *, #47656, .T. ) ;
#69214=ORIENTED_EDGE ( 'NONE', *, *, #94562, .F. ) ;
#69215=PLANE ( 'NONE',  #62706 ) ;
#69221=DIRECTION ( 'NONE',  ( 0.4978433412588729179, 0.000000000000000000, 0.8672669759446635096 ) ) ;
#69230=CIRCLE ( 'NONE', #83502, 1.000000000000000888 ) ;
#69241=DIRECTION ( 'NONE',  ( 0.000000000000000000, 1.000000000000000000, 0.000000000000000000 ) ) ;
#69245=CIRCLE ( 'NONE', #15562, 1.000000000000000888 ) ;
#69247=CARTESIAN_POINT ( 'NONE',  ( -29.91208173166754847, 1525.042337199239910, 222.1821013135304668 ) ) ;
#69249=EDGE_LOOP ( 'NONE', ( #104377, #96633, #155, #106143 ) ) ;
#69264=LINE ( 'NONE', #103370, #107711 ) ;
#69278=CARTESIAN_POINT ( 'NONE',  ( -33.28034951413770415, 1522.644714754858114, 200.8029765415151928 ) ) ;
#69291=B_SPLINE_CURVE_WITH_KNOTS ( 'NONE', 3,
 ( #75092, #100276, #23556, #109780 ),
 .UNSPECIFIED., .F., .F.,
 ( 4, 4 ),
 ( 0.000000000000000000, 0.0002220129587134779374 ),
 .UNSPECIFIED. ) ;
#69294=CARTESIAN_POINT ( 'NONE',  ( -1.435939366445312615, 1526.382868172863937, 178.7444848717731531 ) ) ;
#69311=CARTESIAN_POINT ( 'NONE',  ( 30.31643683089993857, 1523.530935881284904, 222.4932308532203820 ) ) ;
#69315=CARTESIAN_POINT ( 'NONE',  ( 30.30078187369536380, 1526.189899547014420, 201.5450365910303390 ) ) ;
#69316=CARTESIAN_POINT ( 'NONE',  ( -31.81407709660785699, 1522.382868172863937, 196.2902540610632229 ) ) ;
#69319=DIRECTION ( 'NONE',  ( -0.5877852522924802425, 0.000000000000000000, -0.8090169943749422332 ) ) ;
#69330=AXIS2_PLACEMENT_3D ( 'NONE', #88348, #69921, #18908 ) ;
#69340=PLANE ( 'NONE',  #71591 ) ;
#69347=CARTESIAN_POINT ( 'NONE',  ( 17.17241001986506177, 1523.382868172864164, 238.6251415217915053 ) ) ;
#69358=ORIENTED_EDGE ( 'NONE', *, *, #72068, .F. ) ;
#69360=CARTESIAN_POINT ( 'NONE',  ( -2.389876875773859322, 1525.253972588464876, 176.1934926369094399 ) ) ;
#69367=CARTESIAN_POINT ( 'NONE',  ( 16.66936639845652834, 1523.382868172864164, 237.7608804993219280 ) ) ;
#69368=CARTESIAN_POINT ( 'NONE',  ( 20.92767404034497147, 1512.187213306747481, 182.8548762971663848 ) ) ;
#69376=EDGE_LOOP ( 'NONE', ( #77770, #44058, #36680, #55710, #51853, #3809, #79908, #109618 ) ) ;
#69381=CIRCLE ( 'NONE', #24629, 0.9999999999999995559 ) ;
#69405=TOROIDAL_SURFACE ( 'NONE', #21073, 2.000000000000000000, 1.000000000000000000 ) ;
#69415=VECTOR ( 'NONE', #77405, 1000.000000000000000 ) ;
#69442=ORIENTED_EDGE ( 'NONE', *, *, #63186, .T. ) ;
#69446=CARTESIAN_POINT ( 'NONE',  ( -31.65140982495776711, 1525.320827368861046, 216.1854560261664631 ) ) ;
#69463=DIRECTION ( 'NONE',  ( -0.000000000000000000, -1.000000000000000000, -0.000000000000000000 ) ) ;
#69475=CARTESIAN_POINT ( 'NONE',  ( -31.97743984922245275, 1525.878013734321485, 220.1676294520837303 ) ) ;
#69483=CARTESIAN_POINT ( 'NONE',  ( -2.485536261606702269, 1523.919934424249959, 175.4381607306359570 ) ) ;
#69489=LINE ( 'NONE', #42605, #18724 ) ;
#69491=AXIS2_PLACEMENT_3D ( 'NONE', #89193, #78595, #79712 ) ;
#69514=EDGE_CURVE ( 'NONE', #91380, #72816, #23142, .T. ) ;
#69519=CARTESIAN_POINT ( 'NONE',  ( 3.448830483803570157, 1523.382868172864164, 175.1594891075192493 ) ) ;
#69531=CARTESIAN_POINT ( 'NONE',  ( -19.37374569213905318, 1524.382868172863937, 234.3668155954421479 ) ) ;
#69533=CARTESIAN_POINT ( 'NONE',  ( 29.73378234562457934, 1526.349684470114653, 201.0212898931769985 ) ) ;
#69553=CARTESIAN_POINT ( 'NONE',  ( -19.07966196791950608, 1524.244163922423695, 179.2412984082268679 ) ) ;
#69556=LINE ( 'NONE', #25839, #6236 ) ;
#69583=DIRECTION ( 'NONE',  ( 1.224646799147353454E-16, 0.000000000000000000, -1.000000000000000000 ) ) ;
#69595=CARTESIAN_POINT ( 'NONE',  ( -31.16641183314643015, 1524.201816949778276, 196.3723131635786672 ) ) ;
#69631=ORIENTED_EDGE ( 'NONE', *, *, #47977, .T. ) ;
#69632=ORIENTED_EDGE ( 'NONE', *, *, #21409, .F. ) ;
#69634=CARTESIAN_POINT ( 'NONE',  ( 21.39303731107166939, 1524.776010967693765, 184.2561860187820741 ) ) ;
#69669=ORIENTED_EDGE ( 'NONE', *, *, #35083, .F. ) ;
#69686=VECTOR ( 'NONE', #82596, 1000.000000000000000 ) ;
#69695=FACE_OUTER_BOUND ( 'NONE', #69249, .T. ) ;
#69708=ORIENTED_EDGE ( 'NONE', *, *, #69990, .F. ) ;
#69716=CARTESIAN_POINT ( 'NONE',  ( 0.4151546846821903003, 1512.187213306747481, 242.9330574173806951 ) ) ;
#69726=CARTESIAN_POINT ( 'NONE',  ( 19.36857742237545210, 1526.335487865669620, 185.3207153282587285 ) ) ;
#69728=CARTESIAN_POINT ( 'NONE',  ( 0.000000000000000000, 1523.382868172864164, 209.1218459616979999 ) ) ;
#69732=CARTESIAN_POINT ( 'NONE',  ( -31.76119286153750920, 1522.906363951597314, 196.2959455099806121 ) ) ;
#69740=ORIENTED_EDGE ( 'NONE', *, *, #53428, .T. ) ;
#69744=ORIENTED_EDGE ( 'NONE', *, *, #106995, .T. ) ;
#69749=CARTESIAN_POINT ( 'NONE',  ( 3.348648543330357441, 1523.530935881284904, 176.1572159930114196 ) ) ;
#69751=AXIS2_PLACEMENT_3D ( 'NONE', #59960, #94075, #43691 ) ;
#69768=CARTESIAN_POINT ( 'NONE',  ( -32.38114538885259464, 1523.604703353109926, 202.1233279672533172 ) ) ;
#69780=ORIENTED_EDGE ( 'NONE', *, *, #74301, .T. ) ;
#69805=AXIS2_PLACEMENT_3D ( 'NONE', #21326, #22422, #14039 ) ;
#69826=EDGE_CURVE ( 'NONE', #8681, #41836, #70693, .T. ) ;
#69831=VERTEX_POINT ( 'NONE', #23935 ) ;
#69833=DIRECTION ( 'NONE',  ( 0.000000000000000000, 0.07593562622321022026, -0.9971127221483482295 ) ) ;
#69838=CARTESIAN_POINT ( 'NONE',  ( -33.23421991949620491, 1522.906363951597314, 200.8294566360699491 ) ) ;
#69849=ORIENTED_EDGE ( 'NONE', *, *, #1753, .T. ) ;
#69854=FACE_OUTER_BOUND ( 'NONE', #62545, .T. ) ;
#69855=CARTESIAN_POINT ( 'NONE',  ( 29.36670733772781361, 1526.000688113810384, 220.9053709889059576 ) ) ;
#69868=AXIS2_PLACEMENT_3D ( 'NONE', #52407, #79258, #86532 ) ;
#69875=DIRECTION ( 'NONE',  ( 0.000000000000000000, 1.000000000000000000, 0.000000000000000000 ) ) ;
#69888=AXIS2_PLACEMENT_3D ( 'NONE', #22612, #82570, #48428 ) ;
#69889=CARTESIAN_POINT ( 'NONE',  ( 3.351006924987864455, 1524.082582765195411, 242.0157322279995071 ) ) ;
#69895=ADVANCED_FACE ( 'NONE', ( #69854 ), #39215, .T. ) ;
#69901=DIRECTION ( 'NONE',  ( 0.000000000000000000, 0.000000000000000000, 1.000000000000000000 ) ) ;
#69908=DIRECTION ( 'NONE',  ( 0.000000000000000000, -1.000000000000000000, -0.000000000000000000 ) ) ;
#69909=ORIENTED_EDGE ( 'NONE', *, *, #88612, .F. ) ;
#69921=DIRECTION ( 'NONE',  ( 0.8672669759446700599, 0.000000000000000000, 0.4978433412588614271 ) ) ;
#69939=CARTESIAN_POINT ( 'NONE',  ( -3.448830483803561719, 1523.382868172864164, 175.1594891075192209 ) ) ;
#69955=CARTESIAN_POINT ( 'NONE',  ( -33.35590117750204087, 1523.678648413191695, 201.9126545693505648 ) ) ;
#69965=ADVANCED_FACE ( 'NONE', ( #105651 ), #77845, .F. ) ;
#69967=CARTESIAN_POINT ( 'NONE',  ( 2.494564929293782818, 1524.201670966335769, 242.7027287329880210 ) ) ;
#69968=ORIENTED_EDGE ( 'NONE', *, *, #100788, .F. ) ;
#69969=DIRECTION ( 'NONE',  ( 0.9786619618251627406, 0.000000000000000000, 0.2054769195713317953 ) ) ;
#69970=CARTESIAN_POINT ( 'NONE',  ( 20.60985939166236491, 1525.581535527370988, 236.5072125268897025 ) ) ;
#69972=DIRECTION ( 'NONE',  ( -0.8090169943749419001, 0.000000000000000000, 0.5877852522924809087 ) ) ;
#69974=AXIS2_PLACEMENT_3D ( 'NONE', #44130, #86664, #78265 ) ;
#69990=EDGE_CURVE ( 'NONE', #49802, #29937, #11029, .T. ) ;
#70010=AXIS2_PLACEMENT_3D ( 'NONE', #110154, #49166, #16608 ) ;
#70023=ORIENTED_EDGE ( 'NONE', *, *, #6434, .T. ) ;
#70025=EDGE_CURVE ( 'NONE', #22340, #4524, #79362, .T. ) ;
#70036=CARTESIAN_POINT ( 'NONE',  ( -30.29630067237475188, 1526.329757971584741, 221.7900933993811066 ) ) ;
#70038=CARTESIAN_POINT ( 'NONE',  ( 32.32092748916883096, 1524.075132568165600, 202.1437887561546347 ) ) ;
#70039=CARTESIAN_POINT ( 'NONE',  ( 0.000000000000000000, 1526.382868172863937, 209.1218459616979999 ) ) ;
#70060=CARTESIAN_POINT ( 'NONE',  ( 32.28466283162156714, 1522.382868172863937, 219.1752493337713190 ) ) ;
#70084=VERTEX_POINT ( 'NONE', #75359 ) ;
#70092=DIRECTION ( 'NONE',  ( 0.000000000000000000, 1.000000000000000000, 0.000000000000000000 ) ) ;
#70111=AXIS2_PLACEMENT_3D ( 'NONE', #38808, #12519, #46697 ) ;
#70113=CARTESIAN_POINT ( 'NONE',  ( -20.37381179411481469, 1524.397344074318880, 180.2832293763214864 ) ) ;
#70115=DIRECTION ( 'NONE',  ( 0.000000000000000000, 0.000000000000000000, -1.000000000000000000 ) ) ;
#70135=CARTESIAN_POINT ( 'NONE',  ( -34.68852446352570951, 1522.861859112239244, 218.2490599185902624 ) ) ;
#70141=CARTESIAN_POINT ( 'NONE',  ( 32.02808312589916540, 1512.187213306747481, 198.2787714533495489 ) ) ;
#70148=CARTESIAN_POINT ( 'NONE',  ( 18.51436573157358723, 1512.187213306747481, 181.1015051776552696 ) ) ;
#70153=ORIENTED_EDGE ( 'NONE', *, *, #67288, .F. ) ;
#70159=CARTESIAN_POINT ( 'NONE',  ( -29.53442096303453823, 1525.651285554135484, 196.5125176505563900 ) ) ;
#70198=ORIENTED_EDGE ( 'NONE', *, *, #101461, .F. ) ;
#70199=ORIENTED_EDGE ( 'NONE', *, *, #5619, .T. ) ;
#70201=CARTESIAN_POINT ( 'NONE',  ( 20.53760542139772838, 1525.821544997590991, 184.7213720461152775 ) ) ;
#70219=DIRECTION ( 'NONE',  ( 0.9510565162951518658, 0.000000000000000000, -0.3090169943749528914 ) ) ;
#70257=CARTESIAN_POINT ( 'NONE',  ( -16.99777429700792553, 1524.964158026965606, 237.0504674185739873 ) ) ;
#70259=CARTESIAN_POINT ( 'NONE',  ( 30.45769963430792515, 1526.208281990539263, 217.1507671409962370 ) ) ;
#70268=ORIENTED_EDGE ( 'NONE', *, *, #48922, .T. ) ;
#70292=CARTESIAN_POINT ( 'NONE',  ( -30.29630067237287250, 1526.329757971584968, 196.4535985240159448 ) ) ;
#70319=EDGE_LOOP ( 'NONE', ( #45349, #63355, #12063, #72910 ) ) ;
#70326=EDGE_CURVE ( 'NONE', #32377, #5789, #101338, .T. ) ;
#70335=ORIENTED_EDGE ( 'NONE', *, *, #31801, .F. ) ;
#70337=CARTESIAN_POINT ( 'NONE',  ( 20.85167060786188742, 1525.730671948510462, 234.0535507870877439 ) ) ;
#70365=CARTESIAN_POINT ( 'NONE',  ( -29.86283313086175539, 1525.137881624895272, 222.1297143728456263 ) ) ;
#70368=ORIENTED_EDGE ( 'NONE', *, *, #22749, .T. ) ;
#70371=( BOUNDED_CURVE ( )  B_SPLINE_CURVE ( 3, ( #10490, #44661, #68765, #26165 ),
 .UNSPECIFIED., .F., .F. ) 
 B_SPLINE_CURVE_WITH_KNOTS ( ( 4, 4 ),
 ( 0.000000000000000000, 0.7048113239778103223 ),
 .UNSPECIFIED. ) 
 CURVE ( )  GEOMETRIC_REPRESENTATION_ITEM ( )  RATIONAL_B_SPLINE_CURVE ( ( 1.000000000000000000, 0.9590300661663088144, 0.9590300661663088144, 1.000000000000000000 ) ) 
 REPRESENTATION_ITEM ( '' )  );
#70380=CARTESIAN_POINT ( 'NONE',  ( 33.93019615848946557, 1512.187213306747481, 197.6607374645996060 ) ) ;
#70386=ORIENTED_EDGE ( 'NONE', *, *, #43461, .T. ) ;
#70398=CARTESIAN_POINT ( 'NONE',  ( -28.96739426325758870, 1526.189892541618974, 220.8024485780730686 ) ) ;
#70420=CARTESIAN_POINT ( 'NONE',  ( -32.37018134260411983, 1512.187213306747481, 200.1723992780599986 ) ) ;
#70430=CARTESIAN_POINT ( 'NONE',  ( 31.81407709660777527, 1522.382868172863937, 221.9534378623329758 ) ) ;
#70466=CARTESIAN_POINT ( 'NONE',  ( -2.470168521978398424, 1523.382868172864164, 242.8787258963054683 ) ) ;
#70468=AXIS2_PLACEMENT_3D ( 'NONE', #47940, #82075, #14316 ) ;
#70479=ORIENTED_EDGE ( 'NONE', *, *, #55265, .F. ) ;
#70482=AXIS2_PLACEMENT_3D ( 'NONE', #12867, #3950, #81171 ) ;
#70486=ORIENTED_EDGE ( 'NONE', *, *, #3750, .T. ) ;
#70492=CARTESIAN_POINT ( 'NONE',  ( 2.472529913803022783, 1523.678648413191695, 175.3762130535718597 ) ) ;
#70521=ORIENTED_EDGE ( 'NONE', *, *, #110431, .T. ) ;
#70539=CARTESIAN_POINT ( 'NONE',  ( -1.590879946456773775, 1526.333389947990099, 239.8456008596675133 ) ) ;
#70555=CARTESIAN_POINT ( 'NONE',  ( -32.54480841269623426, 1524.547873515804895, 217.0832791832422686 ) ) ;
#70580=CARTESIAN_POINT ( 'NONE',  ( -30.31404213106216972, 1524.330813522192102, 221.7920027509183001 ) ) ;
#70582=CARTESIAN_POINT ( 'NONE',  ( 32.22536377336272295, 1523.621879633028584, 201.4085774011528542 ) ) ;
#70586=DIRECTION ( 'NONE',  ( 0.7414773880254614813, 0.000000000000000000, -0.6709778558543786353 ) ) ;
#70613=ORIENTED_EDGE ( 'NONE', *, *, #52925, .F. ) ;
#70614=AXIS2_PLACEMENT_3D ( 'NONE', #96242, #36325, #18401 ) ;
#70616=DIRECTION ( 'NONE',  ( 0.9510565162951566398, 0.000000000000000000, -0.3090169943749382919 ) ) ;
#70620=AXIS2_PLACEMENT_3D ( 'NONE', #87436, #1795, #70115 ) ;
#70635=ADVANCED_FACE ( 'NONE', ( #31829 ), #58979, .T. ) ;
#70642=ADVANCED_FACE ( 'NONE', ( #66016 ), #31278, .T. ) ;
#70651=EDGE_CURVE ( 'NONE', #56488, #101252, #12821, .T. ) ;
#70663=CARTESIAN_POINT ( 'NONE',  ( -21.11882185303258908, 1525.651285554113201, 233.3142527378166164 ) ) ;
#70675=EDGE_CURVE ( 'NONE', #9501, #77376, #55372, .T. ) ;
#70685=CARTESIAN_POINT ( 'NONE',  ( -30.99338347248342629, 1526.382868172863937, 218.3719692838073740 ) ) ;
#70687=EDGE_CURVE ( 'NONE', #81018, #36007, #21792, .T. ) ;
#70693=( BOUNDED_CURVE ( )  B_SPLINE_CURVE ( 3, ( #31805, #16084, #14986, #65994 ),
 .UNSPECIFIED., .F., .F. ) 
 B_SPLINE_CURVE_WITH_KNOTS ( ( 4, 4 ),
 ( 2.436781329611986457, 3.141592653589793116 ),
 .UNSPECIFIED. ) 
 CURVE ( )  GEOMETRIC_REPRESENTATION_ITEM ( )  RATIONAL_B_SPLINE_CURVE ( ( 1.000000000000000000, 0.9590300661663091475, 0.9590300661663091475, 1.000000000000000000 ) ) 
 REPRESENTATION_ITEM ( '' )  );
#70700=DIRECTION ( 'NONE',  ( 0.6709778558543747495, 0.000000000000000000, 0.7414773880254650340 ) ) ;
#70709=CARTESIAN_POINT ( 'NONE',  ( 20.21716934225403506, 1526.104292489126237, 233.6939662645254430 ) ) ;
#70715=EDGE_CURVE ( 'NONE', #237, #65949, #78668, .T. ) ;
#70719=CIRCLE ( 'NONE', #27751, 1.000000000000003553 ) ;
#70733=FACE_OUTER_BOUND ( 'NONE', #32063, .T. ) ;
#70761=AXIS2_PLACEMENT_3D ( 'NONE', #110649, #92744, #101129 ) ;
#70767=CARTESIAN_POINT ( 'NONE',  ( 32.28466283162151029, 1501.977400791986611, 199.0684425896244250 ) ) ;
#70776=DIRECTION ( 'NONE',  ( -0.000000000000000000, 1.000000000000000000, -0.000000000000000000 ) ) ;
#70779=ADVANCED_FACE ( 'NONE', ( #67664 ), #62855, .F. ) ;
#70802=CARTESIAN_POINT ( 'NONE',  ( -31.93052144186258445, 1525.394057003703438, 217.0185065382337655 ) ) ;
#70809=CARTESIAN_POINT ( 'NONE',  ( 30.12442103006196348, 1524.524650307242382, 222.3821565184462372 ) ) ;
#70811=ORIENTED_EDGE ( 'NONE', *, *, #65090, .F. ) ;
#70812=CARTESIAN_POINT ( 'NONE',  ( -16.48400364723607936, 1525.790286462510494, 236.4799666439590169 ) ) ;
#70826=EDGE_CURVE ( 'NONE', #72142, #1895, #24887, .T. ) ;
#70840=( BOUNDED_CURVE ( )  B_SPLINE_CURVE ( 3, ( #38566, #97919, #90067, #73851 ),
 .UNSPECIFIED., .F., .T. ) 
 B_SPLINE_CURVE_WITH_KNOTS ( ( 4, 4 ),
 ( 0.000000000000000000, 0.7048113239778113215 ),
 .UNSPECIFIED. ) 
 CURVE ( )  GEOMETRIC_REPRESENTATION_ITEM ( )  RATIONAL_B_SPLINE_CURVE ( ( 1.000000000000000000, 0.9590300661663084814, 0.9590300661663084814, 1.000000000000000000 ) ) 
 REPRESENTATION_ITEM ( '' )  );
#70842=CARTESIAN_POINT ( 'NONE',  ( 18.66420869458043796, 1526.382868172863937, 185.4599087859680537 ) ) ;
#70851=CARTESIAN_POINT ( 'NONE',  ( 32.02808312589916540, 1512.187213306747481, 197.2787714533495489 ) ) ;
#70873=ORIENTED_EDGE ( 'NONE', *, *, #13686, .T. ) ;
#70876=DIRECTION ( 'NONE',  ( 0.000000000000000000, 0.000000000000000000, 1.000000000000000000 ) ) ;
#70894=ORIENTED_EDGE ( 'NONE', *, *, #41795, .T. ) ;
#70910=EDGE_CURVE ( 'NONE', #80823, #71507, #48425, .T. ) ;
#70912=ORIENTED_EDGE ( 'NONE', *, *, #105169, .F. ) ;
#70925=CARTESIAN_POINT ( 'NONE',  ( -31.25789155969114219, 1523.954914175594695, 221.8935806748798711 ) ) ;
#70947=CARTESIAN_POINT ( 'NONE',  ( -19.29371659517392601, 1526.349689584397083, 185.0912979150474200 ) ) ;
#70954=CARTESIAN_POINT ( 'NONE',  ( -34.18677586421046044, 1522.906561336852974, 198.4504086008704746 ) ) ;
#70957=CARTESIAN_POINT ( 'NONE',  ( 30.51231035492518728, 1526.382868172863937, 200.0858385050239008 ) ) ;
#70968=CARTESIAN_POINT ( 'NONE',  ( 30.30080019752885434, 1526.189892541618974, 216.6986470857947609 ) ) ;
#70982=VERTEX_POINT ( 'NONE', #76327 ) ;
#70985=DIRECTION ( 'NONE',  ( 0.5877852522924634782, 0.000000000000000000, -0.8090169943749544457 ) ) ;
#71002=CARTESIAN_POINT ( 'NONE',  ( 3.059301852550817102, 1525.343727714918259, 241.3958358433001479 ) ) ;
#71013=CIRCLE ( 'NONE', #26528, 1.000000000000000888 ) ;
#71025=AXIS2_PLACEMENT_3D ( 'NONE', #7975, #25308, #93618 ) ;
#71027=ORIENTED_EDGE ( 'NONE', *, *, #50135, .F. ) ;
#71054=EDGE_LOOP ( 'NONE', ( #45537, #102385, #92435, #64168, #110037 ) ) ;
#71065=DIRECTION ( 'NONE',  ( 0.9510565162951561957, 0.000000000000000000, 0.3090169943749392911 ) ) ;
#71068=DIRECTION ( 'NONE',  ( 0.9786619618251657382, 0.000000000000000000, 0.2054769195713179730 ) ) ;
#71072=CARTESIAN_POINT ( 'NONE',  ( 2.487421823092354156, 1523.954914175591739, 242.7965504892020192 ) ) ;
#71073=ORIENTED_EDGE ( 'NONE', *, *, #63601, .T. ) ;
#71082=CARTESIAN_POINT ( 'NONE',  ( -28.27139721233055170, 1526.382868172863937, 198.6830693683576214 ) ) ;
#71087=CARTESIAN_POINT ( 'NONE',  ( -31.79839622030619495, 1525.159196711359755, 202.0929531505411489 ) ) ;
#71097=CARTESIAN_POINT ( 'NONE',  ( 29.99620953741496976, 1526.382868172863937, 219.7462484079458704 ) ) ;
#71098=DIRECTION ( 'NONE',  ( -0.4978433412588703089, 0.000000000000000000, 0.8672669759446649529 ) ) ;
#71105=ORIENTED_EDGE ( 'NONE', *, *, #67624, .T. ) ;
#71128=EDGE_LOOP ( 'NONE', ( #46327, #4043, #107624, #96770 ) ) ;
#71135=CARTESIAN_POINT ( 'NONE',  ( 31.79806488006812870, 1525.506916460682078, 201.2206263324432030 ) ) ;
#71139=DIRECTION ( 'NONE',  ( 0.000000000000000000, 0.000000000000000000, 1.000000000000000000 ) ) ;
#71153=DIRECTION ( 'NONE',  ( 0.000000000000000000, 1.000000000000000000, 0.000000000000000000 ) ) ;
#71164=AXIS2_PLACEMENT_3D ( 'NONE', #81246, #59388, #34707 ) ;
#71170=DIRECTION ( 'NONE',  ( 0.000000000000000000, -1.000000000000000000, 0.000000000000000000 ) ) ;
#71175=AXIS2_PLACEMENT_3D ( 'NONE', #71578, #2698, #4862 ) ;
#71179=ORIENTED_EDGE ( 'NONE', *, *, #34328, .F. ) ;
#71185=VERTEX_POINT ( 'NONE', #62320 ) ;
#71192=CARTESIAN_POINT ( 'NONE',  ( 32.38114538885255200, 1523.604703353109699, 216.1203639561429100 ) ) ;
#71200=CIRCLE ( 'NONE', #62246, 1.000000000000000888 ) ;
#71203=ORIENTED_EDGE ( 'NONE', *, *, #45214, .T. ) ;
#71209=CARTESIAN_POINT ( 'NONE',  ( -17.89234610336760412, 1523.611961620354123, 180.3157245011626912 ) ) ;
#71236=CARTESIAN_POINT ( 'NONE',  ( 32.85805783624312681, 1523.678648413191695, 217.1983043299902931 ) ) ;
#71259=FACE_OUTER_BOUND ( 'NONE', #81876, .T. ) ;
#71260=DIRECTION ( 'NONE',  ( 0.000000000000000000, 0.000000000000000000, -1.000000000000000000 ) ) ;
#71265=CIRCLE ( 'NONE', #12224, 1.000000000000000888 ) ;
#71277=CARTESIAN_POINT ( 'NONE',  ( 16.66936639845631873, 1523.456872492435195, 180.4828114240739581 ) ) ;
#71278=CARTESIAN_POINT ( 'NONE',  ( 2.372478608332516892, 1501.977400791986611, 243.3440112565233449 ) ) ;
#71298=ORIENTED_EDGE ( 'NONE', *, *, #101981, .F. ) ;
#71317=ORIENTED_EDGE ( 'NONE', *, *, #52115, .F. ) ;
#71334=ORIENTED_EDGE ( 'NONE', *, *, #106995, .F. ) ;
#71339=ORIENTED_EDGE ( 'NONE', *, *, #1464, .F. ) ;
#71342=DIRECTION ( 'NONE',  ( 0.000000000000000000, 0.000000000000000000, 1.000000000000000000 ) ) ;
#71366=CARTESIAN_POINT ( 'NONE',  ( -17.53714238134516279, 1524.871836253796346, 237.4423643566621536 ) ) ;
#71381=EDGE_CURVE ( 'NONE', #83342, #21777, #50027, .T. ) ;
#71392=CARTESIAN_POINT ( 'NONE',  ( -21.75649307329753768, 1524.201670966335769, 183.4206095899358218 ) ) ;
#71433=VERTEX_POINT ( 'NONE', #57634 ) ;
#71434=ORIENTED_EDGE ( 'NONE', *, *, #58534, .T. ) ;
#71443=DIRECTION ( 'NONE',  ( 0.5877852522924743583, 0.000000000000000000, 0.8090169943749466741 ) ) ;
#71451=CARTESIAN_POINT ( 'NONE',  ( -16.73628186595857059, 1526.382868172864164, 184.0591879540917546 ) ) ;
#71452=CARTESIAN_POINT ( 'NONE',  ( 21.45462491533043803, 1525.320849883649316, 233.4406507496946972 ) ) ;
#71455=VERTEX_POINT ( 'NONE', #82050 ) ;
#71459=EDGE_CURVE ( 'NONE', #92224, #40681, #75132, .T. ) ;
#71470=CARTESIAN_POINT ( 'NONE',  ( 2.469061732649111107, 1524.816846803860926, 175.8590321262562952 ) ) ;
#71481=CARTESIAN_POINT ( 'NONE',  ( -30.29139619033233544, 1523.843263703803814, 222.4926162074647777 ) ) ;
#71496=DIRECTION ( 'NONE',  ( 0.8090169943749422332, -0.000000000000000000, -0.5877852522924802425 ) ) ;
#71497=CARTESIAN_POINT ( 'NONE',  ( -18.51436573157398158, 1511.187213306747708, 181.1015051776554969 ) ) ;
#71499=EDGE_CURVE ( 'NONE', #56418, #44154, #53648, .T. ) ;
#71507=VERTEX_POINT ( 'NONE', #15392 ) ;
#71523=ORIENTED_EDGE ( 'NONE', *, *, #91702, .T. ) ;
#71578=CARTESIAN_POINT ( 'NONE',  ( 31.43069643840511773, 1526.748660780343471, 201.6857111062222998 ) ) ;
#71582=CIRCLE ( 'NONE', #105509, 1.000000000000000888 ) ;
#71584=DIRECTION ( 'NONE',  ( 0.000000000000000000, 0.000000000000000000, 1.000000000000000000 ) ) ;
#71591=AXIS2_PLACEMENT_3D ( 'NONE', #78831, #63169, #86661 ) ;
#71593=EDGE_LOOP ( 'NONE', ( #37862, #31247, #42880 ) ) ;
#71594=CARTESIAN_POINT ( 'NONE',  ( -3.355801963978114255, 1523.843263703804951, 176.1812209933808901 ) ) ;
#71605=ORIENTED_EDGE ( 'NONE', *, *, #95512, .T. ) ;
#71606=ORIENTED_EDGE ( 'NONE', *, *, #81541, .F. ) ;
#71634=DIRECTION ( 'NONE',  ( 0.9510565162951561957, 0.000000000000000000, 0.3090169943749392911 ) ) ;
#71655=AXIS2_PLACEMENT_3D ( 'NONE', #96865, #3371, #44259 ) ;
#71677=DIRECTION ( 'NONE',  ( -0.8090169943749551118, -0.000000000000000000, -0.5877852522924625900 ) ) ;
#71688=CARTESIAN_POINT ( 'NONE',  ( 2.620401159549909487, 1523.382868172863937, 242.1631858340802523 ) ) ;
#71695=EDGE_CURVE ( 'NONE', #70084, #108510, #50117, .T. ) ;
#71705=CARTESIAN_POINT ( 'NONE',  ( 32.21733187661251918, 1523.844789899204898, 201.4553037014809149 ) ) ;
#71711=CARTESIAN_POINT ( 'NONE',  ( 30.90487439922549484, 1525.907212628473644, 201.8101144455178257 ) ) ;
#71731=VERTEX_POINT ( 'NONE', #58463 ) ;
#71738=TOROIDAL_SURFACE ( 'NONE', #107406, 1.000000000000000000, 1.000000000000000000 ) ;
#71741=CARTESIAN_POINT ( 'NONE',  ( 16.83198307404049743, 1526.000688113711703, 235.9162354438186071 ) ) ;
#71742=ORIENTED_EDGE ( 'NONE', *, *, #46715, .T. ) ;
#71753=CARTESIAN_POINT ( 'NONE',  ( 0.5770119038902407071, 1525.581535527370761, 174.8524476110296177 ) ) ;
#71761=FACE_OUTER_BOUND ( 'NONE', #105739, .T. ) ;
#71769=ORIENTED_EDGE ( 'NONE', *, *, #46840, .T. ) ;
#71771=LINE ( 'NONE', #38115, #37269 ) ;
#71773=DIRECTION ( 'NONE',  ( 0.4090087482554383147, 0.000000000000000000, 0.9125304618753937724 ) ) ;
#71779=VECTOR ( 'NONE', #76425, 1000.000000000000114 ) ;
#71815=CARTESIAN_POINT ( 'NONE',  ( 0.000000000000000000, 1526.382868172863937, 209.1218459616979999 ) ) ;
#71817=CARTESIAN_POINT ( 'NONE',  ( -30.57819355944234019, 1525.253996226949539, 196.6735304476125066 ) ) ;
#71820=CARTESIAN_POINT ( 'NONE',  ( 17.17241001986484505, 1523.382868172864164, 179.6185504016043524 ) ) ;
#71826=CARTESIAN_POINT ( 'NONE',  ( -2.620401159549909487, 1523.382868172863937, 176.0805060893157474 ) ) ;
#71827=EDGE_CURVE ( 'NONE', #16710, #33454, #15862, .T. ) ;
#71828=CARTESIAN_POINT ( 'NONE',  ( 19.53786426059039982, 1511.187213306747708, 236.7197124308265188 ) ) ;
#71832=DIRECTION ( 'NONE',  ( 0.4090087482554447540, 1.419034154957372271E-15, 0.9125304618753908859 ) ) ;
#71835=LINE ( 'NONE', #71278, #47933 ) ;
#71845=B_SPLINE_CURVE_WITH_KNOTS ( 'NONE', 3,
 ( #110459, #60635, #103713, #9639, #94760, #77415, #42711, #93633, #85804, #43813 ),
 .UNSPECIFIED., .F., .F.,
 ( 4, 2, 2, 2, 4 ),
 ( 0.000000000000000000, 0.0007189769279726051935, 0.001437953855945210387, 0.002156930783917815689, 0.002875907711890420774 ),
 .UNSPECIFIED. ) ;
#71849=AXIS2_PLACEMENT_3D ( 'NONE', #32927, #103290, #35554 ) ;
#71856=VERTEX_POINT ( 'NONE', #87529 ) ;
#71859=ORIENTED_EDGE ( 'NONE', *, *, #91022, .F. ) ;
#71874=ORIENTED_EDGE ( 'NONE', *, *, #9882, .F. ) ;
#71885=AXIS2_PLACEMENT_3D ( 'NONE', #67901, #27527, #34269 ) ;
#71909=CARTESIAN_POINT ( 'NONE',  ( -32.85805783624297760, 1523.678648413191695, 217.1983043299907763 ) ) ;
#71915=CARTESIAN_POINT ( 'NONE',  ( 30.15498238788762819, 1525.730671215510711, 221.2486442788145382 ) ) ;
#71941=CARTESIAN_POINT ( 'NONE',  ( -22.08327125186963258, 1523.604703353109926, 184.4267662568474009 ) ) ;
#71944=VERTEX_POINT ( 'NONE', #25929 ) ;
#71958=CARTESIAN_POINT ( 'NONE',  ( -20.79738390328697761, 1511.187213306747708, 237.0406858230491025 ) ) ;
#71959=ORIENTED_EDGE ( 'NONE', *, *, #49598, .T. ) ;
#71983=DIRECTION ( 'NONE',  ( 0.000000000000000000, -1.000000000000000000, 0.000000000000000000 ) ) ;
#71984=CARTESIAN_POINT ( 'NONE',  ( -31.34137657907861652, 1523.481610118011986, 196.3411265156833565 ) ) ;
#71985=CARTESIAN_POINT ( 'NONE',  ( 19.39983987835422496, 1501.977400791986611, 239.2921289694223219 ) ) ;
#71988=CARTESIAN_POINT ( 'NONE',  ( 22.03465957474552539, 1512.187213306747481, 182.8300405912328301 ) ) ;
#71997=CARTESIAN_POINT ( 'NONE',  ( 0.000000000000000000, 1511.187213306747708, 179.0139814193315999 ) ) ;
#71999=ADVANCED_FACE ( 'NONE', ( #48839 ), #6255, .T. ) ;
#72008=CARTESIAN_POINT ( 'NONE',  ( -28.54286204732466103, 1526.382868172863937, 219.8009395035764726 ) ) ;
#72013=CARTESIAN_POINT ( 'NONE',  ( 0.000000000000000000, 1523.382868172864164, 209.1218459616979999 ) ) ;
#72016=CARTESIAN_POINT ( 'NONE',  ( 30.31940284292419818, 1523.382868172864164, 222.4933038710543087 ) ) ;
#72028=ORIENTED_EDGE ( 'NONE', *, *, #31527, .F. ) ;
#72062=EDGE_CURVE ( 'NONE', #53799, #57779, #42912, .T. ) ;
#72063=CARTESIAN_POINT ( 'NONE',  ( 0.4681535437661719090, 1524.397344074316607, 244.4282029790948627 ) ) ;
#72068=EDGE_CURVE ( 'NONE', #1550, #36754, #32007, .T. ) ;
#72085=ORIENTED_EDGE ( 'NONE', *, *, #27349, .F. ) ;
#72102=FACE_OUTER_BOUND ( 'NONE', #87553, .T. ) ;
#72106=ORIENTED_EDGE ( 'NONE', *, *, #51036, .F. ) ;
#72116=CARTESIAN_POINT ( 'NONE',  ( -29.85692247043837710, 1525.159196711359755, 222.1259805706810084 ) ) ;
#72130=EDGE_LOOP ( 'NONE', ( #71874, #97023, #48719, #50363 ) ) ;
#72138=FACE_OUTER_BOUND ( 'NONE', #68537, .T. ) ;
#72141=ORIENTED_EDGE ( 'NONE', *, *, #97442, .T. ) ;
#72142=VERTEX_POINT ( 'NONE', #107467 ) ;
#72157=ORIENTED_EDGE ( 'NONE', *, *, #9743, .F. ) ;
#72161=FACE_OUTER_BOUND ( 'NONE', #41545, .T. ) ;
#72169=CARTESIAN_POINT ( 'NONE',  ( 32.02808312589922224, 1501.977400791986611, 219.9649204700462235 ) ) ;
#72190=DIRECTION ( 'NONE',  ( 0.9786619618251632957, 0.000000000000000000, -0.2054769195713296581 ) ) ;
#72191=FACE_OUTER_BOUND ( 'NONE', #49819, .T. ) ;
#72230=CARTESIAN_POINT ( 'NONE',  ( 30.95751052620454402, 1525.821544997590308, 201.4531494772885196 ) ) ;
#72234=CARTESIAN_POINT ( 'NONE',  ( 3.300164695495766853, 1524.538768545233779, 176.3797544596794182 ) ) ;
#72255=ORIENTED_EDGE ( 'NONE', *, *, #97988, .F. ) ;
#72267=ORIENTED_EDGE ( 'NONE', *, *, #39849, .T. ) ;
#72275=CARTESIAN_POINT ( 'NONE',  ( 2.682480990172567470, 1524.330813522192102, 176.3761848884416281 ) ) ;
#72277=CARTESIAN_POINT ( 'NONE',  ( 17.04521562810657187, 1526.211523310372513, 235.5955797450462796 ) ) ;
#72293=AXIS2_PLACEMENT_3D ( 'NONE', #65031, #32525, #50443 ) ;
#72310=CARTESIAN_POINT ( 'NONE',  ( 30.44526109729614305, 1526.211528530236592, 217.1519773718490569 ) ) ;
#72328=CARTESIAN_POINT ( 'NONE',  ( 17.07724394728954209, 1524.330813522192102, 181.0533268958136830 ) ) ;
#72333=ORIENTED_EDGE ( 'NONE', *, *, #39103, .T. ) ;
#72348=CARTESIAN_POINT ( 'NONE',  ( -32.97913964219446115, 1511.187213306747708, 197.9697544589750464 ) ) ;
#72349=CARTESIAN_POINT ( 'NONE',  ( -2.470168522032202940, 1523.481610118012441, 175.3649660273468101 ) ) ;
#72351=EDGE_LOOP ( 'NONE', ( #28581, #55594, #32984, #63314 ) ) ;
#72356=CARTESIAN_POINT ( 'NONE',  ( 33.42844755917195698, 1522.382868172863937, 222.1271778627166213 ) ) ;
#72361=CYLINDRICAL_SURFACE ( 'NONE', #26448, 0.9999999999999865663 ) ;
#72372=ORIENTED_EDGE ( 'NONE', *, *, #69826, .F. ) ;
#72376=ORIENTED_EDGE ( 'NONE', *, *, #47629, .T. ) ;
#72417=CARTESIAN_POINT ( 'NONE',  ( -17.43549085681739541, 1525.211473355384896, 181.0323682579330580 ) ) ;
#72451=EDGE_LOOP ( 'NONE', ( #54220, #64777, #42768 ) ) ;
#72474=CARTESIAN_POINT ( 'NONE',  ( 31.87600794503219603, 1525.042337199240137, 216.1377579384306671 ) ) ;
#72517=CARTESIAN_POINT ( 'NONE',  ( 20.53760542139780298, 1525.821544997590536, 233.5223198772804665 ) ) ;
#72522=CARTESIAN_POINT ( 'NONE',  ( 30.29630067237317803, 1526.329757971585195, 196.4535985240150637 ) ) ;
#72549=AXIS2_PLACEMENT_3D ( 'NONE', #102172, #84813, #34976 ) ;
#72557=FACE_OUTER_BOUND ( 'NONE', #65780, .T. ) ;
#72563=CARTESIAN_POINT ( 'NONE',  ( -19.39983987835443457, 1522.382868172863937, 178.9515629539737631 ) ) ;
#72587=CARTESIAN_POINT ( 'NONE',  ( 2.372478608334043670, 1522.644714754858114, 243.3440112565160973 ) ) ;
#72588=ORIENTED_EDGE ( 'NONE', *, *, #52115, .T. ) ;
#72595=CARTESIAN_POINT ( 'NONE',  ( -3.302346719094112260, 1524.524650307243519, 241.8695341946817337 ) ) ;
#72600=AXIS2_PLACEMENT_3D ( 'NONE', #72013, #27218, #36720 ) ;
#72606=CARTESIAN_POINT ( 'NONE',  ( 32.30068554584606488, 1526.382868172863937, 198.0073124585814242 ) ) ;
#72609=ORIENTED_EDGE ( 'NONE', *, *, #93847, .T. ) ;
#72610=CYLINDRICAL_SURFACE ( 'NONE', #65001, 2.000000000000000888 ) ;
#72625=CARTESIAN_POINT ( 'NONE',  ( 32.36284091028937127, 1525.878013734321257, 199.2622049721660176 ) ) ;
#72629=ORIENTED_EDGE ( 'NONE', *, *, #50933, .F. ) ;
#72637=DIRECTION ( 'NONE',  ( 0.9942586961433758086, 0.000000000000000000, 0.1070030146457303932 ) ) ;
#72638=EDGE_CURVE ( 'NONE', #107075, #29531, #50625, .T. ) ;
#72639=DIRECTION ( 'NONE',  ( 0.9786619618251657382, 0.000000000000000000, 0.2054769195713184449 ) ) ;
#72642=ADVANCED_FACE ( 'NONE', ( #6958 ), #3614, .T. ) ;
#72661=DIRECTION ( 'NONE',  ( -0.8090169943749507819, -0.000000000000000000, -0.5877852522924685852 ) ) ;
#72670=ORIENTED_EDGE ( 'NONE', *, *, #62426, .T. ) ;
#72677=EDGE_CURVE ( 'NONE', #105138, #15491, #55466, .T. ) ;
#72679=CARTESIAN_POINT ( 'NONE',  ( -33.28034951413921760, 1522.382868172863937, 217.4407153818824838 ) ) ;
#72686=ORIENTED_EDGE ( 'NONE', *, *, #89323, .F. ) ;
#72689=ORIENTED_EDGE ( 'NONE', *, *, #6290, .T. ) ;
#72697=CARTESIAN_POINT ( 'NONE',  ( 32.86470156657956920, 1523.580204110583963, 201.0415738463115360 ) ) ;
#72704=DIRECTION ( 'NONE',  ( -0.03173147633638096626, -0.9969860201949397593, 0.07079540200725449595 ) ) ;
#72707=DIRECTION ( 'NONE',  ( -0.1070030146457249254, 0.000000000000000000, 0.9942586961433763637 ) ) ;
#72717=AXIS2_PLACEMENT_3D ( 'NONE', #24421, #101124, #18640 ) ;
#72722=DIRECTION ( 'NONE',  ( 0.000000000000000000, -1.000000000000000000, -0.000000000000000000 ) ) ;
#72750=DIRECTION ( 'NONE',  ( 0.000000000000000000, 0.000000000000000000, -1.000000000000000000 ) ) ;
#72754=DIRECTION ( 'NONE',  ( 0.000000000000000000, 0.000000000000000000, 1.000000000000000000 ) ) ;
#72759=CARTESIAN_POINT ( 'NONE',  ( 17.61183580542362037, 1523.982201850120191, 237.6741279912554035 ) ) ;
#72769=CARTESIAN_POINT ( 'NONE',  ( -3.448830483803564828, 1512.187213306747481, 243.0842028158767789 ) ) ;
#72770=CARTESIAN_POINT ( 'NONE',  ( -3.448830483803564828, 1511.187213306747708, 243.0842028158767789 ) ) ;
#72776=CIRCLE ( 'NONE', #67443, 1.000000000000001554 ) ;
#72801=VERTEX_POINT ( 'NONE', #104 ) ;
#72805=EDGE_CURVE ( 'NONE', #16677, #10257, #85904, .T. ) ;
#72807=CARTESIAN_POINT ( 'NONE',  ( 16.50400130224763018, 1525.907212628473644, 236.2546788475580968 ) ) ;
#72812=VERTEX_POINT ( 'NONE', #87400 ) ;
#72816=VERTEX_POINT ( 'NONE', #34227 ) ;
#72817=CARTESIAN_POINT ( 'NONE',  ( 2.792392588003332232, 1526.382868172863937, 176.8996806668727118 ) ) ;
#72818=FACE_OUTER_BOUND ( 'NONE', #59557, .T. ) ;
#72824=DIRECTION ( 'NONE',  ( 0.000000000000000000, 1.000000000000000000, 0.000000000000000000 ) ) ;
#72827=CARTESIAN_POINT ( 'NONE',  ( 29.67375955053568148, 1525.697946996616565, 196.9718785854857401 ) ) ;
#72841=ORIENTED_EDGE ( 'NONE', *, *, #56365, .F. ) ;
#72860=CARTESIAN_POINT ( 'NONE',  ( -31.32995031131182628, 1523.678648413191695, 221.9013357025048947 ) ) ;
#72865=CARTESIAN_POINT ( 'NONE',  ( 18.37487226820733355, 1526.382868172863937, 182.5038319547554693 ) ) ;
#72876=CARTESIAN_POINT ( 'NONE',  ( 0.000000000000000000, 1523.382868172864164, 209.1218459616979999 ) ) ;
#72888=EDGE_LOOP ( 'NONE', ( #106627, #75921, #78682 ) ) ;
#72893=DIRECTION ( 'NONE',  ( 0.000000000000000000, 1.000000000000000000, 0.000000000000000000 ) ) ;
#72901=CARTESIAN_POINT ( 'NONE',  ( -31.23437356469425907, 1523.382868172864164, 222.8968241038848248 ) ) ;
#72910=ORIENTED_EDGE ( 'NONE', *, *, #37278, .F. ) ;
#72917=ORIENTED_EDGE ( 'NONE', *, *, #40063, .T. ) ;
#72919=EDGE_LOOP ( 'NONE', ( #103060, #3134 ) ) ;
#72928=CARTESIAN_POINT ( 'NONE',  ( 156.6846457583361882, 1526.382868172863937, 340.9912860285725174 ) ) ;
#72978=EDGE_LOOP ( 'NONE', ( #67674, #92822, #33496, #88765, #49975 ) ) ;
#72979=CARTESIAN_POINT ( 'NONE',  ( -1.775988990187477246, 1526.208281990535852, 177.6737791622278451 ) ) ;
#72996=VECTOR ( 'NONE', #84003, 1000.000000000000000 ) ;
#72997=DIRECTION ( 'NONE',  ( 0.000000000000000000, 1.000000000000000000, 0.000000000000000000 ) ) ;
#72998=B_SPLINE_CURVE_WITH_KNOTS ( 'NONE', 3,
 ( #36764, #87165, #9900, #70398, #78207, #3741 ),
 .UNSPECIFIED., .F., .F.,
 ( 4, 2, 4 ),
 ( -1.131363979616252987E-05, 0.001067788114096044532, 0.002146889867988251502 ),
 .UNSPECIFIED. ) ;
#73009=DIRECTION ( 'NONE',  ( -0.000000000000000000, -1.000000000000000000, -0.000000000000000000 ) ) ;
#73014=CARTESIAN_POINT ( 'NONE',  ( -21.12212911286992068, 1512.187213306747481, 235.8226600804187285 ) ) ;
#73019=CARTESIAN_POINT ( 'NONE',  ( 32.13446200735371860, 1525.163457223744444, 217.0282479337336383 ) ) ;
#73050=CARTESIAN_POINT ( 'NONE',  ( 2.372478608332514671, 1512.187213306747481, 174.8996806668726549 ) ) ;
#73063=DIRECTION ( 'NONE',  ( -0.000000000000000000, -1.000000000000000000, -0.000000000000000000 ) ) ;
#73068=CIRCLE ( 'NONE', #31959, 0.9999999999999998890 ) ;
#73070=CARTESIAN_POINT ( 'NONE',  ( -29.61692403811275298, 1526.104292489132376, 197.4873780791112949 ) ) ;
#73096=CARTESIAN_POINT ( 'NONE',  ( 28.27139721233031722, 1526.382868172864164, 198.6830693683572235 ) ) ;
#73118=ORIENTED_EDGE ( 'NONE', *, *, #22303, .F. ) ;
#73136=CARTESIAN_POINT ( 'NONE',  ( 3.348648543330357885, 1523.530935881284904, 242.0864759303845801 ) ) ;
#73140=CARTESIAN_POINT ( 'NONE',  ( -2.708195641334396608, 1524.374578187333100, 241.9868732463102958 ) ) ;
#73145=CARTESIAN_POINT ( 'NONE',  ( 30.31940284292420174, 1518.913060387330006, 222.4933038710543087 ) ) ;
#73152=CARTESIAN_POINT ( 'NONE',  ( -32.28466283162143213, 1512.187213306747481, 219.1752493337717738 ) ) ;
#73156=DIRECTION ( 'NONE',  ( 0.000000000000000000, 1.000000000000000000, 0.000000000000000000 ) ) ;
#73167=CARTESIAN_POINT ( 'NONE',  ( -2.372478608332517336, 1522.382868172863937, 243.3440112565233449 ) ) ;
#73172=CARTESIAN_POINT ( 'NONE',  ( 31.50799703744293367, 1524.382868172863937, 201.8203724569132191 ) ) ;
#73175=VERTEX_POINT ( 'NONE', #5456 ) ;
#73180=DIRECTION ( 'NONE',  ( 0.000000000000000000, 0.000000000000000000, -1.000000000000000000 ) ) ;
#73181=CYLINDRICAL_SURFACE ( 'NONE', #107333, 1.000000000000003109 ) ;
#73196=LINE ( 'NONE', #49659, #88366 ) ;
#73227=DIRECTION ( 'NONE',  ( -0.4035202328300252494, 0.000000000000000000, 0.9149707217702663931 ) ) ;
#73239=CYLINDRICAL_SURFACE ( 'NONE', #102162, 3.999999999999991118 ) ;
#73250=FACE_OUTER_BOUND ( 'NONE', #37384, .T. ) ;
#73264=PLANE ( 'NONE',  #101475 ) ;
#73274=( BOUNDED_SURFACE ( )  B_SPLINE_SURFACE ( 3, 2, ( 
 ( #55545, #12954, #29764 ),
 ( #96993, #30313, #80732 ),
 ( #47135, #7190, #72349 ),
 ( #106478, #71826, #20256 ) ),
 .UNSPECIFIED., .F., .F., .T. ) 
 B_SPLINE_SURFACE_WITH_KNOTS ( ( 4, 4 ),
 ( 3, 3 ),
 ( 0.000000000000000000, 0.0002960034161023844057 ),
 ( 0.000000000000000000, 1.000000000000000000 ),
 .UNSPECIFIED. ) 
 GEOMETRIC_REPRESENTATION_ITEM ( )  RATIONAL_B_SPLINE_SURFACE ( (
 ( 1.000000000000000000, 0.8070209408749940971, 1.000000000000000000),
 ( 1.000000000000000000, 0.8071723757218307593, 1.000000000000000000),
 ( 1.000000000000000000, 0.8072480346917725313, 1.000000000000000000),
 ( 1.000000000000000000, 0.8072480644198083422, 1.000000000000000000) ) ) 
 REPRESENTATION_ITEM ( '' )  SURFACE ( )  );
#73294=CARTESIAN_POINT ( 'NONE',  ( 1.909779004914692990, 1526.107876515966382, 177.3667160767706150 ) ) ;
#73305=CARTESIAN_POINT ( 'NONE',  ( 18.00465857451067819, 1523.390106123591067, 238.0296012445054998 ) ) ;
#73331=VECTOR ( 'NONE', #87534, 1000.000000000000227 ) ;
#73338=DIRECTION ( 'NONE',  ( 0.000000000000000000, 0.000000000000000000, 1.000000000000000000 ) ) ;
#73340=ORIENTED_EDGE ( 'NONE', *, *, #51036, .T. ) ;
#73359=ADVANCED_FACE ( 'NONE', ( #79580 ), #19718, .T. ) ;
#73374=CARTESIAN_POINT ( 'NONE',  ( 30.11859361092137632, 1525.055402519434438, 196.5532433872490969 ) ) ;
#73412=CARTESIAN_POINT ( 'NONE',  ( -31.34137657934000387, 1523.481610426287716, 221.9025654077414345 ) ) ;
#73424=CARTESIAN_POINT ( 'NONE',  ( -17.78112617923709138, 1523.954924407802537, 180.4163696555889658 ) ) ;
#73462=CARTESIAN_POINT ( 'NONE',  ( 17.83486663330506872, 1523.678648413191695, 237.8759530894958800 ) ) ;
#73472=EDGE_CURVE ( 'NONE', #81438, #53391, #46607, .T. ) ;
#73476=CYLINDRICAL_SURFACE ( 'NONE', #104715, 1.000000000000000888 ) ;
#73487=CARTESIAN_POINT ( 'NONE',  ( 0.000000000000000000, 1523.382868172864164, 209.1218459616979999 ) ) ;
#73495=EDGE_CURVE ( 'NONE', #32890, #81031, #50198, .T. ) ;
#73504=CARTESIAN_POINT ( 'NONE',  ( 30.31052258194597115, 1523.604703353109699, 222.4930856806589929 ) ) ;
#73512=AXIS2_PLACEMENT_3D ( 'NONE', #10190, #60624, #36500 ) ;
#73515=VERTEX_POINT ( 'NONE', #2568 ) ;
#73518=CARTESIAN_POINT ( 'NONE',  ( -18.51436573157338117, 1511.187213306747708, 237.1421867457408723 ) ) ;
#73522=CARTESIAN_POINT ( 'NONE',  ( 32.86802468386284914, 1523.382868172864164, 201.0396662540042030 ) ) ;
#73525=DIRECTION ( 'NONE',  ( 0.4090087482554383147, -0.000000000000000000, 0.9125304618753937724 ) ) ;
#73537=ORIENTED_EDGE ( 'NONE', *, *, #64472, .F. ) ;
#73540=ADVANCED_FACE ( 'NONE', ( #77047 ), #45116, .T. ) ;
#73542=DIRECTION ( 'NONE',  ( 0.000000000000000000, 0.000000000000000000, 1.000000000000000000 ) ) ;
#73548=EDGE_CURVE ( 'NONE', #83547, #100304, #61615, .T. ) ;
#73570=EDGE_CURVE ( 'NONE', #17762, #100644, #89496, .T. ) ;
#73580=CARTESIAN_POINT ( 'NONE',  ( -30.87201549882227525, 1524.816548299036867, 221.7489384518832196 ) ) ;
#73583=CARTESIAN_POINT ( 'NONE',  ( 32.06267705388252409, 1524.739563915922645, 216.1098277237242655 ) ) ;
#73596=CARTESIAN_POINT ( 'NONE',  ( 17.42134197181193045, 1525.253996226949084, 237.1661559799196652 ) ) ;
#73611=CARTESIAN_POINT ( 'NONE',  ( 0.000000000000000000, 1512.187213306747481, 209.1218459616979999 ) ) ;
#73615=( BOUNDED_SURFACE ( )  B_SPLINE_SURFACE ( 3, 2, ( 
 ( #10058, #103563, #105233 ),
 ( #44231, #35823, #10624 ),
 ( #44791, #36363, #78943 ),
 ( #78375, #2251, #70555 ),
 ( #104673, #68897, #62151 ),
 ( #62721, #19555, #53761 ),
 ( #17323, #51517, #94606 ),
 ( #8950, #34706, #102999 ),
 ( #26296, #86212, #9505 ),
 ( #69446, #63261, #4961 ),
 ( #22286, #21738, #55940 ),
 ( #106328, #99009, #37473 ),
 ( #13898, #11720, #45892 ),
 ( #3349, #30716, #48085 ) ),
 .UNSPECIFIED., .F., .F., .F. ) 
 B_SPLINE_SURFACE_WITH_KNOTS ( ( 4, 2, 2, 2, 2, 2, 4 ),
 ( 3, 3 ),
 ( 0.000000000000000000, 0.0009440840677144979451, 0.001416126101571746863, 0.001888168135428995890, 0.002360210169286244917, 0.002832252203143493727, 0.003776336270857991780 ),
 ( 0.000000000000000000, 1.000000000000000000 ),
 .UNSPECIFIED. ) 
 GEOMETRIC_REPRESENTATION_ITEM ( )  RATIONAL_B_SPLINE_SURFACE ( (
 ( 1.000000000000000000, 0.8070209408750077529, 1.000000000000000000),
 ( 1.000000000000000000, 0.8215603905271136043, 1.000000000000000000),
 ( 1.000000000000000000, 0.8340988699078115687, 1.000000000000000000),
 ( 1.000000000000000000, 0.8516751610450099541, 1.000000000000000000),
 ( 1.000000000000000000, 0.8573697395149780798, 1.000000000000000000),
 ( 1.000000000000000000, 0.8683586635666556974, 1.000000000000000000),
 ( 1.000000000000000000, 0.8736518481708377415, 1.000000000000000000),
 ( 1.000000000000000000, 0.8840377753030403962, 1.000000000000000000),
 ( 1.000000000000000000, 0.8891294171309215288, 1.000000000000000000),
 ( 1.000000000000000000, 0.8992456600571828718, 1.000000000000000000),
 ( 1.000000000000000000, 0.9042785869255108855, 1.000000000000000000),
 ( 1.000000000000000000, 0.9189749222834227016, 1.000000000000000000),
 ( 1.000000000000000000, 0.9283978182351991792, 1.000000000000000000),
 ( 1.000000000000000000, 0.9376006582765968878, 1.000000000000000000) ) ) 
 REPRESENTATION_ITEM ( '' )  SURFACE ( )  );
#73625=ORIENTED_EDGE ( 'NONE', *, *, #76848, .T. ) ;
#73653=AXIS2_PLACEMENT_3D ( 'NONE', #42573, #110324, #59950 ) ;
#73682=CARTESIAN_POINT ( 'NONE',  ( 31.97743984922262683, 1525.878013734321485, 220.1676294520832755 ) ) ;
#73683=VERTEX_POINT ( 'NONE', #3363 ) ;
#73718=EDGE_CURVE ( 'NONE', #35166, #49199, #21507, .T. ) ;
#73731=CARTESIAN_POINT ( 'NONE',  ( -31.23437356469455040, 1512.187213306747481, 195.3468678195118287 ) ) ;
#73739=CARTESIAN_POINT ( 'NONE',  ( 32.40058737600722338, 1524.130440953581001, 201.3079925683071849 ) ) ;
#73748=CYLINDRICAL_SURFACE ( 'NONE', #3621, 0.9999999999999976685 ) ;
#73749=CIRCLE ( 'NONE', #2219, 0.9999999999999953371 ) ;
#73756=VERTEX_POINT ( 'NONE', #10638 ) ;
#73757=FACE_OUTER_BOUND ( 'NONE', #62083, .T. ) ;
#73759=ORIENTED_EDGE ( 'NONE', *, *, #81678, .T. ) ;
#73783=CARTESIAN_POINT ( 'NONE',  ( -8.840620885073990465, 1512.187213306747481, 223.8289249455316394 ) ) ;
#73813=ADVANCED_FACE ( 'NONE', ( #62738 ), #68913, .F. ) ;
#73829=PLANE ( 'NONE',  #58673 ) ;
#73846=VERTEX_POINT ( 'NONE', #80597 ) ;
#73851=CARTESIAN_POINT ( 'NONE',  ( -17.83486663330526767, 1523.678648413191695, 180.3677388339002334 ) ) ;
#73854=CARTESIAN_POINT ( 'NONE',  ( 31.23437356469446868, 1512.187213306747481, 222.8968241038843701 ) ) ;
#73864=DIRECTION ( 'NONE',  ( 0.000000000000000000, 1.000000000000000000, 0.000000000000000000 ) ) ;
#73873=DIRECTION ( 'NONE',  ( -0.000000000000000000, -1.000000000000000000, -0.000000000000000000 ) ) ;
#73886=DIRECTION ( 'NONE',  ( 0.9786619618251657382, 0.000000000000000000, -0.2054769195713184449 ) ) ;
#73891=EDGE_CURVE ( 'NONE', #10257, #54321, #17640, .T. ) ;
#73896=DIRECTION ( 'NONE',  ( -0.000000000000000000, -1.000000000000000000, -0.000000000000000000 ) ) ;
#73918=CARTESIAN_POINT ( 'NONE',  ( 2.686147501205802701, 1526.329757971589515, 176.3936480404081237 ) ) ;
#73927=CARTESIAN_POINT ( 'NONE',  ( 30.15498091547360460, 1525.730671948510917, 196.9950492442363270 ) ) ;
#73938=( BOUNDED_SURFACE ( )  B_SPLINE_SURFACE ( 3, 2, ( 
 ( #5783, #99808, #98721 ),
 ( #21981, #91435, #14711 ),
 ( #13590, #4138, #56173 ),
 ( #80283, #64048, #97631 ),
 ( #55099, #89225, #46698 ),
 ( #29862, #21438, #32070 ) ),
 .UNSPECIFIED., .F., .F., .F. ) 
 B_SPLINE_SURFACE_WITH_KNOTS ( ( 4, 2, 4 ),
 ( 3, 3 ),
 ( -4.293440603042597559E-17, 0.001312027981647320837, 0.002624055963294684608 ),
 ( 0.000000000000000000, 1.000000000000000000 ),
 .UNSPECIFIED. ) 
 GEOMETRIC_REPRESENTATION_ITEM ( )  RATIONAL_B_SPLINE_SURFACE ( (
 ( 1.000000000000000000, 0.9376006582765885611, 1.000000000000000000),
 ( 1.000000000000000000, 0.9569320108022199012, 1.000000000000000000),
 ( 1.000000000000000000, 0.9725743441619376650, 1.000000000000000000),
 ( 1.000000000000000000, 0.9942095667135113501, 1.000000000000000000),
 ( 1.000000000000000000, 1.000043666450747493, 1.000000000000000000),
 ( 1.000000000000000000, 1.000000000000000000, 1.000000000000000000) ) ) 
 REPRESENTATION_ITEM ( '' )  SURFACE ( )  );
#73940=VERTEX_POINT ( 'NONE', #21196 ) ;
#73945=ADVANCED_FACE ( 'NONE', ( #99576 ), #13915, .F. ) ;
#73953=CARTESIAN_POINT ( 'NONE',  ( -22.08327125186962192, 1523.604703353109699, 184.4267662568474009 ) ) ;
#73959=DIRECTION ( 'NONE',  ( 0.000000000000000000, 0.000000000000000000, -1.000000000000000000 ) ) ;
#73961=CARTESIAN_POINT ( 'NONE',  ( -0.5770119038902318254, 1525.581535527370534, 174.8524476110295325 ) ) ;
#73962=CARTESIAN_POINT ( 'NONE',  ( 9.373950541344202136, 1512.187213306747481, 228.8708405320806492 ) ) ;
#73971=ORIENTED_EDGE ( 'NONE', *, *, #39743, .T. ) ;
#73982=CARTESIAN_POINT ( 'NONE',  ( -21.96543842109194600, 1523.313115944345327, 182.9844783913652861 ) ) ;
#73984=CARTESIAN_POINT ( 'NONE',  ( -19.37774363895776730, 1525.878013734318984, 236.8539400710568259 ) ) ;
#73987=CARTESIAN_POINT ( 'NONE',  ( 16.56942828594079842, 1526.189892541618974, 182.6454327952257302 ) ) ;
#73999=LINE ( 'NONE', #66171, #85911 ) ;
#74013=CARTESIAN_POINT ( 'NONE',  ( 2.640434834157764143, 1526.748660780343471, 176.9315852594520777 ) ) ;
#74028=DIRECTION ( 'NONE',  ( 3.469446951953611033E-14, 0.000000000000000000, 1.000000000000000000 ) ) ;
#74050=CYLINDRICAL_SURFACE ( 'NONE', #18133, 0.9999999999999976685 ) ;
#74053=ORIENTED_EDGE ( 'NONE', *, *, #82556, .T. ) ;
#74065=CARTESIAN_POINT ( 'NONE',  ( 33.93019615848945847, 1512.187213306747481, 197.6607374645996060 ) ) ;
#74074=CARTESIAN_POINT ( 'NONE',  ( 0.000000000000000000, 1526.382868172863937, 209.1218459616979999 ) ) ;
#74087=CARTESIAN_POINT ( 'NONE',  ( -17.24701964721560543, 1523.844782250842172, 237.3932573007202222 ) ) ;
#74116=AXIS2_PLACEMENT_3D ( 'NONE', #86294, #93575, #16850 ) ;
#74126=AXIS2_PLACEMENT_3D ( 'NONE', #30878, #89688, #47700 ) ;
#74130=CARTESIAN_POINT ( 'NONE',  ( -19.34601893677229967, 1526.333389948038530, 185.2009018889136200 ) ) ;
#74143=CARTESIAN_POINT ( 'NONE',  ( 17.72016947435118084, 1524.201816949777140, 237.7555919081156617 ) ) ;
#74151=CIRCLE ( 'NONE', #31444, 1.000000000000000888 ) ;
#74172=FILL_AREA_STYLE_COLOUR ( '', #43160 ) ;
#74187=EDGE_CURVE ( 'NONE', #32820, #39464, #65747, .T. ) ;
#74218=DIRECTION ( 'NONE',  ( 1.000000000000000000, -0.000000000000000000, 1.224646799147353207E-16 ) ) ;
#74225=CARTESIAN_POINT ( 'NONE',  ( 30.31940284292408805, 1523.382868172864164, 195.7503880523414352 ) ) ;
#74226=LINE ( 'NONE', #83155, #19923 ) ;
#74233=CARTESIAN_POINT ( 'NONE',  ( -32.38845791999504797, 1523.382868172864164, 202.1182848005516348 ) ) ;
#74234=CARTESIAN_POINT ( 'NONE',  ( 32.99911596133151193, 1524.244163922423695, 222.0809728102182135 ) ) ;
#74252=AXIS2_PLACEMENT_3D ( 'NONE', #42771, #103782, #33252 ) ;
#74264=DIRECTION ( 'NONE',  ( -0.000000000000000000, -1.000000000000000000, -0.000000000000000000 ) ) ;
#74275=ORIENTED_EDGE ( 'NONE', *, *, #54969, .T. ) ;
#74277=DIRECTION ( 'NONE',  ( 0.000000000000000000, 1.000000000000000000, 0.000000000000000000 ) ) ;
#74289=CARTESIAN_POINT ( 'NONE',  ( 33.72300830903895275, 1524.397344074319108, 198.6568221122816453 ) ) ;
#74301=EDGE_CURVE ( 'NONE', #39623, #47286, #86389, .T. ) ;
#74312=ORIENTED_EDGE ( 'NONE', *, *, #41906, .F. ) ;
#74314=EDGE_CURVE ( 'NONE', #95189, #43597, #100262, .T. ) ;
#74320=EDGE_CURVE ( 'NONE', #30404, #29269, #17935, .T. ) ;
#74326=DIRECTION ( 'NONE',  ( 0.2054769195713296304, 0.000000000000000000, 0.9786619618251631847 ) ) ;
#74328=TOROIDAL_SURFACE ( 'NONE', #8112, 1.000000000000000000, 1.000000000000000000 ) ;
#74333=ORIENTED_EDGE ( 'NONE', *, *, #32256, .T. ) ;
#74334=ORIENTED_EDGE ( 'NONE', *, *, #91748, .T. ) ;
#74349=ORIENTED_EDGE ( 'NONE', *, *, #93178, .T. ) ;
#74354=DIRECTION ( 'NONE',  ( -0.6709778558543728622, 0.000000000000000000, 0.7414773880254666993 ) ) ;
#74361=CARTESIAN_POINT ( 'NONE',  ( 30.61443310237131499, 1523.382868172863937, 221.8243310972799236 ) ) ;
#74371=CIRCLE ( 'NONE', #29659, 0.9999999999999015232 ) ;
#74384=ORIENTED_EDGE ( 'NONE', *, *, #7293, .F. ) ;
#74391=CARTESIAN_POINT ( 'NONE',  ( 0.000000000000000000, 1512.187213306747481, 209.1218459616979999 ) ) ;
#74394=AXIS2_PLACEMENT_3D ( 'NONE', #59646, #5656, #31389 ) ;
#74414=DIRECTION ( 'NONE',  ( 0.000000000000000000, 0.000000000000000000, 1.000000000000000000 ) ) ;
#74418=FACE_OUTER_BOUND ( 'NONE', #23605, .T. ) ;
#74428=EDGE_CURVE ( 'NONE', #65751, #81551, #28766, .T. ) ;
#74439=CARTESIAN_POINT ( 'NONE',  ( 29.00779973304118897, 1526.382868172864164, 200.9494832830835378 ) ) ;
#74476=VERTEX_POINT ( 'NONE', #47024 ) ;
#74477=CARTESIAN_POINT ( 'NONE',  ( 2.470168521978398424, 1523.382868172864164, 175.3649660270905315 ) ) ;
#74480=ORIENTED_EDGE ( 'NONE', *, *, #57642, .T. ) ;
#74510=CARTESIAN_POINT ( 'NONE',  ( 17.29393938232459860, 1523.621879633029039, 180.8572348224458608 ) ) ;
#74518=CARTESIAN_POINT ( 'NONE',  ( 0.000000000000000000, 1523.382868172864164, 209.1218459616979999 ) ) ;
#74520=DIRECTION ( 'NONE',  ( -0.2113515706023144647, 0.000000000000000000, 0.9774101051267757301 ) ) ;
#74525=VERTEX_POINT ( 'NONE', #6653 ) ;
#74532=CARTESIAN_POINT ( 'NONE',  ( -17.19739463999671614, 1525.960063244516959, 181.9833109756550300 ) ) ;
#74545=CARTESIAN_POINT ( 'NONE',  ( 16.50400130224750583, 1525.907212628473644, 181.9890130758377040 ) ) ;
#74569=EDGE_LOOP ( 'NONE', ( #108917, #8721, #24446, #29308 ) ) ;
#74572=CYLINDRICAL_SURFACE ( 'NONE', #65296, 0.9999999999999970024 ) ;
#74585=FACE_OUTER_BOUND ( 'NONE', #69376, .T. ) ;
#74589=VERTEX_POINT ( 'NONE', #43030 ) ;
#74611=ORIENTED_EDGE ( 'NONE', *, *, #41795, .F. ) ;
#74614=DIRECTION ( 'NONE',  ( 0.000000000000000000, 0.000000000000000000, -1.000000000000000000 ) ) ;
#74620=CARTESIAN_POINT ( 'NONE',  ( -21.41029105011889300, 1526.329757971582922, 184.2230555347968561 ) ) ;
#74635=CARTESIAN_POINT ( 'NONE',  ( -1.488474718482915460, 1526.348417187222594, 178.3303222095513831 ) ) ;
#74638=CARTESIAN_POINT ( 'NONE',  ( -2.470168521978398868, 1501.977400791986611, 242.8787258963054683 ) ) ;
#74662=EDGE_CURVE ( 'NONE', #67570, #90273, #102026, .T. ) ;
#74680=CARTESIAN_POINT ( 'NONE',  ( 32.21733215212998402, 1523.844782250843537, 216.7883898251401149 ) ) ;
#74683=ADVANCED_FACE ( 'NONE', ( #73757 ), #47988, .T. ) ;
#74689=ADVANCED_FACE ( 'NONE', ( #90526 ), #107880, .F. ) ;
#74695=CARTESIAN_POINT ( 'NONE',  ( -29.33431687954604783, 1526.382868172863937, 201.1003846321129629 ) ) ;
#74705=ORIENTED_EDGE ( 'NONE', *, *, #13794, .T. ) ;
#74713=CARTESIAN_POINT ( 'NONE',  ( 22.08622291482331335, 1512.187213306747481, 184.4183880513174927 ) ) ;
#74723=ORIENTED_EDGE ( 'NONE', *, *, #37056, .T. ) ;
#74736=ORIENTED_EDGE ( 'NONE', *, *, #104329, .T. ) ;
#74746=AXIS2_PLACEMENT_3D ( 'NONE', #55669, #64621, #13064 ) ;
#74763=ORIENTED_EDGE ( 'NONE', *, *, #92242, .T. ) ;
#74767=DIRECTION ( 'NONE',  ( 0.000000000000000000, 0.000000000000000000, 1.000000000000000000 ) ) ;
#74781=EDGE_CURVE ( 'NONE', #39868, #55319, #23382, .T. ) ;
#74787=EDGE_CURVE ( 'NONE', #49270, #72812, #90853, .T. ) ;
#74793=CARTESIAN_POINT ( 'NONE',  ( 20.49599333844836124, 1525.960063244517187, 184.3798832129035645 ) ) ;
#74798=EDGE_CURVE ( 'NONE', #90799, #70084, #41236, .T. ) ;
#74825=CARTESIAN_POINT ( 'NONE',  ( -16.73628186595857059, 1526.382868172863937, 184.0591879540917546 ) ) ;
#74846=CARTESIAN_POINT ( 'NONE',  ( 1.191524307911316916, 1526.382868172864164, 239.2353018730791518 ) ) ;
#74859=CARTESIAN_POINT ( 'NONE',  ( -20.49599333844893678, 1525.960063244516959, 184.3798832129038203 ) ) ;
#74874=ORIENTED_EDGE ( 'NONE', *, *, #72677, .T. ) ;
#74875=ORIENTED_EDGE ( 'NONE', *, *, #324, .T. ) ;
#74877=CARTESIAN_POINT ( 'NONE',  ( -28.97303002314116682, 1526.186458717541882, 220.8123550170195699 ) ) ;
#74879=EDGE_CURVE ( 'NONE', #98801, #100321, #57403, .T. ) ;
#74882=B_SPLINE_CURVE_WITH_KNOTS ( 'NONE', 3,
 ( #34851, #69040, #52230, #28108 ),
 .UNSPECIFIED., .F., .F.,
 ( 4, 4 ),
 ( 0.000000000000000000, 0.0002960034161023843515 ),
 .UNSPECIFIED. ) ;
#74894=CARTESIAN_POINT ( 'NONE',  ( 21.53981368633935745, 1523.542365884049104, 234.3096115065364984 ) ) ;
#74915=( BOUNDED_SURFACE ( )  B_SPLINE_SURFACE ( 3, 2, ( 
 ( #12951, #47132, #82918 ),
 ( #38707, #4573, #90767 ),
 ( #14047, #82378, #5678 ),
 ( #73984, #65590, #32527 ),
 ( #6755, #49334, #59400 ),
 ( #75095, #66699, #16784 ),
 ( #100278, #33061, #57750 ),
 ( #101344, #84019, #102463 ),
 ( #43137, #67249, #58832 ),
 ( #25753, #108674, #40915 ) ),
 .UNSPECIFIED., .F., .F., .F. ) 
 B_SPLINE_SURFACE_WITH_KNOTS ( ( 4, 2, 2, 2, 4 ),
 ( 3, 3 ),
 ( 1.570796326794896558, 1.963495408493620697, 2.356194490192344837, 2.748893571891068976, 3.141592653589793116 ),
 ( 0.000000000000000000, 1.000000000000000000 ),
 .UNSPECIFIED. ) 
 GEOMETRIC_REPRESENTATION_ITEM ( )  RATIONAL_B_SPLINE_SURFACE ( (
 ( 1.000000000000000000, 0.7071067811865904273, 1.000000000000000000),
 ( 1.000000000000000000, 0.7166207884824742358, 1.000000000000000000),
 ( 1.000000000000000000, 0.7259222650903540686, 1.000000000000000000),
 ( 1.000000000000000000, 0.7428408967933899376, 1.000000000000000000),
 ( 1.000000000000000000, 0.7504512394528214392, 1.000000000000000000),
 ( 1.000000000000000000, 0.7630177051946679390, 1.000000000000000000),
 ( 1.000000000000000000, 0.7679730451967922145, 1.000000000000000000),
 ( 1.000000000000000000, 0.7746454561802565975, 1.000000000000000000),
 ( 1.000000000000000000, 0.7763684247031245045, 1.000000000000000000),
 ( 1.000000000000000000, 0.7763623250684338339, 1.000000000000000000) ) ) 
 REPRESENTATION_ITEM ( '' )  SURFACE ( )  );
#74941=CARTESIAN_POINT ( 'NONE',  ( 18.40343465886133600, 1525.402221411349956, 179.8532301504589839 ) ) ;
#74961=DIRECTION ( 'NONE',  ( 0.4090087482554252696, -0.000000000000000000, -0.9125304618753996566 ) ) ;
#74969=AXIS2_PLACEMENT_3D ( 'NONE', #84011, #7312, #101336 ) ;
#74979=DIRECTION ( 'NONE',  ( -0.000000000000000000, -1.000000000000000000, -0.000000000000000000 ) ) ;
#75003=DIRECTION ( 'NONE',  ( 0.000000000000000000, 0.000000000000000000, 1.000000000000000000 ) ) ;
#75015=ORIENTED_EDGE ( 'NONE', *, *, #100368, .F. ) ;
#75042=VECTOR ( 'NONE', #73525, 1000.000000000000114 ) ;
#75044=CARTESIAN_POINT ( 'NONE',  ( 32.38114538885250226, 1523.604703353109699, 202.1233279672528624 ) ) ;
#75050=FACE_OUTER_BOUND ( 'NONE', #18220, .T. ) ;
#75055=EDGE_CURVE ( 'NONE', #73175, #107075, #58992, .T. ) ;
#75059=CARTESIAN_POINT ( 'NONE',  ( -29.67167576298847109, 1526.344110814222859, 201.2571182723721961 ) ) ;
#75069=ADVANCED_FACE ( 'NONE', ( #29935 ), #24190, .F. ) ;
#75071=CARTESIAN_POINT ( 'NONE',  ( -2.582675909239641854, 1526.178928173327677, 175.9008252398585626 ) ) ;
#75076=ORIENTED_EDGE ( 'NONE', *, *, #31936, .T. ) ;
#75078=CARTESIAN_POINT ( 'NONE',  ( 3.347801439296141268, 1512.187213306747481, 242.0893193391992497 ) ) ;
#75086=CARTESIAN_POINT ( 'NONE',  ( -16.50400130224786466, 1525.907212628473644, 181.9890130758379030 ) ) ;
#75092=CARTESIAN_POINT ( 'NONE',  ( 32.38845791999495560, 1523.382868172864164, 202.1182848005512085 ) ) ;
#75094=ADVANCED_FACE ( 'NONE', ( #63585 ), #56810, .T. ) ;
#75095=CARTESIAN_POINT ( 'NONE',  ( -20.17436656406251672, 1524.841055067849766, 237.7389007707605515 ) ) ;
#75108=CIRCLE ( 'NONE', #41118, 2.000000000000001776 ) ;
#75120=DIRECTION ( 'NONE',  ( 0.000000000000000000, 0.000000000000000000, 1.000000000000000000 ) ) ;
#75123=ORIENTED_EDGE ( 'NONE', *, *, #1753, .F. ) ;
#75132=CIRCLE ( 'NONE', #107326, 1.000000000000000888 ) ;
#75144=ORIENTED_EDGE ( 'NONE', *, *, #56744, .T. ) ;
#75178=CARTESIAN_POINT ( 'NONE',  ( 31.23437356469435144, 1512.187213306747481, 195.3468678195113739 ) ) ;
#75209=AXIS2_PLACEMENT_3D ( 'NONE', #38516, #19508, #30109 ) ;
#75212=ADVANCED_FACE ( 'NONE', ( #91915 ), #57164, .T. ) ;
#75220=DIRECTION ( 'NONE',  ( 0.000000000000000000, -1.000000000000000000, 0.000000000000000000 ) ) ;
#75224=CARTESIAN_POINT ( 'NONE',  ( 17.17241001986483795, 1511.187213306747708, 179.6185504016043240 ) ) ;
#75226=CARTESIAN_POINT ( 'NONE',  ( -30.98826378581289021, 1524.599984580802129, 221.8039704955955642 ) ) ;
#75230=LINE ( 'NONE', #51677, #37588 ) ;
#75245=CARTESIAN_POINT ( 'NONE',  ( 17.36692773919801169, 1525.425665131968344, 237.0071470213579232 ) ) ;
#75266=DIRECTION ( 'NONE',  ( -0.000000000000000000, -1.000000000000000000, -0.000000000000000000 ) ) ;
#75278=ORIENTED_EDGE ( 'NONE', *, *, #65365, .F. ) ;
#75288=ORIENTED_EDGE ( 'NONE', *, *, #72062, .T. ) ;
#75293=ORIENTED_EDGE ( 'NONE', *, *, #41460, .T. ) ;
#75295=ORIENTED_EDGE ( 'NONE', *, *, #95175, .T. ) ;
#75298=EDGE_CURVE ( 'NONE', #40736, #23656, #36968, .T. ) ;
#75318=AXIS2_PLACEMENT_3D ( 'NONE', #65668, #38788, #65119 ) ;
#75324=DIRECTION ( 'NONE',  ( 0.000000000000000000, 0.000000000000000000, 1.000000000000000000 ) ) ;
#75325=AXIS2_PLACEMENT_3D ( 'NONE', #40613, #84804, #92660 ) ;
#75344=TOROIDAL_SURFACE ( 'NONE', #9231, 1.000000000000000000, 1.000000000000000000 ) ;
#75351=CARTESIAN_POINT ( 'NONE',  ( 18.98249322451690446, 1526.382868172864164, 185.2725498412042953 ) ) ;
#75359=CARTESIAN_POINT ( 'NONE',  ( -22.03465957474533354, 1512.187213306747481, 235.4136513321633117 ) ) ;
#75361=CARTESIAN_POINT ( 'NONE',  ( -16.66231036550740541, 1523.604703353109699, 180.4882076302515372 ) ) ;
#75362=CARTESIAN_POINT ( 'NONE',  ( 16.49514809540576366, 1525.343727714918259, 181.2134271599560691 ) ) ;
#75363=AXIS2_PLACEMENT_3D ( 'NONE', #69955, #103510, #1087 ) ;
#75375=CARTESIAN_POINT ( 'NONE',  ( -18.98249322453838417, 1526.382868172864164, 232.9711420821614070 ) ) ;
#75384=CARTESIAN_POINT ( 'NONE',  ( -2.686147501205254695, 1526.329757971589288, 241.8500438829907466 ) ) ;
#75401=CARTESIAN_POINT ( 'NONE',  ( 1.961418762360136681, 1526.143142182266047, 240.4212258933422675 ) ) ;
#75403=DIRECTION ( 'NONE',  ( 0.000000000000000000, 1.000000000000000000, 0.000000000000000000 ) ) ;
#75415=EDGE_CURVE ( 'NONE', #10931, #23627, #26764, .T. ) ;
#75425=CIRCLE ( 'NONE', #50331, 2.000000000000001776 ) ;
#75430=CARTESIAN_POINT ( 'NONE',  ( -16.66936639845670598, 1523.382868172864164, 180.4828114240741570 ) ) ;
#75434=DIRECTION ( 'NONE',  ( -0.5030436214085368674, 0.000000000000000000, 0.8642610224695920218 ) ) ;
#75435=EDGE_CURVE ( 'NONE', #13274, #42640, #100050, .T. ) ;
#75446=ORIENTED_EDGE ( 'NONE', *, *, #89780, .F. ) ;
#75449=EDGE_CURVE ( 'NONE', #72812, #74476, #103658, .T. ) ;
#75467=EDGE_LOOP ( 'NONE', ( #58730, #4740, #97259, #97390 ) ) ;
#75472=CARTESIAN_POINT ( 'NONE',  ( -22.69876404240057965, 1501.977400791986611, 236.8953202675781426 ) ) ;
#75474=FACE_OUTER_BOUND ( 'NONE', #25396, .T. ) ;
#75483=DIRECTION ( 'NONE',  ( 0.9510565162951545304, 0.000000000000000000, 0.3090169943749447312 ) ) ;
#75501=DIRECTION ( 'NONE',  ( 0.000000000000000000, 0.000000000000000000, 1.000000000000000000 ) ) ;
#75515=CARTESIAN_POINT ( 'NONE',  ( -29.00779973304142345, 1526.382868172863937, 200.9494832830838789 ) ) ;
#75537=EDGE_CURVE ( 'NONE', #85718, #95777, #67957, .T. ) ;
#75546=CARTESIAN_POINT ( 'NONE',  ( -2.444993193446221014, 1524.972383263452912, 175.9711954026445824 ) ) ;
#75558=DIRECTION ( 'NONE',  ( 0.000000000000000000, 0.000000000000000000, -1.000000000000000000 ) ) ;
#75571=ORIENTED_EDGE ( 'NONE', *, *, #20753, .F. ) ;
#75575=( BOUNDED_SURFACE ( )  B_SPLINE_SURFACE ( 3, 2, ( 
 ( #52322, #94849, #103222 ),
 ( #18125, #86445, #86996 ),
 ( #9735, #93179, #61290 ),
 ( #43901, #16448, #59057 ),
 ( #110540, #44461, #33827 ),
 ( #68019, #102128, #25407 ),
 ( #52868, #10284, #34390 ),
 ( #59600, #93716, #16993 ),
 ( #51193, #85323, #102663 ),
 ( #8618, #68565, #60158 ) ),
 .UNSPECIFIED., .F., .F., .T. ) 
 B_SPLINE_SURFACE_WITH_KNOTS ( ( 4, 2, 2, 2, 4 ),
 ( 3, 3 ),
 ( 0.000000000000000000, 0.3926990816987241395, 0.7853981633974482790, 1.178097245096172418, 1.570796326794896558 ),
 ( 0.000000000000000000, 1.000000000000000000 ),
 .UNSPECIFIED. ) 
 GEOMETRIC_REPRESENTATION_ITEM ( )  RATIONAL_B_SPLINE_SURFACE ( (
 ( 1.000000000000000000, 0.7763623250684315025, 1.000000000000000000),
 ( 1.000000000000000000, 0.7763684247040171238, 1.000000000000000000),
 ( 1.000000000000000000, 0.7746454561790633297, 1.000000000000000000),
 ( 1.000000000000000000, 0.7679730451979892569, 1.000000000000000000),
 ( 1.000000000000000000, 0.7630177051949805778, 1.000000000000000000),
 ( 1.000000000000000000, 0.7504512394525143515, 1.000000000000000000),
 ( 1.000000000000000000, 0.7428408967930927309, 1.000000000000000000),
 ( 1.000000000000000000, 0.7259222650906490548, 1.000000000000000000),
 ( 1.000000000000000000, 0.7166207884822589635, 1.000000000000000000),
 ( 1.000000000000000000, 0.7071067811865853203, 1.000000000000000000) ) ) 
 REPRESENTATION_ITEM ( '' )  SURFACE ( )  );
#75581=ORIENTED_EDGE ( 'NONE', *, *, #14485, .F. ) ;
#75601=DIRECTION ( 'NONE',  ( -3.552713678800501718E-15, 0.000000000000000000, -1.000000000000000000 ) ) ;
#75626=CARTESIAN_POINT ( 'NONE',  ( 31.23437356469435144, 1518.913060387330006, 195.3468678195113739 ) ) ;
#75628=CARTESIAN_POINT ( 'NONE',  ( 1.679554717346656512, 1526.335487865669393, 178.4817626271500899 ) ) ;
#75634=CARTESIAN_POINT ( 'NONE',  ( -16.97880994393915799, 1525.055427061254477, 181.2503854651100710 ) ) ;
#75635=FACE_OUTER_BOUND ( 'NONE', #65381, .T. ) ;
#75637=CARTESIAN_POINT ( 'NONE',  ( -16.69343462643249509, 1526.373507135059526, 183.7014874209610866 ) ) ;
#75649=CARTESIAN_POINT ( 'NONE',  ( -1.679554717346650072, 1526.335487865669393, 239.7619292962459383 ) ) ;
#75656=DIRECTION ( 'NONE',  ( 0.000000000000000000, 1.000000000000000000, 0.000000000000000000 ) ) ;
#75677=EDGE_CURVE ( 'NONE', #32377, #49931, #94701, .T. ) ;
#75694=DIRECTION ( 'NONE',  ( 0.000000000000000000, 0.000000000000000000, -1.000000000000000000 ) ) ;
#75698=CARTESIAN_POINT ( 'NONE',  ( 29.30029655192931770, 1525.907212628473872, 221.3719603026171114 ) ) ;
#75721=DIRECTION ( 'NONE',  ( 2.664535259100376091E-15, 0.000000000000000000, -1.000000000000000000 ) ) ;
#75722=EDGE_CURVE ( 'NONE', #39623, #65697, #17782, .T. ) ;
#75729=EDGE_CURVE ( 'NONE', #28004, #67358, #41361, .T. ) ;
#75732=VERTEX_POINT ( 'NONE', #51681 ) ;
#75739=CARTESIAN_POINT ( 'NONE',  ( 16.66936639845630097, 1518.913060387330006, 180.4828114240739296 ) ) ;
#75747=CARTESIAN_POINT ( 'NONE',  ( -32.23393008293637507, 1523.462669333491931, 216.8400319009761006 ) ) ;
#75761=CARTESIAN_POINT ( 'NONE',  ( 20.87480701074298750, 1525.712835404586031, 234.0672321669388509 ) ) ;
#75770=CARTESIAN_POINT ( 'NONE',  ( -16.49514809540558247, 1525.343727714918259, 237.0302647634398170 ) ) ;
#75778=CARTESIAN_POINT ( 'NONE',  ( 17.62880125161999345, 1524.547395018738143, 180.6298994264734858 ) ) ;
#75787=DIRECTION ( 'NONE',  ( -0.000000000000000000, -1.000000000000000000, -0.000000000000000000 ) ) ;
#75797=ORIENTED_EDGE ( 'NONE', *, *, #98706, .T. ) ;
#75804=LINE ( 'NONE', #7487, #6950 ) ;
#75817=EDGE_LOOP ( 'NONE', ( #78394, #97723, #37525, #15889 ) ) ;
#75833=ORIENTED_EDGE ( 'NONE', *, *, #91235, .F. ) ;
#75835=ORIENTED_EDGE ( 'NONE', *, *, #70025, .T. ) ;
#75838=EDGE_CURVE ( 'NONE', #92224, #62492, #14281, .T. ) ;
#75846=CARTESIAN_POINT ( 'NONE',  ( -173.8335085727399871, 1526.382868172863937, 100.8557906292094373 ) ) ;
#75852=CARTESIAN_POINT ( 'NONE',  ( -21.44521871417750702, 1525.343710797494396, 233.4338460867892877 ) ) ;
#75864=CIRCLE ( 'NONE', #27584, 0.9999999999999135136 ) ;
#75874=( BOUNDED_SURFACE ( )  B_SPLINE_SURFACE ( 3, 2, ( 
 ( #21509, #47295, #20965 ),
 ( #64117, #48413, #71984 ),
 ( #90940, #90377, #107195 ),
 ( #81419, #63040, #12035 ) ),
 .UNSPECIFIED., .F., .F., .F. ) 
 B_SPLINE_SURFACE_WITH_KNOTS ( ( 4, 4 ),
 ( 3, 3 ),
 ( 0.000000000000000000, 0.0002960034161023842973 ),
 ( 0.000000000000000000, 1.000000000000000000 ),
 .UNSPECIFIED. ) 
 GEOMETRIC_REPRESENTATION_ITEM ( )  RATIONAL_B_SPLINE_SURFACE ( (
 ( 1.000000000000000000, 0.8072480644198088973, 1.000000000000000000),
 ( 1.000000000000000000, 0.8072480346917575433, 1.000000000000000000),
 ( 1.000000000000000000, 0.8071723757218559614, 1.000000000000000000),
 ( 1.000000000000000000, 0.8070209408749943192, 1.000000000000000000) ) ) 
 REPRESENTATION_ITEM ( '' )  SURFACE ( )  );
#75876=DIRECTION ( 'NONE',  ( 0.000000000000000000, 1.000000000000000000, 0.000000000000000000 ) ) ;
#75878=CARTESIAN_POINT ( 'NONE',  ( -17.16388877745089303, 1523.678648413191695, 179.6262614458747464 ) ) ;
#75885=CARTESIAN_POINT ( 'NONE',  ( -21.48648064083822362, 1524.477587234266139, 184.1567740173552465 ) ) ;
#75887=ORIENTED_EDGE ( 'NONE', *, *, #98052, .F. ) ;
#75901=VERTEX_POINT ( 'NONE', #12419 ) ;
#75904=ORIENTED_EDGE ( 'NONE', *, *, #99903, .T. ) ;
#75905=ORIENTED_EDGE ( 'NONE', *, *, #54202, .F. ) ;
#75921=ORIENTED_EDGE ( 'NONE', *, *, #105133, .F. ) ;
#75922=ORIENTED_EDGE ( 'NONE', *, *, #11350, .T. ) ;
#75928=CARTESIAN_POINT ( 'NONE',  ( 1.689251544526354731, 1526.344110814221267, 239.7716210576236904 ) ) ;
#75937=CARTESIAN_POINT ( 'NONE',  ( 2.038646110889675178, 1525.960063244516959, 241.1857569150893994 ) ) ;
#75950=ORIENTED_EDGE ( 'NONE', *, *, #90698, .F. ) ;
#75959=CARTESIAN_POINT ( 'NONE',  ( 30.01999388067563146, 1525.848198008145346, 197.1136717113790553 ) ) ;
#75960=VERTEX_POINT ( 'NONE', #37629 ) ;
#75978=CARTESIAN_POINT ( 'NONE',  ( -18.86688640473621703, 1512.187213306747481, 180.7825021045441076 ) ) ;
#75986=DIRECTION ( 'NONE',  ( 0.000000000000000000, 1.000000000000000000, 0.000000000000000000 ) ) ;
#75996=DIRECTION ( 'NONE',  ( 0.000000000000000000, 1.000000000000000000, 0.000000000000000000 ) ) ;
#76011=CARTESIAN_POINT ( 'NONE',  ( 28.44698416550310327, 1526.373507135059072, 219.8751933407330341 ) ) ;
#76019=EDGE_CURVE ( 'NONE', #99467, #107075, #91335, .T. ) ;
#76022=CIRCLE ( 'NONE', #20609, 1.000000000000000000 ) ;
#76029=ORIENTED_EDGE ( 'NONE', *, *, #6253, .F. ) ;
#76038=EDGE_CURVE ( 'NONE', #22289, #16677, #32122, .T. ) ;
#76043=DIRECTION ( 'NONE',  ( -0.000000000000000000, -1.000000000000000000, -0.000000000000000000 ) ) ;
#76092=LINE ( 'NONE', #42477, #4255 ) ;
#76106=CIRCLE ( 'NONE', #36708, 2.000000000000001776 ) ;
#76127=CARTESIAN_POINT ( 'NONE',  ( 2.311632204762886111, 1525.506926151471362, 241.8052033139069010 ) ) ;
#76143=CARTESIAN_POINT ( 'NONE',  ( -29.74444329484511940, 1526.348417187221685, 201.0223654199412806 ) ) ;
#76152=CARTESIAN_POINT ( 'NONE',  ( -0.4260839224734190300, 1523.429859730332510, 173.4147438076392405 ) ) ;
#76153=EDGE_CURVE ( 'NONE', #39456, #911, #48109, .T. ) ;
#76158=CARTESIAN_POINT ( 'NONE',  ( 0.000000000000000000, 1512.187213306747481, 209.1218459616979999 ) ) ;
#76168=CARTESIAN_POINT ( 'NONE',  ( 2.472529913803013013, 1523.678648413191695, 175.3762130535718313 ) ) ;
#76185=CARTESIAN_POINT ( 'NONE',  ( -1.436439550961307932, 1526.373507135059526, 239.4995027077839325 ) ) ;
#76188=CIRCLE ( 'NONE', #60063, 2.000000000000001776 ) ;
#76189=CARTESIAN_POINT ( 'NONE',  ( -16.66231036550682987, 1523.604703353109699, 237.7554842931448036 ) ) ;
#76216=( BOUNDED_CURVE ( )  B_SPLINE_CURVE ( 3, ( #61145, #9041, #44318, #26955 ),
 .UNSPECIFIED., .F., .T. ) 
 B_SPLINE_CURVE_WITH_KNOTS ( ( 4, 4 ),
 ( 2.436781329611979352, 3.141592653589793116 ),
 .UNSPECIFIED. ) 
 CURVE ( )  GEOMETRIC_REPRESENTATION_ITEM ( )  RATIONAL_B_SPLINE_CURVE ( ( 1.000000000000000000, 0.9590300661663082593, 0.9590300661663082593, 1.000000000000000000 ) ) 
 REPRESENTATION_ITEM ( '' )  );
#76225=ORIENTED_EDGE ( 'NONE', *, *, #43449, .T. ) ;
#76227=CARTESIAN_POINT ( 'NONE',  ( -16.66936639845670243, 1518.913060387330006, 180.4828114240741854 ) ) ;
#76228=ORIENTED_EDGE ( 'NONE', *, *, #22164, .F. ) ;
#76248=VERTEX_POINT ( 'NONE', #95070 ) ;
#76256=CARTESIAN_POINT ( 'NONE',  ( 18.02257621027576917, 1526.382868172863937, 182.8951942368371988 ) ) ;
#76267=CARTESIAN_POINT ( 'NONE',  ( -21.51496489921823851, 1524.872178180562969, 234.5520185365066652 ) ) ;
#76291=AXIS2_PLACEMENT_3D ( 'NONE', #67275, #40388, #75120 ) ;
#76294=CARTESIAN_POINT ( 'NONE',  ( -32.38114538885245963, 1523.604703353109699, 216.1203639561433647 ) ) ;
#76306=EDGE_CURVE ( 'NONE', #40681, #13824, #71582, .T. ) ;
#76309=CARTESIAN_POINT ( 'NONE',  ( -30.60461244942494119, 1523.621879633029039, 196.4204177336144426 ) ) ;
#76316=ADVANCED_FACE ( 'NONE', ( #2696 ), #96174, .T. ) ;
#76317=CARTESIAN_POINT ( 'NONE',  ( 21.84020450222056908, 1512.187213306747481, 234.9798068779740277 ) ) ;
#76319=CARTESIAN_POINT ( 'NONE',  ( 31.23437356469435144, 1512.187213306747481, 195.3468678195113739 ) ) ;
#76326=CARTESIAN_POINT ( 'NONE',  ( 17.26793975759715138, 1525.730671948510235, 181.5864082646643851 ) ) ;
#76327=CARTESIAN_POINT ( 'NONE',  ( -2.472529913803023227, 1523.678648413191695, 175.3762130535718597 ) ) ;
#76331=DIRECTION ( 'NONE',  ( 0.000000000000000000, 0.000000000000000000, -1.000000000000000000 ) ) ;
#76333=CARTESIAN_POINT ( 'NONE',  ( -16.66936639845609847, 1518.913060387330006, 237.7608804993221838 ) ) ;
#76336=CYLINDRICAL_SURFACE ( 'NONE', #19690, 1.000000000000001110 ) ;
#76349=EDGE_LOOP ( 'NONE', ( #60413, #82128, #36583, #80208 ) ) ;
#76355=ADVANCED_FACE ( 'NONE', ( #21093 ), #73748, .T. ) ;
#76364=ORIENTED_EDGE ( 'NONE', *, *, #16601, .F. ) ;
#76379=ORIENTED_EDGE ( 'NONE', *, *, #79257, .F. ) ;
#76389=DIRECTION ( 'NONE',  ( 0.000000000000000000, 1.000000000000000000, 0.000000000000000000 ) ) ;
#76396=CARTESIAN_POINT ( 'NONE',  ( -21.77174004986084555, 1524.860077346004800, 233.5882226505204642 ) ) ;
#76419=CARTESIAN_POINT ( 'NONE',  ( -33.28034951413127374, 1522.644714754858796, 217.4407153818779079 ) ) ;
#76420=CYLINDRICAL_SURFACE ( 'NONE', #75325, 33.13701971169416538 ) ;
#76425=DIRECTION ( 'NONE',  ( 0.7414773880254760252, -0.000000000000000000, 0.6709778558543624261 ) ) ;
#76429=CARTESIAN_POINT ( 'NONE',  ( -21.26060865160879843, 1525.055402519452628, 184.3612730374274520 ) ) ;
#76441=CARTESIAN_POINT ( 'NONE',  ( 16.62351968733444352, 1524.082582765195411, 180.5404605103855999 ) ) ;
#76442=DIRECTION ( 'NONE',  ( 0.000000000000000000, 1.000000000000000000, 0.000000000000000000 ) ) ;
#76444=ADVANCED_FACE ( 'NONE', ( #89426 ), #73181, .T. ) ;
#76456=DIRECTION ( 'NONE',  ( -0.3090169943749515036, 0.000000000000000000, -0.9510565162951521989 ) ) ;
#76461=AXIS2_PLACEMENT_3D ( 'NONE', #61436, #60316, #19383 ) ;
#76478=EDGE_CURVE ( 'NONE', #63483, #81290, #87687, .T. ) ;
#76479=CARTESIAN_POINT ( 'NONE',  ( 1.191524307911317804, 1526.382868172864164, 239.2353018730791518 ) ) ;
#76486=ORIENTED_EDGE ( 'NONE', *, *, #43179, .F. ) ;
#76487=CARTESIAN_POINT ( 'NONE',  ( 2.143764089412641738, 1525.848198008145346, 241.3832866758193632 ) ) ;
#76492=CYLINDRICAL_SURFACE ( 'NONE', #109194, 1.000000000000003553 ) ;
#76499=FACE_OUTER_BOUND ( 'NONE', #12136, .T. ) ;
#76517=CARTESIAN_POINT ( 'NONE',  ( -29.55269881708354873, 1525.821544997590991, 221.1141083160998448 ) ) ;
#76523=FACE_OUTER_BOUND ( 'NONE', #81673, .T. ) ;
#76532=DIRECTION ( 'NONE',  ( -0.000000000000000000, -1.000000000000000000, -0.000000000000000000 ) ) ;
#76534=CONICAL_SURFACE ( 'NONE', #64033, 23.69926344187880929, 1.195358426993359036 ) ;
#76542=ORIENTED_EDGE ( 'NONE', *, *, #71827, .F. ) ;
#76545=CARTESIAN_POINT ( 'NONE',  ( 3.143084115766277886, 1525.137906803777241, 176.7009701364783893 ) ) ;
#76556=CARTESIAN_POINT ( 'NONE',  ( 2.686147501205266686, 1526.329757971589288, 241.8500438829907182 ) ) ;
#76560=AXIS2_PLACEMENT_3D ( 'NONE', #89227, #12523, #46701 ) ;
#76564=VECTOR ( 'NONE', #27972, 1000.000000000000227 ) ;
#76572=AXIS2_PLACEMENT_3D ( 'NONE', #69531, #18515, #78456 ) ;
#76579=CARTESIAN_POINT ( 'NONE',  ( 32.40058737600813998, 1524.130440953581001, 216.9356993550890707 ) ) ;
#76585=CARTESIAN_POINT ( 'NONE',  ( -22.08622291482314282, 1518.913060387330006, 233.8253038720786776 ) ) ;
#76589=DIRECTION ( 'NONE',  ( 0.000000000000000000, 0.000000000000000000, 1.000000000000000000 ) ) ;
#76592=CARTESIAN_POINT ( 'NONE',  ( -21.53981368633734661, 1523.542365884046603, 234.3096115065273750 ) ) ;
#76626=VERTEX_POINT ( 'NONE', #1870 ) ;
#76634=DIRECTION ( 'NONE',  ( 0.8090169943749507819, -0.000000000000000000, 0.5877852522924685852 ) ) ;
#76646=TOROIDAL_SURFACE ( 'NONE', #22990, 2.000000000000000000, 1.000000000000000000 ) ;
#76658=LINE ( 'NONE', #93444, #15792 ) ;
#76672=CARTESIAN_POINT ( 'NONE',  ( -29.99620953741480278, 1524.382868172863937, 219.7462484079463252 ) ) ;
#76676=CARTESIAN_POINT ( 'NONE',  ( -32.23393008313284724, 1523.382868172864164, 201.4036600223109588 ) ) ;
#76678=CARTESIAN_POINT ( 'NONE',  ( 32.31945039880172033, 1524.082740465118377, 202.1440840643585943 ) ) ;
#76708=CARTESIAN_POINT ( 'NONE',  ( 1.436439550961320810, 1526.373507135059526, 178.7441892156120389 ) ) ;
#76718=CARTESIAN_POINT ( 'NONE',  ( 2.622430729442960740, 1523.621879633028811, 176.0901726876731459 ) ) ;
#76735=ORIENTED_EDGE ( 'NONE', *, *, #53067, .T. ) ;
#76799=VECTOR ( 'NONE', #50440, 1000.000000000000000 ) ;
#76804=DIRECTION ( 'NONE',  ( -0.000000000000000000, -1.000000000000000000, -0.000000000000000000 ) ) ;
#76808=DIRECTION ( 'NONE',  ( -0.000000000000000000, -1.000000000000000000, -0.000000000000000000 ) ) ;
#76837=EDGE_CURVE ( 'NONE', #20553, #38713, #83450, .T. ) ;
#76848=EDGE_CURVE ( 'NONE', #30026, #47770, #5426, .T. ) ;
#76855=AXIS2_PLACEMENT_3D ( 'NONE', #53050, #2107, #62586 ) ;
#76860=ORIENTED_EDGE ( 'NONE', *, *, #26231, .T. ) ;
#76875=CARTESIAN_POINT ( 'NONE',  ( -19.02270174366844913, 1526.382868172864164, 185.3889643600148815 ) ) ;
#76887=CARTESIAN_POINT ( 'NONE',  ( 17.72020223055846699, 1524.201670966335769, 180.4880726372848017 ) ) ;
#76903=AXIS2_PLACEMENT_3D ( 'NONE', #28401, #69319, #88309 ) ;
#76909=CARTESIAN_POINT ( 'NONE',  ( 21.92026280708336827, 1524.524650307258071, 184.5694803541689453 ) ) ;
#76910=ORIENTED_EDGE ( 'NONE', *, *, #104050, .T. ) ;
#76912=DIRECTION ( 'NONE',  ( 0.4090087482554189968, 4.257102464871849587E-15, -0.9125304618754023211 ) ) ;
#76942=AXIS2_PLACEMENT_3D ( 'NONE', #1297, #80756, #53366 ) ;
#76945=EDGE_LOOP ( 'NONE', ( #70153, #16079, #16639, #24573 ) ) ;
#76953=FACE_OUTER_BOUND ( 'NONE', #97021, .T. ) ;
#76955=CARTESIAN_POINT ( 'NONE',  ( 29.40443212115394189, 1511.187213306747708, 222.0897836382243042 ) ) ;
#76957=EDGE_CURVE ( 'NONE', #72801, #47896, #17860, .T. ) ;
#76963=CARTESIAN_POINT ( 'NONE',  ( 30.57819355944784689, 1525.253996226933623, 221.5701614757928439 ) ) ;
#76972=CIRCLE ( 'NONE', #28694, 30.10786454236638576 ) ;
#76982=EDGE_CURVE ( 'NONE', #81986, #8168, #39393, .T. ) ;
#76983=CIRCLE ( 'NONE', #9022, 1.000000000000000888 ) ;
#76996=CARTESIAN_POINT ( 'NONE',  ( -21.50863349123644142, 1524.374142163903798, 184.1251891552226994 ) ) ;
#77007=CARTESIAN_POINT ( 'NONE',  ( 31.40702543711169881, 1523.611961620354123, 196.3340613265677916 ) ) ;
#77012=FACE_OUTER_BOUND ( 'NONE', #4246, .T. ) ;
#77013=CARTESIAN_POINT ( 'NONE',  ( 32.86802468386284914, 1512.187213306747481, 201.0396662540042030 ) ) ;
#77017=ORIENTED_EDGE ( 'NONE', *, *, #63675, .T. ) ;
#77018=CIRCLE ( 'NONE', #46576, 1.000000000000000888 ) ;
#77024=CYLINDRICAL_SURFACE ( 'NONE', #6331, 1.999999999999994005 ) ;
#77025=DIRECTION ( 'NONE',  ( 0.9510565162951523099, 0.000000000000000000, -0.3090169943749515591 ) ) ;
#77030=CARTESIAN_POINT ( 'NONE',  ( -2.792392588003326903, 1526.382868172863937, 241.3440112565233164 ) ) ;
#77045=CARTESIAN_POINT ( 'NONE',  ( 1.191524307911315805, 1526.382868172864164, 239.2353018730791518 ) ) ;
#77047=FACE_OUTER_BOUND ( 'NONE', #82773, .T. ) ;
#77057=EDGE_LOOP ( 'NONE', ( #43310, #108588, #12484 ) ) ;
#77058=VERTEX_POINT ( 'NONE', #13673 ) ;
#77060=CARTESIAN_POINT ( 'NONE',  ( -21.76695791008670611, 1524.152349020271004, 183.4045362816220290 ) ) ;
#77076=DIRECTION ( 'NONE',  ( 0.000000000000000000, 1.000000000000000000, 0.000000000000000000 ) ) ;
#77087=EDGE_CURVE ( 'NONE', #92786, #62492, #93013, .T. ) ;
#77091=ORIENTED_EDGE ( 'NONE', *, *, #44061, .T. ) ;
#77097=AXIS2_PLACEMENT_3D ( 'NONE', #298, #42831, #845 ) ;
#77103=LINE ( 'NONE', #411, #102727 ) ;
#77119=CARTESIAN_POINT ( 'NONE',  ( 3.177670542995198133, 1525.042412244750722, 176.6379763401895673 ) ) ;
#77134=DIRECTION ( 'NONE',  ( 0.2054769195713318786, 0.000000000000000000, -0.9786619618251628516 ) ) ;
#77138=CARTESIAN_POINT ( 'NONE',  ( 29.16136750932905741, 1526.143142182216252, 220.6593063690870622 ) ) ;
#77142=FACE_OUTER_BOUND ( 'NONE', #107400, .T. ) ;
#77145=VECTOR ( 'NONE', #92764, 1000.000000000000000 ) ;
#77169=CARTESIAN_POINT ( 'NONE',  ( 32.86802468386292020, 1523.481610426287716, 217.2040256693915410 ) ) ;
#77187=CARTESIAN_POINT ( 'NONE',  ( -33.93019615848960768, 1501.977400791986611, 197.6607374646001176 ) ) ;
#77196=ORIENTED_EDGE ( 'NONE', *, *, #107194, .T. ) ;
#77198=CARTESIAN_POINT ( 'NONE',  ( -3.302453616664800418, 1524.523992613103019, 176.3738900077313758 ) ) ;
#77200=( BOUNDED_SURFACE ( )  B_SPLINE_SURFACE ( 3, 2, ( 
 ( #101245, #24544, #86682 ),
 ( #7763, #68809, #16147 ),
 ( #35177, #50351, #86134 ),
 ( #33498, #102911, #103470 ),
 ( #110781, #8309, #25100 ),
 ( #85015, #95090, #69360 ),
 ( #34072, #68265, #26777 ),
 ( #59846, #43041, #75546 ),
 ( #8858, #109682, #9427 ),
 ( #77198, #17793, #501 ),
 ( #26210, #60399, #51993 ),
 ( #43591, #77739, #53670 ),
 ( #71594, #105714, #79401 ),
 ( #44706, #96756, #27327 ) ),
 .UNSPECIFIED., .F., .F., .F. ) 
 B_SPLINE_SURFACE_WITH_KNOTS ( ( 4, 2, 2, 2, 2, 2, 4 ),
 ( 3, 3 ),
 ( 3.503057219300664826E-16, 0.0009443072508239316355, 0.001416460876235722246, 0.001888614501647512857, 0.002360768127059303251, 0.002832921752471094078, 0.003777229003294675300 ),
 ( 0.000000000000000000, 1.000000000000000000 ),
 .UNSPECIFIED. ) 
 GEOMETRIC_REPRESENTATION_ITEM ( )  RATIONAL_B_SPLINE_SURFACE ( (
 ( 1.000000000000000000, 0.9376006582765973318, 1.000000000000000000),
 ( 1.000000000000000000, 0.9283977714730347053, 1.000000000000000000),
 ( 1.000000000000000000, 0.9189750060488452998, 1.000000000000000000),
 ( 1.000000000000000000, 0.9042792056123225564, 1.000000000000000000),
 ( 1.000000000000000000, 0.8992469033844563420, 1.000000000000000000),
 ( 1.000000000000000000, 0.8891280264680836432, 1.000000000000000000),
 ( 1.000000000000000000, 0.8840337471678507697, 1.000000000000000000),
 ( 1.000000000000000000, 0.8736395124160363235, 1.000000000000000000),
 ( 1.000000000000000000, 0.8683406746552264632, 1.000000000000000000),
 ( 1.000000000000000000, 0.8573361860708257343, 1.000000000000000000),
 ( 1.000000000000000000, 0.8516508399493437631, 1.000000000000000000),
 ( 1.000000000000000000, 0.8340914917071454715, 1.000000000000000000),
 ( 1.000000000000000000, 0.8215597275857998705, 1.000000000000000000),
 ( 1.000000000000000000, 0.8070209408750025348, 1.000000000000000000) ) ) 
 REPRESENTATION_ITEM ( '' )  SURFACE ( )  );
#77220=EDGE_CURVE ( 'NONE', #108859, #25949, #76972, .T. ) ;
#77223=CARTESIAN_POINT ( 'NONE',  ( -31.12456774391156600, 1525.960063244517187, 217.0912716842400698 ) ) ;
#77238=CARTESIAN_POINT ( 'NONE',  ( -32.02808312589908013, 1511.187213306747708, 220.9649204700466782 ) ) ;
#77246=ORIENTED_EDGE ( 'NONE', *, *, #83786, .F. ) ;
#77299=DIRECTION ( 'NONE',  ( -0.8386695113602927742, -0.4884709562387165027, 0.2408932868012759743 ) ) ;
#77302=VERTEX_POINT ( 'NONE', #32968 ) ;
#77313=CARTESIAN_POINT ( 'NONE',  ( -30.45769963430608129, 1526.208281990539263, 217.1507671409966349 ) ) ;
#77320=DIRECTION ( 'NONE',  ( 0.000000000000000000, -1.000000000000000000, 0.000000000000000000 ) ) ;
#77339=VERTEX_POINT ( 'NONE', #5582 ) ;
#77340=EDGE_LOOP ( 'NONE', ( #16162, #10138, #37654, #52909 ) ) ;
#77343=DIRECTION ( 'NONE',  ( -0.03006000153037165917, -0.4884709562386974624, 0.8720622232497212689 ) ) ;
#77376=VERTEX_POINT ( 'NONE', #32439 ) ;
#77377=CARTESIAN_POINT ( 'NONE',  ( 28.54286204732486709, 1526.382868172863937, 198.4427524198199535 ) ) ;
#77378=CARTESIAN_POINT ( 'NONE',  ( 33.36586802512172767, 1512.187213306747481, 201.9069332299488622 ) ) ;
#77393=CARTESIAN_POINT ( 'NONE',  ( 0.4151546846821904668, 1524.726013923371283, 244.9330574173806383 ) ) ;
#77405=DIRECTION ( 'NONE',  ( 1.000000000000000000, 0.000000000000000000, 0.000000000000000000 ) ) ;
#77413=CARTESIAN_POINT ( 'NONE',  ( 21.63731731441962935, 1524.599984580802129, 234.6744441581147953 ) ) ;
#77415=CARTESIAN_POINT ( 'NONE',  ( 30.04349656869209895, 1524.760046179776054, 195.9289099819404214 ) ) ;
#77432=DIRECTION ( 'NONE',  ( 0.2054769195713296304, 0.000000000000000000, -0.9786619618251631847 ) ) ;
#77437=CARTESIAN_POINT ( 'NONE',  ( 16.97881484272545549, 1525.055402519452173, 181.2503677391246129 ) ) ;
#77452=( NAMED_UNIT ( * ) PLANE_ANGLE_UNIT ( ) SI_UNIT ( $, .RADIAN. ) );
#77458=CARTESIAN_POINT ( 'NONE',  ( 20.68299398337628858, 1525.856065479229073, 184.2887586734088643 ) ) ;
#77487=ADVANCED_FACE ( 'NONE', ( #72138 ), #63193, .T. ) ;
#77505=DIRECTION ( 'NONE',  ( -0.000000000000000000, -1.000000000000000000, -0.000000000000000000 ) ) ;
#77511=CARTESIAN_POINT ( 'NONE',  ( 29.86461515634920971, 1525.960063244517187, 220.9690070206020494 ) ) ;
#77521=CARTESIAN_POINT ( 'NONE',  ( 19.37182493330882593, 1526.345556099435726, 232.9230866865991629 ) ) ;
#77524=ADVANCED_FACE ( 'NONE', ( #11647 ), #54231, .F. ) ;
#77529=EDGE_LOOP ( 'NONE', ( #55371, #32853, #1594 ) ) ;
#77539=EDGE_CURVE ( 'NONE', #37235, #31591, #94784, .T. ) ;
#77541=CYLINDRICAL_SURFACE ( 'NONE', #77097, 0.9999999999999948930 ) ;
#77544=CARTESIAN_POINT ( 'NONE',  ( 19.92151515271105566, 1526.208281990539490, 184.7237256173480944 ) ) ;
#77550=TOROIDAL_SURFACE ( 'NONE', #41805, 30.13701971169416538, 3.000000000000000000 ) ;
#77552=CARTESIAN_POINT ( 'NONE',  ( -21.84020450222019250, 1523.382868172864164, 234.9798068779743403 ) ) ;
#77559=CARTESIAN_POINT ( 'NONE',  ( 31.81407709660777527, 1501.977400791986611, 221.9534378623329758 ) ) ;
#77591=CARTESIAN_POINT ( 'NONE',  ( -31.52384429374384567, 1525.730671948512054, 201.2079775281771390 ) ) ;
#77603=ORIENTED_EDGE ( 'NONE', *, *, #100368, .T. ) ;
#77604=DIRECTION ( 'NONE',  ( 0.9510565162951478690, 0.000000000000000000, -0.3090169943749654369 ) ) ;
#77606=EDGE_CURVE ( 'NONE', #12203, #96482, #44166, .T. ) ;
#77614=CARTESIAN_POINT ( 'NONE',  ( 3.687149994097108433E-15, 1518.913060387330006, 239.2297105040643714 ) ) ;
#77628=AXIS2_PLACEMENT_3D ( 'NONE', #73783, #30656, #64841 ) ;
#77630=CARTESIAN_POINT ( 'NONE',  ( -29.53441971554730472, 1525.651286436461760, 221.7311721888731881 ) ) ;
#77642=DIRECTION ( 'NONE',  ( 0.5877852522924762457, 0.000000000000000000, 0.8090169943749451198 ) ) ;
#77659=CARTESIAN_POINT ( 'NONE',  ( -29.85692059557563027, 1525.159177407156221, 196.1177194699280903 ) ) ;
#77669=FACE_OUTER_BOUND ( 'NONE', #64350, .T. ) ;
#77677=CARTESIAN_POINT ( 'NONE',  ( 28.72841836130201543, 1526.333389947990099, 220.1290250959143862 ) ) ;
#77683=DIRECTION ( 'NONE',  ( 0.9942586961433764747, -0.000000000000000000, 0.1070030146457237041 ) ) ;
#77686=ORIENTED_EDGE ( 'NONE', *, *, #14374, .F. ) ;
#77687=DIRECTION ( 'NONE',  ( -0.8090169943749534465, -0.000000000000000000, -0.5877852522924650325 ) ) ;
#77695=CARTESIAN_POINT ( 'NONE',  ( 18.51436573157378618, 1511.187213306747708, 237.1421867457405881 ) ) ;
#77699=EDGE_CURVE ( 'NONE', #83466, #31153, #72776, .T. ) ;
#77700=AXIS2_PLACEMENT_3D ( 'NONE', #3311, #104637, #103524 ) ;
#77729=EDGE_LOOP ( 'NONE', ( #85418, #69909, #33935, #30781 ) ) ;
#77739=CARTESIAN_POINT ( 'NONE',  ( -2.692976938448824242, 1524.059547553519678, 176.1570252011561593 ) ) ;
#77748=ORIENTED_EDGE ( 'NONE', *, *, #11102, .T. ) ;
#77755=ORIENTED_EDGE ( 'NONE', *, *, #42986, .F. ) ;
#77758=DIRECTION ( 'NONE',  ( 0.000000000000000000, 0.000000000000000000, 1.000000000000000000 ) ) ;
#77770=ORIENTED_EDGE ( 'NONE', *, *, #72677, .F. ) ;
#77787=CARTESIAN_POINT ( 'NONE',  ( 2.596261494520144986, 1525.907212628473872, 240.7735774411710850 ) ) ;
#77789=CARTESIAN_POINT ( 'NONE',  ( -1.909775791882407869, 1526.107880201381477, 177.3667237755819031 ) ) ;
#77795=B_SPLINE_CURVE_WITH_KNOTS ( 'NONE', 3,
 ( #5079, #16080, #39796, #85492, #108085, #76011, #31380, #84945 ),
 .UNSPECIFIED., .F., .F.,
 ( 4, 2, 2, 4 ),
 ( 2.964296775167216948E-17, 0.001073044933456093883, 0.001609567400184125970, 0.002146089866912157841 ),
 .UNSPECIFIED. ) ;
#77834=CARTESIAN_POINT ( 'NONE',  ( -17.17241001986523941, 1511.187213306747708, 179.6185504016045797 ) ) ;
#77839=DIRECTION ( 'NONE',  ( 0.000000000000000000, 1.000000000000000000, 0.000000000000000000 ) ) ;
#77842=ORIENTED_EDGE ( 'NONE', *, *, #20828, .T. ) ;
#77845=( BOUNDED_SURFACE ( )  B_SPLINE_SURFACE ( 3, 2, ( 
 ( #12121, #21605, #64204 ),
 ( #38962, #97776, #30014 ),
 ( #4292, #29468, #30577 ),
 ( #89927, #73140, #63661 ),
 ( #72595, #46313, #62575 ),
 ( #21051, #107283, #55254 ),
 ( #80442, #98327, #19402 ),
 ( #11579, #89386, #12677 ),
 ( #19964, #38419, #3207 ),
 ( #45756, #45198, #96127 ),
 ( #46857, #106723, #79893 ),
 ( #4816, #105086, #63126 ),
 ( #55810, #28936, #2650 ),
 ( #47392, #54159, #36778 ) ),
 .UNSPECIFIED., .F., .F., .F. ) 
 B_SPLINE_SURFACE_WITH_KNOTS ( ( 4, 2, 2, 2, 2, 2, 4 ),
 ( 3, 3 ),
 ( 0.000000000000000000, 0.0009440840677143950543, 0.001416126101571592473, 0.001888168135428790109, 0.002360210169285987744, 0.002832252203143184946, 0.003776336270857580217 ),
 ( 0.000000000000000000, 1.000000000000000000 ),
 .UNSPECIFIED. ) 
 GEOMETRIC_REPRESENTATION_ITEM ( )  RATIONAL_B_SPLINE_SURFACE ( (
 ( 1.000000000000000000, 0.8070209408750095292, 1.000000000000000000),
 ( 1.000000000000000000, 0.8215603905278417995, 1.000000000000000000),
 ( 1.000000000000000000, 0.8340988699068413448, 1.000000000000000000),
 ( 1.000000000000000000, 0.8516751610454839083, 1.000000000000000000),
 ( 1.000000000000000000, 0.8573697395150315925, 1.000000000000000000),
 ( 1.000000000000000000, 0.8683586635666024067, 1.000000000000000000),
 ( 1.000000000000000000, 0.8736518481709272255, 1.000000000000000000),
 ( 1.000000000000000000, 0.8840377753029367014, 1.000000000000000000),
 ( 1.000000000000000000, 0.8891294171307203564, 1.000000000000000000),
 ( 1.000000000000000000, 0.8992456600573149883, 1.000000000000000000),
 ( 1.000000000000000000, 0.9042785869252324416, 1.000000000000000000),
 ( 1.000000000000000000, 0.9189749222839583842, 1.000000000000000000),
 ( 1.000000000000000000, 0.9283978182347645269, 1.000000000000000000),
 ( 1.000000000000000000, 0.9376006582765933350, 1.000000000000000000) ) ) 
 REPRESENTATION_ITEM ( '' )  SURFACE ( )  );
#77856=CARTESIAN_POINT ( 'NONE',  ( -29.52630218505378323, 1525.661276915132476, 221.7199201227869310 ) ) ;
#77858=CARTESIAN_POINT ( 'NONE',  ( -2.038646110889675178, 1525.960063244516959, 177.0579350083066004 ) ) ;
#77863=LINE ( 'NONE', #43165, #27703 ) ;
#77871=EDGE_CURVE ( 'NONE', #70982, #73683, #47767, .T. ) ;
#77887=ORIENTED_EDGE ( 'NONE', *, *, #16854, .F. ) ;
#77893=VECTOR ( 'NONE', #24893, 1000.000000000000000 ) ;
#77921=CARTESIAN_POINT ( 'NONE',  ( 29.61076270571687630, 1526.107880201381477, 197.4926688362025402 ) ) ;
#77922=CARTESIAN_POINT ( 'NONE',  ( -18.19590854888186726, 1522.382868172863937, 180.0410247165186206 ) ) ;
#77951=CARTESIAN_POINT ( 'NONE',  ( 21.83550407203919974, 1523.678648413191695, 234.9693198511250785 ) ) ;
#77954=DIRECTION ( 'NONE',  ( -0.8672669759446604010, 6.017873532443123780E-15, 0.4978433412588780804 ) ) ;
#77961=CARTESIAN_POINT ( 'NONE',  ( -20.79738390328759223, 1511.187213306747708, 181.2030061003473236 ) ) ;
#77962=CARTESIAN_POINT ( 'NONE',  ( 29.40443212115383531, 1512.187213306747481, 196.1539082851714966 ) ) ;
#77976=CARTESIAN_POINT ( 'NONE',  ( -1.393816646507355372, 1511.187213306747708, 175.1051575864439656 ) ) ;
#77979=CARTESIAN_POINT ( 'NONE',  ( 16.88555894881584862, 1525.556090473913855, 181.6768911977973744 ) ) ;
#77992=CYLINDRICAL_SURFACE ( 'NONE', #76942, 1.999999999999995559 ) ;
#78000=CARTESIAN_POINT ( 'NONE',  ( 22.08327125186924533, 1523.604703353109699, 184.4267662568470314 ) ) ;
#78001=ORIENTED_EDGE ( 'NONE', *, *, #87830, .F. ) ;
#78004=CARTESIAN_POINT ( 'NONE',  ( -17.17241001986462123, 1518.913060387330006, 237.6251415217917895 ) ) ;
#78054=CARTESIAN_POINT ( 'NONE',  ( 30.44070839969077014, 1525.425665131984488, 221.4735044094857699 ) ) ;
#78062=EDGE_CURVE ( 'NONE', #38471, #100597, #67327, .T. ) ;
#78079=CARTESIAN_POINT ( 'NONE',  ( -19.01764264267205817, 1526.373507135059981, 232.8535685347059427 ) ) ;
#78082=DIRECTION ( 'NONE',  ( 0.000000000000000000, 0.000000000000000000, 1.000000000000000000 ) ) ;
#78097=AXIS2_PLACEMENT_3D ( 'NONE', #29736, #46571, #20231 ) ;
#78106=ORIENTED_EDGE ( 'NONE', *, *, #64421, .F. ) ;
#78111=CARTESIAN_POINT ( 'NONE',  ( 3.347801439296147041, 1523.382868172864164, 176.1543725841967500 ) ) ;
#78116=DIRECTION ( 'NONE',  ( -0.4090087482554316534, -0.000000000000000000, -0.9125304618753967700 ) ) ;
#78127=CARTESIAN_POINT ( 'NONE',  ( -31.92312126443670905, 1524.775785348137561, 201.5796050126409966 ) ) ;
#78135=CARTESIAN_POINT ( 'NONE',  ( 29.99620953741496976, 1524.382868172863937, 219.7462484079458704 ) ) ;
#78145=AXIS2_PLACEMENT_3D ( 'NONE', #58788, #95935, #68315 ) ;
#78172=EDGE_CURVE ( 'NONE', #68723, #107075, #90587, .T. ) ;
#78189=EDGE_CURVE ( 'NONE', #20574, #36754, #83545, .T. ) ;
#78204=CARTESIAN_POINT ( 'NONE',  ( -33.72300830903907354, 1524.397344074319108, 198.6568221122821001 ) ) ;
#78207=CARTESIAN_POINT ( 'NONE',  ( -29.13505175353617105, 1526.073429442291854, 221.0961561632167047 ) ) ;
#78218=AXIS2_PLACEMENT_3D ( 'NONE', #69149, #95439, #52899 ) ;
#78239=CARTESIAN_POINT ( 'NONE',  ( 29.17014196280698357, 1526.382868172864164, 201.0245104653888006 ) ) ;
#78246=DIRECTION ( 'NONE',  ( -1.000000000000000000, -0.000000000000000000, 0.000000000000000000 ) ) ;
#78260=DIRECTION ( 'NONE',  ( -1.000000000000000000, 0.000000000000000000, 0.000000000000000000 ) ) ;
#78265=DIRECTION ( 'NONE',  ( 0.000000000000000000, 0.000000000000000000, 1.000000000000000000 ) ) ;
#78271=ORIENTED_EDGE ( 'NONE', *, *, #94728, .F. ) ;
#78277=AXIS2_PLACEMENT_3D ( 'NONE', #29719, #99660, #38122 ) ;
#78295=ADVANCED_FACE ( 'NONE', ( #71761 ), #56715, .T. ) ;
#78302=CIRCLE ( 'NONE', #108759, 2.000000000000000444 ) ;
#78303=CARTESIAN_POINT ( 'NONE',  ( 2.372478608332516892, 1522.862737210649811, 174.8996806668726549 ) ) ;
#78336=CARTESIAN_POINT ( 'NONE',  ( 3.017174818680797177, 1525.408337840050081, 241.3338438474178815 ) ) ;
#78337=ORIENTED_EDGE ( 'NONE', *, *, #100969, .T. ) ;
#78356=CARTESIAN_POINT ( 'NONE',  ( -1.961418762362024282, 1526.143142182216707, 240.4212258933359578 ) ) ;
#78358=AXIS2_PLACEMENT_3D ( 'NONE', #75626, #25178, #109760 ) ;
#78359=ADVANCED_FACE ( 'NONE', ( #72557 ), #38382, .T. ) ;
#78374=CARTESIAN_POINT ( 'NONE',  ( 22.08327125186944428, 1523.604703353109699, 233.8169256665487694 ) ) ;
#78375=CARTESIAN_POINT ( 'NONE',  ( -32.21013329178911988, 1524.412928176729110, 216.0988866155133508 ) ) ;
#78378=ORIENTED_EDGE ( 'NONE', *, *, #49397, .T. ) ;
#78394=ORIENTED_EDGE ( 'NONE', *, *, #54820, .F. ) ;
#78401=CARTESIAN_POINT ( 'NONE',  ( -30.80549360313072427, 1524.130440953581001, 221.8448932001217031 ) ) ;
#78403=CARTESIAN_POINT ( 'NONE',  ( 32.21013329178848750, 1524.412928176728428, 202.1448053078787552 ) ) ;
#78416=ORIENTED_EDGE ( 'NONE', *, *, #87728, .F. ) ;
#78437=ORIENTED_EDGE ( 'NONE', *, *, #88419, .F. ) ;
#78442=CIRCLE ( 'NONE', #13994, 1.000000000000000888 ) ;
#78456=DIRECTION ( 'NONE',  ( -0.9125304618754029873, 0.000000000000000000, -0.4090087482554177756 ) ) ;
#78457=ORIENTED_EDGE ( 'NONE', *, *, #96154, .F. ) ;
#78462=CARTESIAN_POINT ( 'NONE',  ( 32.86802468386292730, 1501.977400791986611, 217.2040256693915410 ) ) ;
#78465=CARTESIAN_POINT ( 'NONE',  ( 32.38845791999500534, 1523.382868172864164, 216.1254071228445639 ) ) ;
#78479=CARTESIAN_POINT ( 'NONE',  ( -18.10570579381849043, 1525.713797967456912, 180.1226510103712144 ) ) ;
#78481=CYLINDRICAL_SURFACE ( 'NONE', #70620, 33.13701971169416538 ) ;
#78499=CARTESIAN_POINT ( 'NONE',  ( -33.45065857237986506, 1524.841055067849993, 219.4656524796156987 ) ) ;
#78501=CARTESIAN_POINT ( 'NONE',  ( -20.55201027734695884, 1526.382868172863937, 236.4070436938631872 ) ) ;
#78513=CARTESIAN_POINT ( 'NONE',  ( 21.96543842109177902, 1523.313115944345327, 235.2592135320308273 ) ) ;
#78516=ORIENTED_EDGE ( 'NONE', *, *, #1118, .F. ) ;
#78517=CARTESIAN_POINT ( 'NONE',  ( -31.23437356469425907, 1512.187213306747481, 221.8968241038848248 ) ) ;
#78520=DIRECTION ( 'NONE',  ( 0.000000000000000000, 0.000000000000000000, -1.000000000000000000 ) ) ;
#78555=ORIENTED_EDGE ( 'NONE', *, *, #100179, .F. ) ;
#78559=CARTESIAN_POINT ( 'NONE',  ( 21.53712143570552939, 1523.621879633028811, 183.9400870382961841 ) ) ;
#78566=CIRCLE ( 'NONE', #35623, 2.000000000000009770 ) ;
#78577=ORIENTED_EDGE ( 'NONE', *, *, #75537, .F. ) ;
#78593=ORIENTED_EDGE ( 'NONE', *, *, #28685, .T. ) ;
#78595=DIRECTION ( 'NONE',  ( 0.000000000000000000, 1.000000000000000000, 0.000000000000000000 ) ) ;
#78596=EDGE_LOOP ( 'NONE', ( #46781, #109657, #62594, #43752 ) ) ;
#78599=CARTESIAN_POINT ( 'NONE',  ( -34.18677586421195258, 1522.382868172863937, 198.4504086008750505 ) ) ;
#78602=CARTESIAN_POINT ( 'NONE',  ( -2.372478608332516892, 1522.382868172863937, 174.8996806668726549 ) ) ;
#78616=CARTESIAN_POINT ( 'NONE',  ( 29.91204167771608269, 1525.042412244735488, 222.1820579943630776 ) ) ;
#78619=CARTESIAN_POINT ( 'NONE',  ( -16.94363731710831189, 1525.231909165016305, 236.8652039782725751 ) ) ;
#78620=CIRCLE ( 'NONE', #107221, 0.9999999999999976685 ) ;
#78647=ORIENTED_EDGE ( 'NONE', *, *, #58040, .T. ) ;
#78648=AXIS2_PLACEMENT_3D ( 'NONE', #101492, #50026, #41620 ) ;
#78654=CARTESIAN_POINT ( 'NONE',  ( -30.31404213106243617, 1524.330813522192102, 196.4516891724783534 ) ) ;
#78667=LINE ( 'NONE', #8136, #59983 ) ;
#78668=LINE ( 'NONE', #96014, #28518 ) ;
#78677=DIRECTION ( 'NONE',  ( -4.440892098500627739E-15, 0.000000000000000000, -1.000000000000000000 ) ) ;
#78682=ORIENTED_EDGE ( 'NONE', *, *, #48069, .F. ) ;
#78691=CARTESIAN_POINT ( 'NONE',  ( -32.05702909905236453, 1524.477587234266139, 201.5541149372814402 ) ) ;
#78692=ADVANCED_FACE ( 'NONE', ( #83154 ), #85677, .F. ) ;
#78706=ORIENTED_EDGE ( 'NONE', *, *, #82080, .F. ) ;
#78734=CARTESIAN_POINT ( 'NONE',  ( -30.44069153017106544, 1525.425686270225015, 221.4734925813270081 ) ) ;
#78758=CARTESIAN_POINT ( 'NONE',  ( 3.451191875628180750, 1523.678648413191695, 175.1707361340005207 ) ) ;
#78759=EDGE_LOOP ( 'NONE', ( #83238, #85276, #13543, #57457 ) ) ;
#78761=B_SPLINE_CURVE_WITH_KNOTS ( 'NONE', 3,
 ( #35942, #47641, #72310, #90169, #12917, #82340 ),
 .UNSPECIFIED., .F., .F.,
 ( 4, 2, 4 ),
 ( 1.040834085586084257E-17, 0.001087661325621735488, 0.002175322651243460567 ),
 .UNSPECIFIED. ) ;
#78765=CARTESIAN_POINT ( 'NONE',  ( -34.61172972909721324, 1523.342713519622976, 200.0387150244875443 ) ) ;
#78799=ORIENTED_EDGE ( 'NONE', *, *, #23975, .F. ) ;
#78819=CARTESIAN_POINT ( 'NONE',  ( -29.99620953741502660, 1524.382868172863937, 198.4974435154502999 ) ) ;
#78822=EDGE_CURVE ( 'NONE', #105990, #100644, #81693, .T. ) ;
#78823=( BOUNDED_SURFACE ( )  B_SPLINE_SURFACE ( 3, 2, ( 
 ( #19308, #897, #61369 ),
 ( #61920, #10939, #87653 ),
 ( #95488, #26618, #77591 ),
 ( #36142, #45114, #79809 ),
 ( #19871, #18755, #88201 ),
 ( #45671, #87087, #10371 ),
 ( #35022, #60813, #86529 ),
 ( #17642, #78127, #9280 ),
 ( #3115, #9824, #44545 ),
 ( #43992, #78691, #85981 ),
 ( #37243, #1431, #2007 ),
 ( #51844, #26049, #2566 ),
 ( #36688, #35574, #94361 ),
 ( #69768, #47845, #39444 ) ),
 .UNSPECIFIED., .F., .F., .F. ) 
 B_SPLINE_SURFACE_WITH_KNOTS ( ( 4, 2, 2, 2, 2, 2, 4 ),
 ( 3, 3 ),
 ( 6.873841773558098112E-17, 0.0009443072508236353231, 0.001416460876235418670, 0.001888614501647201908, 0.002360768127058984929, 0.002832921752470768384, 0.003777229003294335294 ),
 ( 0.000000000000000000, 1.000000000000000000 ),
 .UNSPECIFIED. ) 
 GEOMETRIC_REPRESENTATION_ITEM ( )  RATIONAL_B_SPLINE_SURFACE ( (
 ( 1.000000000000000000, 0.9376006582765963326, 1.000000000000000000),
 ( 1.000000000000000000, 0.9283977714734873432, 1.000000000000000000),
 ( 1.000000000000000000, 0.9189750060482670957, 1.000000000000000000),
 ( 1.000000000000000000, 0.9042792056126127687, 1.000000000000000000),
 ( 1.000000000000000000, 0.8992469033848606852, 1.000000000000000000),
 ( 1.000000000000000000, 0.8891280264676786338, 1.000000000000000000),
 ( 1.000000000000000000, 0.8840337471672635727, 1.000000000000000000),
 ( 1.000000000000000000, 0.8736395124166199677, 1.000000000000000000),
 ( 1.000000000000000000, 0.8683406746562497558, 1.000000000000000000),
 ( 1.000000000000000000, 0.8573361860698035519, 1.000000000000000000),
 ( 1.000000000000000000, 0.8516508399500833937, 1.000000000000000000),
 ( 1.000000000000000000, 0.8340914917056792000, 1.000000000000000000),
 ( 1.000000000000000000, 0.8215597275869019889, 1.000000000000000000),
 ( 1.000000000000000000, 0.8070209408750123048, 1.000000000000000000) ) ) 
 REPRESENTATION_ITEM ( '' )  SURFACE ( )  );
#78831=CARTESIAN_POINT ( 'NONE',  ( 33.42844755917195698, 1501.977400791986611, 222.1271778627166213 ) ) ;
#78841=LINE ( 'NONE', #2152, #19349 ) ;
#78844=ADVANCED_FACE ( 'NONE', ( #59491 ), #51084, .T. ) ;
#78845=ORIENTED_EDGE ( 'NONE', *, *, #39222, .T. ) ;
#78847=CIRCLE ( 'NONE', #132, 1.000000000000000888 ) ;
#78850=CARTESIAN_POINT ( 'NONE',  ( -2.470168521978402421, 1523.481610426287716, 242.8787258963054398 ) ) ;
#78857=CARTESIAN_POINT ( 'NONE',  ( -28.82451532742571487, 1526.348417187218956, 198.1911182592219518 ) ) ;
#78886=ORIENTED_EDGE ( 'NONE', *, *, #67514, .T. ) ;
#78943=CARTESIAN_POINT ( 'NONE',  ( -32.70814417905852167, 1524.201816949777822, 217.1264145000764074 ) ) ;
#78951=EDGE_CURVE ( 'NONE', #100304, #22289, #67002, .T. ) ;
#78954=DIRECTION ( 'NONE',  ( 0.4978433412588781914, 0.000000000000000000, 0.8672669759446606230 ) ) ;
#78973=CARTESIAN_POINT ( 'NONE',  ( -31.76119286153722499, 1522.906363951597314, 221.9477464134160414 ) ) ;
#78979=DIRECTION ( 'NONE',  ( 0.000000000000000000, 1.000000000000000000, 0.000000000000000000 ) ) ;
#78980=EDGE_CURVE ( 'NONE', #36364, #56488, #103269, .T. ) ;
#78989=ORIENTED_EDGE ( 'NONE', *, *, #110441, .T. ) ;
#79012=AXIS2_PLACEMENT_3D ( 'NONE', #48096, #45096, #79236 ) ;
#79015=ADVANCED_FACE ( 'NONE', ( #8918 ), #83422, .T. ) ;
#79016=FACE_OUTER_BOUND ( 'NONE', #15192, .T. ) ;
#79048=DIRECTION ( 'NONE',  ( 0.01594118961724032973, -0.9969860201949399814, -0.07592597717146747083 ) ) ;
#79049=CARTESIAN_POINT ( 'NONE',  ( -19.39983987835444879, 1522.382868172863937, 178.9515629539737631 ) ) ;
#79054=DIRECTION ( 'NONE',  ( 0.000000000000000000, 0.000000000000000000, -1.000000000000000000 ) ) ;
#79056=DIRECTION ( 'NONE',  ( -0.4090087482554316534, 0.000000000000000000, -0.9125304618753967700 ) ) ;
#79068=CARTESIAN_POINT ( 'NONE',  ( -32.40058737600715233, 1524.130440953581001, 216.9356993550890138 ) ) ;
#79096=DIRECTION ( 'NONE',  ( -1.000000000000000000, 0.000000000000000000, 0.000000000000000000 ) ) ;
#79117=CARTESIAN_POINT ( 'NONE',  ( -2.596261494520238688, 1525.907212628473644, 240.7735774411713123 ) ) ;
#79119=CIRCLE ( 'NONE', #25436, 1.000000000000000888 ) ;
#79140=EDGE_LOOP ( 'NONE', ( #101442, #41928, #90136, #60717, #7771 ) ) ;
#79144=VERTEX_POINT ( 'NONE', #4931 ) ;
#79151=EDGE_CURVE ( 'NONE', #96612, #14943, #13310, .T. ) ;
#79152=EDGE_CURVE ( 'NONE', #21147, #32555, #108575, .T. ) ;
#79157=DIRECTION ( 'NONE',  ( 0.000000000000000000, 1.000000000000000000, 0.000000000000000000 ) ) ;
#79172=CYLINDRICAL_SURFACE ( 'NONE', #20685, 0.9999999999999942268 ) ;
#79185=CARTESIAN_POINT ( 'NONE',  ( 30.95230591800835995, 1524.659802833170943, 221.7850325738306765 ) ) ;
#79188=CARTESIAN_POINT ( 'NONE',  ( -16.54283724222759488, 1524.843178112495707, 237.3984430206447200 ) ) ;
#79201=DIRECTION ( 'NONE',  ( -0.9786619618251657382, 0.000000000000000000, 0.2054769195713179730 ) ) ;
#79220=CARTESIAN_POINT ( 'NONE',  ( -31.97743984922253446, 1525.878013734321030, 198.0760624713092284 ) ) ;
#79230=VERTEX_POINT ( 'NONE', #106299 ) ;
#79236=DIRECTION ( 'NONE',  ( -0.8090169943749507819, 0.000000000000000000, -0.5877852522924685852 ) ) ;
#79248=ORIENTED_EDGE ( 'NONE', *, *, #5642, .F. ) ;
#79257=EDGE_CURVE ( 'NONE', #99467, #32820, #21227, .T. ) ;
#79258=DIRECTION ( 'NONE',  ( -0.2054769195713296581, 0.000000000000000000, 0.9786619618251632957 ) ) ;
#79310=AXIS2_PLACEMENT_3D ( 'NONE', #109513, #73156, #65322 ) ;
#79315=ORIENTED_EDGE ( 'NONE', *, *, #8708, .F. ) ;
#79321=CARTESIAN_POINT ( 'NONE',  ( -20.92767404034537648, 1511.187213306747708, 182.8548762971666406 ) ) ;
#79323=CARTESIAN_POINT ( 'NONE',  ( -33.52308185467866508, 1525.402221411349728, 200.6636391946740616 ) ) ;
#79332=CARTESIAN_POINT ( 'NONE',  ( 0.4151546846821905778, 1522.382868172863937, 244.9330574173806951 ) ) ;
#79339=CARTESIAN_POINT ( 'NONE',  ( -30.31940284292399213, 1518.913060387330006, 222.4933038710547919 ) ) ;
#79362=B_SPLINE_CURVE_WITH_KNOTS ( 'NONE', 3,
 ( #5377, #108391, #108945, #90476 ),
 .UNSPECIFIED., .F., .F.,
 ( 4, 4 ),
 ( 0.000000000000000000, 0.0002220129587134773411 ),
 .UNSPECIFIED. ) ;
#79388=CARTESIAN_POINT ( 'NONE',  ( 18.86688640473602874, 1511.187213306747708, 237.4611898188519774 ) ) ;
#79401=CARTESIAN_POINT ( 'NONE',  ( -2.487421823092379913, 1523.954914175592194, 175.4471414341940942 ) ) ;
#79402=CARTESIAN_POINT ( 'NONE',  ( 29.78220350812342332, 1526.382868172863937, 196.5089261231633202 ) ) ;
#79415=ORIENTED_EDGE ( 'NONE', *, *, #88448, .T. ) ;
#79446=CARTESIAN_POINT ( 'NONE',  ( -32.86470158750932313, 1523.580203803270933, 217.2021180890991445 ) ) ;
#79451=EDGE_CURVE ( 'NONE', #81018, #71944, #29988, .T. ) ;
#79472=AXIS2_PLACEMENT_3D ( 'NONE', #105115, #90919, #14205 ) ;
#79473=DIRECTION ( 'NONE',  ( -0.8672669759446666182, 0.000000000000000000, -0.4978433412588672557 ) ) ;
#79494=CARTESIAN_POINT ( 'NONE',  ( 33.36586802512179162, 1512.187213306747481, 216.3367586934468818 ) ) ;
#79504=EDGE_CURVE ( 'NONE', #71507, #97242, #33646, .T. ) ;
#79515=CARTESIAN_POINT ( 'NONE',  ( 31.92299894892067513, 1524.776010967693537, 201.5796163247183870 ) ) ;
#79523=CARTESIAN_POINT ( 'NONE',  ( 19.39983987835422496, 1522.382868172863937, 239.2921289694223219 ) ) ;
#79545=EDGE_LOOP ( 'NONE', ( #60847, #55181, #81636, #90233 ) ) ;
#79554=AXIS2_PLACEMENT_3D ( 'NONE', #80821, #106568, #81903 ) ;
#79556=VECTOR ( 'NONE', #11864, 1000.000000000000000 ) ;
#79563=ORIENTED_EDGE ( 'NONE', *, *, #73548, .T. ) ;
#79569=ORIENTED_EDGE ( 'NONE', *, *, #62533, .T. ) ;
#79570=ORIENTED_EDGE ( 'NONE', *, *, #81012, .F. ) ;
#79580=FACE_OUTER_BOUND ( 'NONE', #14930, .T. ) ;
#79591=CARTESIAN_POINT ( 'NONE',  ( -20.85167258424259629, 1525.730671215490020, 234.0535516931209656 ) ) ;
#79618=EDGE_CURVE ( 'NONE', #61077, #20210, #80037, .T. ) ;
#79630=ORIENTED_EDGE ( 'NONE', *, *, #89939, .T. ) ;
#79633=CARTESIAN_POINT ( 'NONE',  ( 31.81407709660768290, 1522.382868172863937, 196.2902540610627682 ) ) ;
#79634=EDGE_CURVE ( 'NONE', #82322, #71856, #14720, .T. ) ;
#79638=CARTESIAN_POINT ( 'NONE',  ( -30.01483979339426966, 1525.231887713368451, 196.6362079710710020 ) ) ;
#79664=CARTESIAN_POINT ( 'NONE',  ( 16.56943046651975848, 1526.189899547014875, 235.5982391528384312 ) ) ;
#79668=DIRECTION ( 'NONE',  ( 0.000000000000000000, 0.000000000000000000, -1.000000000000000000 ) ) ;
#79678=AXIS2_PLACEMENT_3D ( 'NONE', #45191, #107274, #45749 ) ;
#79688=CIRCLE ( 'NONE', #86852, 1.000000000000005551 ) ;
#79695=VERTEX_POINT ( 'NONE', #41026 ) ;
#79703=LINE ( 'NONE', #96489, #65804 ) ;
#79712=DIRECTION ( 'NONE',  ( 0.000000000000000000, 0.000000000000000000, 1.000000000000000000 ) ) ;
#79713=ORIENTED_EDGE ( 'NONE', *, *, #82353, .F. ) ;
#79727=CARTESIAN_POINT ( 'NONE',  ( 0.000000000000000000, 1523.382868172864164, 209.1218459616979999 ) ) ;
#79732=DIRECTION ( 'NONE',  ( 0.000000000000000000, 0.000000000000000000, 1.000000000000000000 ) ) ;
#79734=EDGE_LOOP ( 'NONE', ( #100785, #492, #52819, #3715 ) ) ;
#79735=CARTESIAN_POINT ( 'NONE',  ( -17.42134945962463988, 1525.253972588476699, 237.1661777806035332 ) ) ;
#79737=ADVANCED_FACE ( 'NONE', ( #30831 ), #90739, .T. ) ;
#79738=CARTESIAN_POINT ( 'NONE',  ( 29.00779973304128134, 1526.382868172864164, 217.2942086403122630 ) ) ;
#79755=DIRECTION ( 'NONE',  ( 0.3090169943749515591, -0.000000000000000000, 0.9510565162951523099 ) ) ;
#79758=LINE ( 'NONE', #6183, #87899 ) ;
#79775=DIRECTION ( 'NONE',  ( 0.000000000000000000, 1.000000000000000000, 0.000000000000000000 ) ) ;
#79799=CARTESIAN_POINT ( 'NONE',  ( -3.348648543330357441, 1523.530935881284904, 242.0864759303845801 ) ) ;
#79800=ORIENTED_EDGE ( 'NONE', *, *, #956, .T. ) ;
#79801=VERTEX_POINT ( 'NONE', #35607 ) ;
#79802=CIRCLE ( 'NONE', #101173, 1.000000000000000888 ) ;
#79805=FACE_OUTER_BOUND ( 'NONE', #8754, .T. ) ;
#79809=CARTESIAN_POINT ( 'NONE',  ( -31.79805362023597226, 1525.506926151470680, 201.2206259782555549 ) ) ;
#79820=CARTESIAN_POINT ( 'NONE',  ( 21.11881948555302557, 1525.651286436460168, 233.3142521953524238 ) ) ;
#79821=ORIENTED_EDGE ( 'NONE', *, *, #41875, .F. ) ;
#79827=ORIENTED_EDGE ( 'NONE', *, *, #25434, .F. ) ;
#79830=( BOUNDED_CURVE ( )  B_SPLINE_CURVE ( 3, ( #7989, #24227, #93094, #92539 ),
 .UNSPECIFIED., .F., .F. ) 
 B_SPLINE_CURVE_WITH_KNOTS ( ( 4, 4 ),
 ( 3.141592653589793116, 4.712388980384689674 ),
 .UNSPECIFIED. ) 
 CURVE ( )  GEOMETRIC_REPRESENTATION_ITEM ( )  RATIONAL_B_SPLINE_CURVE ( ( 1.000000000000000000, 0.8047378541243649375, 0.8047378541243649375, 1.000000000000000000 ) ) 
 REPRESENTATION_ITEM ( '' )  );
#79839=FACE_OUTER_BOUND ( 'NONE', #103967, .T. ) ;
#79841=CARTESIAN_POINT ( 'NONE',  ( 20.49599333844873783, 1525.960063244516959, 233.8638087104922931 ) ) ;
#79846=DIRECTION ( 'NONE',  ( 0.000000000000000000, -0.8286769424886156754, -0.5597271880011900347 ) ) ;
#79860=CARTESIAN_POINT ( 'NONE',  ( -29.73378234562438749, 1526.349684470114653, 217.2224020302186602 ) ) ;
#79864=CARTESIAN_POINT ( 'NONE',  ( 22.08622291487997558, 1523.456924617338700, 184.4183880513681402 ) ) ;
#79886=CARTESIAN_POINT ( 'NONE',  ( 2.314969334973908666, 1525.402221411349728, 243.6179210388352203 ) ) ;
#79889=CARTESIAN_POINT ( 'NONE',  ( -30.31940284292426924, 1523.456872492435195, 195.7503880523418616 ) ) ;
#79893=CARTESIAN_POINT ( 'NONE',  ( -2.311636021096358018, 1525.506916460682305, 241.8052139131910963 ) ) ;
#79901=CARTESIAN_POINT ( 'NONE',  ( 22.08622291482350519, 1518.913060387330006, 233.8253038720783366 ) ) ;
#79908=ORIENTED_EDGE ( 'NONE', *, *, #19333, .T. ) ;
#79946=AXIS2_PLACEMENT_3D ( 'NONE', #95850, #61187, #18021 ) ;
#79948=ORIENTED_EDGE ( 'NONE', *, *, #50184, .F. ) ;
#79957=DIRECTION ( 'NONE',  ( -0.000000000000000000, -1.000000000000000000, -0.000000000000000000 ) ) ;
#79963=DIRECTION ( 'NONE',  ( 0.000000000000000000, 1.000000000000000000, 0.000000000000000000 ) ) ;
#79965=AXIS2_PLACEMENT_3D ( 'NONE', #34387, #101560, #94846 ) ;
#79989=CARTESIAN_POINT ( 'NONE',  ( 3.261946504277382086, 1524.739563915922190, 241.7746690245087677 ) ) ;
#80028=CARTESIAN_POINT ( 'NONE',  ( 17.15830831501806131, 1512.187213306747481, 209.3391145445731070 ) ) ;
#80029=ORIENTED_EDGE ( 'NONE', *, *, #99903, .F. ) ;
#80033=LINE ( 'NONE', #36920, #105193 ) ;
#80037=CIRCLE ( 'NONE', #38857, 33.13701971169416538 ) ;
#80039=CARTESIAN_POINT ( 'NONE',  ( -31.23437356469425907, 1511.187213306747708, 222.8968241038848248 ) ) ;
#80051=CARTESIAN_POINT ( 'NONE',  ( 32.05521452193837462, 1525.253996226948402, 201.2193335479506118 ) ) ;
#80057=CARTESIAN_POINT ( 'NONE',  ( -2.143764089412641738, 1525.848198008145346, 176.8604052475766650 ) ) ;
#80059=CARTESIAN_POINT ( 'NONE',  ( 17.17241001986506888, 1512.187213306747481, 238.6251415217915337 ) ) ;
#80073=EDGE_CURVE ( 'NONE', #85994, #80823, #63068, .T. ) ;
#80085=EDGE_LOOP ( 'NONE', ( #1872, #30910, #78799, #58453 ) ) ;
#80091=AXIS2_PLACEMENT_3D ( 'NONE', #93565, #25806, #24694 ) ;
#80102=CARTESIAN_POINT ( 'NONE',  ( 2.456601303385831159, 1523.611961620354123, 175.3003469896238755 ) ) ;
#80120=DIRECTION ( 'NONE',  ( 0.000000000000000000, 0.07593562622321022026, -0.9971127221483482295 ) ) ;
#80124=( BOUNDED_SURFACE ( )  B_SPLINE_SURFACE ( 3, 2, ( 
 ( #55683, #66294, #32108 ),
 ( #64083, #13624, #21473 ),
 ( #100410, #98755, #38842 ),
 ( #14190, #14747, #56769 ),
 ( #5251, #83063, #30450 ),
 ( #64634, #23694, #48934 ),
 ( #72474, #57342, #73019 ),
 ( #47263, #108813, #22015 ),
 ( #73583, #65725, #81385 ),
 ( #56213, #91466, #108258 ),
 ( #31547, #22564, #39407 ),
 ( #57879, #15282, #6354 ),
 ( #90343, #74680, #89805 ),
 ( #38294, #106604, #92012 ) ),
 .UNSPECIFIED., .F., .F., .F. ) 
 B_SPLINE_SURFACE_WITH_KNOTS ( ( 4, 2, 2, 2, 2, 2, 4 ),
 ( 3, 3 ),
 ( 7.470152968425125550E-17, 0.0009443072508236408525, 0.001416460876235424091, 0.001888614501647207112, 0.002360768127058990133, 0.002832921752470773588, 0.003777229003294339631 ),
 ( 0.000000000000000000, 1.000000000000000000 ),
 .UNSPECIFIED. ) 
 GEOMETRIC_REPRESENTATION_ITEM ( )  RATIONAL_B_SPLINE_SURFACE ( (
 ( 1.000000000000000000, 0.9376006582765959996, 1.000000000000000000),
 ( 1.000000000000000000, 0.9283977714734229503, 1.000000000000000000),
 ( 1.000000000000000000, 0.9189750060483535821, 1.000000000000000000),
 ( 1.000000000000000000, 0.9042792056125676936, 1.000000000000000000),
 ( 1.000000000000000000, 0.8992469033842545034, 1.000000000000000000),
 ( 1.000000000000000000, 0.8891280264682865919, 1.000000000000000000),
 ( 1.000000000000000000, 0.8840337471676149583, 1.000000000000000000),
 ( 1.000000000000000000, 0.8736395124162725789, 1.000000000000000000),
 ( 1.000000000000000000, 0.8683406746555091260, 1.000000000000000000),
 ( 1.000000000000000000, 0.8573361860705441817, 1.000000000000000000),
 ( 1.000000000000000000, 0.8516508399497870752, 1.000000000000000000),
 ( 1.000000000000000000, 0.8340914917062759448, 1.000000000000000000),
 ( 1.000000000000000000, 0.8215597275864434668, 1.000000000000000000),
 ( 1.000000000000000000, 0.8070209408750140812, 1.000000000000000000) ) ) 
 REPRESENTATION_ITEM ( '' )  SURFACE ( )  );
#80127=ORIENTED_EDGE ( 'NONE', *, *, #25225, .F. ) ;
#80158=DIRECTION ( 'NONE',  ( 0.000000000000000000, 0.000000000000000000, 1.000000000000000000 ) ) ;
#80159=ORIENTED_EDGE ( 'NONE', *, *, #73472, .T. ) ;
#80160=DIRECTION ( 'NONE',  ( 0.3090169943749654369, 2.144236138472418401E-15, 0.9510565162951478690 ) ) ;
#80162=CARTESIAN_POINT ( 'NONE',  ( 33.43367350703735497, 1524.397344074318653, 197.7663411554291315 ) ) ;
#80169=VECTOR ( 'NONE', #104144, 1000.000000000000000 ) ;
#80172=CARTESIAN_POINT ( 'NONE',  ( 20.49599333844867033, 1525.960063244516959, 233.8638087104924068 ) ) ;
#80184=AXIS2_PLACEMENT_3D ( 'NONE', #93706, #68553, #16984 ) ;
#80186=CARTESIAN_POINT ( 'NONE',  ( 2.596261494520241353, 1525.907212628473644, 177.4701144822246874 ) ) ;
#80202=AXIS2_PLACEMENT_3D ( 'NONE', #91374, #108165, #93009 ) ;
#80208=ORIENTED_EDGE ( 'NONE', *, *, #105810, .F. ) ;
#80211=ORIENTED_EDGE ( 'NONE', *, *, #66546, .T. ) ;
#80228=CARTESIAN_POINT ( 'NONE',  ( -17.19739463999606599, 1525.960063244516959, 236.2603809477411971 ) ) ;
#80229=ORIENTED_EDGE ( 'NONE', *, *, #73495, .F. ) ;
#80230=ORIENTED_EDGE ( 'NONE', *, *, #42653, .F. ) ;
#80239=EDGE_CURVE ( 'NONE', #108592, #21237, #48438, .T. ) ;
#80247=ORIENTED_EDGE ( 'NONE', *, *, #90605, .T. ) ;
#80254=EDGE_CURVE ( 'NONE', #30516, #58921, #96098, .T. ) ;
#80269=CARTESIAN_POINT ( 'NONE',  ( -32.72607202732667275, 1524.152444737676660, 217.1332748866506108 ) ) ;
#80278=CARTESIAN_POINT ( 'NONE',  ( -16.58908872130532686, 1524.412455883367329, 237.5996433428405794 ) ) ;
#80280=CARTESIAN_POINT ( 'NONE',  ( 30.79916350760332833, 1526.104292489136469, 217.1177548920526306 ) ) ;
#80283=CARTESIAN_POINT ( 'NONE',  ( 16.89460221417492036, 1526.348417187221685, 183.3360764755736341 ) ) ;
#80298=CARTESIAN_POINT ( 'NONE',  ( -20.06031067115785760, 1526.189899547014420, 233.0619662239967340 ) ) ;
#80310=CARTESIAN_POINT ( 'NONE',  ( -33.34040796508471516, 1523.342713519623203, 196.1259889609353877 ) ) ;
#80339=CIRCLE ( 'NONE', #19490, 1.000000000000000888 ) ;
#80343=ORIENTED_EDGE ( 'NONE', *, *, #70675, .T. ) ;
#80345=DIRECTION ( 'NONE',  ( 0.000000000000000000, 0.000000000000000000, 1.000000000000000000 ) ) ;
#80356=DIRECTION ( 'NONE',  ( -0.000000000000000000, -1.000000000000000000, -0.000000000000000000 ) ) ;
#80361=CARTESIAN_POINT ( 'NONE',  ( -16.81049281788192218, 1526.143142182265819, 182.6472226615217380 ) ) ;
#80362=CARTESIAN_POINT ( 'NONE',  ( 21.83181799873717566, 1524.739563915921508, 233.6212106848500412 ) ) ;
#80403=AXIS2_PLACEMENT_3D ( 'NONE', #73854, #48659, #74414 ) ;
#80406=AXIS2_PLACEMENT_3D ( 'NONE', #53350, #3504, #10782 ) ;
#80412=FACE_OUTER_BOUND ( 'NONE', #21403, .T. ) ;
#80419=CIRCLE ( 'NONE', #64285, 1.000000000000000888 ) ;
#80440=CIRCLE ( 'NONE', #62573, 1.000000000000077494 ) ;
#80442=CARTESIAN_POINT ( 'NONE',  ( -3.237065521149570912, 1524.843416604498543, 241.7215981950958223 ) ) ;
#80454=AXIS2_PLACEMENT_3D ( 'NONE', #31282, #31834, #90631 ) ;
#80456=CARTESIAN_POINT ( 'NONE',  ( -16.50400130224731754, 1525.907212628473644, 236.2546788475584094 ) ) ;
#80473=CARTESIAN_POINT ( 'NONE',  ( 33.28034951413927445, 1522.382868172863937, 200.8029765415137717 ) ) ;
#80482=FACE_OUTER_BOUND ( 'NONE', #9725, .T. ) ;
#80488=CARTESIAN_POINT ( 'NONE',  ( -29.74901212038058418, 1525.343727714918259, 222.0046262735807829 ) ) ;
#80497=ORIENTED_EDGE ( 'NONE', *, *, #52118, .T. ) ;
#80499=DIRECTION ( 'NONE',  ( 0.9510565162951478690, 0.000000000000000000, -0.3090169943749654369 ) ) ;
#80506=ORIENTED_EDGE ( 'NONE', *, *, #11073, .F. ) ;
#80515=ORIENTED_EDGE ( 'NONE', *, *, #71499, .T. ) ;
#80522=EDGE_CURVE ( 'NONE', #42444, #88474, #5498, .T. ) ;
#80533=ORIENTED_EDGE ( 'NONE', *, *, #93180, .F. ) ;
#80561=CARTESIAN_POINT ( 'NONE',  ( -31.63976464710271941, 1525.343727714918259, 202.0582035741803679 ) ) ;
#80565=CARTESIAN_POINT ( 'NONE',  ( -2.390047989675008644, 1526.069472839384844, 240.5369618407216024 ) ) ;
#80568=CARTESIAN_POINT ( 'NONE',  ( -16.89460221416782915, 1526.348417187221685, 234.9076154478163687 ) ) ;
#80575=CARTESIAN_POINT ( 'NONE',  ( 32.06031249785753090, 1524.760046179776054, 216.1076607587503133 ) ) ;
#80591=AXIS2_PLACEMENT_3D ( 'NONE', #65416, #90586, #39072 ) ;
#80597=CARTESIAN_POINT ( 'NONE',  ( -31.44837959398574867, 1511.187213306747708, 220.9083067115980725 ) ) ;
#80608=CARTESIAN_POINT ( 'NONE',  ( 31.80535162409334049, 1525.137906803776559, 202.0924949887490243 ) ) ;
#80612=CARTESIAN_POINT ( 'NONE',  ( 3.232732302729357521, 1524.860077346004800, 176.5310237116080714 ) ) ;
#80616=CARTESIAN_POINT ( 'NONE',  ( 30.31118248177486052, 1526.186458717538926, 201.5497466985118820 ) ) ;
#80644=VECTOR ( 'NONE', #4913, 1000.000000000000000 ) ;
#80654=EDGE_LOOP ( 'NONE', ( #107772, #84218, #107864, #26807 ) ) ;
#80678=CARTESIAN_POINT ( 'NONE',  ( 21.83863730836016614, 1523.580203803270706, 183.2673815773253239 ) ) ;
#80685=TOROIDAL_SURFACE ( 'NONE', #12661, 2.000000000000000000, 1.000000000000000000 ) ;
#80686=CARTESIAN_POINT ( 'NONE',  ( 16.66231036550724198, 1523.604703353109699, 237.7554842931445478 ) ) ;
#80694=CARTESIAN_POINT ( 'NONE',  ( -22.75273496409559826, 1512.187213306747481, 234.5707981297189235 ) ) ;
#80697=CARTESIAN_POINT ( 'NONE',  ( -32.85805783624314813, 1523.678648413191695, 201.0453875934059340 ) ) ;
#80702=AXIS2_PLACEMENT_3D ( 'NONE', #98185, #47245, #13607 ) ;
#80725=CARTESIAN_POINT ( 'NONE',  ( -17.84054674790860773, 1523.580204110581235, 237.8810931398598143 ) ) ;
#80732=CARTESIAN_POINT ( 'NONE',  ( -2.470955850358427686, 1523.580204110584191, 175.3687159778811520 ) ) ;
#80741=LINE ( 'NONE', #106487, #33594 ) ;
#80746=DIRECTION ( 'NONE',  ( 0.000000000000000000, -1.000000000000000000, -0.000000000000000000 ) ) ;
#80750=FACE_OUTER_BOUND ( 'NONE', #56813, .T. ) ;
#80754=TOROIDAL_SURFACE ( 'NONE', #73653, 30.13701971169416538, 3.000000000000000000 ) ;
#80756=DIRECTION ( 'NONE',  ( 0.000000000000000000, 1.000000000000000000, 0.000000000000000000 ) ) ;
#80758=FACE_OUTER_BOUND ( 'NONE', #9331, .T. ) ;
#80761=VERTEX_POINT ( 'NONE', #67773 ) ;
#80779=ORIENTED_EDGE ( 'NONE', *, *, #92721, .F. ) ;
#80782=ORIENTED_EDGE ( 'NONE', *, *, #89359, .T. ) ;
#80799=VERTEX_POINT ( 'NONE', #110306 ) ;
#80803=CARTESIAN_POINT ( 'NONE',  ( -17.27380372710149103, 1525.712830164893376, 181.5601675622793039 ) ) ;
#80814=CARTESIAN_POINT ( 'NONE',  ( 20.71343476517513338, 1522.382868172863937, 179.9059455038194528 ) ) ;
#80821=CARTESIAN_POINT ( 'NONE',  ( 0.000000000000000000, 1511.187213306747708, 209.1218459616979999 ) ) ;
#80823=VERTEX_POINT ( 'NONE', #49866 ) ;
#80829=AXIS2_PLACEMENT_3D ( 'NONE', #10225, #9667, #43839 ) ;
#80838=EDGE_CURVE ( 'NONE', #35962, #79801, #58627, .T. ) ;
#80840=ADVANCED_FACE ( 'NONE', ( #33581 ), #41465, .F. ) ;
#80841=CARTESIAN_POINT ( 'NONE',  ( 3.350338079455601026, 1523.604703353109699, 176.1628856388066708 ) ) ;
#80870=CARTESIAN_POINT ( 'NONE',  ( 31.64580750758041461, 1523.313115944345327, 196.3083633854960794 ) ) ;
#80874=EDGE_CURVE ( 'NONE', #91565, #108700, #29605, .T. ) ;
#80878=DIRECTION ( 'NONE',  ( -0.9510565162951518658, 0.000000000000000000, 0.3090169943749528914 ) ) ;
#80903=CARTESIAN_POINT ( 'NONE',  ( 31.23437356469435144, 1512.187213306747481, 195.3468678195113739 ) ) ;
#80906=B_SPLINE_CURVE_WITH_KNOTS ( 'NONE', 3,
 ( #17862, #104101, #88408, #3332, #37456, #102978, #9486, #3878, #38007, #63776 ),
 .UNSPECIFIED., .F., .F.,
 ( 4, 2, 2, 2, 4 ),
 ( 0.000000000000000000, 0.0007189769279726045429, 0.001437953855945209086, 0.002156930783917813520, 0.002875907711890418172 ),
 .UNSPECIFIED. ) ;
#80910=CARTESIAN_POINT ( 'NONE',  ( 20.70484064406385727, 1525.907212628473872, 233.2025904124104443 ) ) ;
#80925=CARTESIAN_POINT ( 'NONE',  ( -29.35072644275227560, 1526.211528530236592, 220.5206086590065127 ) ) ;
#80933=CARTESIAN_POINT ( 'NONE',  ( 34.68852446352940433, 1501.977400791986611, 199.9946320047950223 ) ) ;
#80940=CARTESIAN_POINT ( 'NONE',  ( -30.77259778570326176, 1524.972383263453366, 221.6912870679553862 ) ) ;
#80946=EDGE_LOOP ( 'NONE', ( #7064, #79827, #21581, #102079 ) ) ;
#80957=CARTESIAN_POINT ( 'NONE',  ( 0.4151546846821903003, 1511.187213306747708, 243.9330574173806951 ) ) ;
#80959=ORIENTED_EDGE ( 'NONE', *, *, #106908, .T. ) ;
#80971=ADVANCED_FACE ( 'NONE', ( #21176 ), #39099, .T. ) ;
#80979=DIRECTION ( 'NONE',  ( 0.4090087482554204401, 2.838068309914575726E-15, 0.9125304618754019881 ) ) ;
#80983=CARTESIAN_POINT ( 'NONE',  ( -17.55396644409012907, 1524.816548299036640, 237.4834937945546187 ) ) ;
#80998=ORIENTED_EDGE ( 'NONE', *, *, #29636, .T. ) ;
#81009=DIRECTION ( 'NONE',  ( -0.000000000000000000, -1.000000000000000000, -0.000000000000000000 ) ) ;
#81012=EDGE_CURVE ( 'NONE', #49931, #64042, #71200, .T. ) ;
#81013=CARTESIAN_POINT ( 'NONE',  ( -21.41971086555122028, 1511.187213306747708, 185.1638823089581081 ) ) ;
#81018=VERTEX_POINT ( 'NONE', #107967 ) ;
#81031=VERTEX_POINT ( 'NONE', #83321 ) ;
#81049=VERTEX_POINT ( 'NONE', #49192 ) ;
#81063=ORIENTED_EDGE ( 'NONE', *, *, #27517, .T. ) ;
#81075=DIRECTION ( 'NONE',  ( -0.000000000000000000, -1.000000000000000000, -0.000000000000000000 ) ) ;
#81076=CARTESIAN_POINT ( 'NONE',  ( 31.34137657934018506, 1523.382868172864164, 221.9025654077410081 ) ) ;
#81080=ORIENTED_EDGE ( 'NONE', *, *, #9797, .T. ) ;
#81095=CARTESIAN_POINT ( 'NONE',  ( -32.31946296792706619, 1524.082582765195411, 202.1440730665343324 ) ) ;
#81100=FACE_OUTER_BOUND ( 'NONE', #7234, .T. ) ;
#81121=LINE ( 'NONE', #30161, #76564 ) ;
#81134=ORIENTED_EDGE ( 'NONE', *, *, #19899, .F. ) ;
#81135=ORIENTED_EDGE ( 'NONE', *, *, #50041, .F. ) ;
#81137=CARTESIAN_POINT ( 'NONE',  ( 18.40343465886353513, 1525.402221411349501, 238.3904617729369306 ) ) ;
#81149=CARTESIAN_POINT ( 'NONE',  ( 3.350338079455601026, 1523.604703353109699, 176.1628856388066708 ) ) ;
#81171=DIRECTION ( 'NONE',  ( 0.000000000000000000, 0.000000000000000000, 1.000000000000000000 ) ) ;
#81191=CARTESIAN_POINT ( 'NONE',  ( 2.314969334973882464, 1525.402221411349956, 174.6257708845645595 ) ) ;
#81202=CARTESIAN_POINT ( 'NONE',  ( 29.86461515634905695, 1525.960063244517187, 197.2746849027936378 ) ) ;
#81209=AXIS2_PLACEMENT_3D ( 'NONE', #80039, #44803, #105808 ) ;
#81214=DIRECTION ( 'NONE',  ( -0.000000000000000000, -1.000000000000000000, 0.000000000000000000 ) ) ;
#81227=CARTESIAN_POINT ( 'NONE',  ( -19.63708787179571402, 1526.382868172863937, 234.8228066531185334 ) ) ;
#81241=CARTESIAN_POINT ( 'NONE',  ( 17.89234610336922771, 1523.611961620354123, 180.3157245011607017 ) ) ;
#81246=CARTESIAN_POINT ( 'NONE',  ( 18.86688640473582268, 1512.187213306747481, 180.7825021045438803 ) ) ;
#81261=CARTESIAN_POINT ( 'NONE',  ( 2.038646110889573038, 1525.960063244516959, 177.0579350083065435 ) ) ;
#81284=VERTEX_POINT ( 'NONE', #91596 ) ;
#81290=VERTEX_POINT ( 'NONE', #90486 ) ;
#81312=CARTESIAN_POINT ( 'NONE',  ( 31.93049531883788816, 1525.394081235439444, 217.0185068061728941 ) ) ;
#81327=ORIENTED_EDGE ( 'NONE', *, *, #68470, .F. ) ;
#81328=CARTESIAN_POINT ( 'NONE',  ( -17.37724426307464753, 1525.394057003702756, 181.1943177926724502 ) ) ;
#81347=CARTESIAN_POINT ( 'NONE',  ( 29.30029655192936033, 1525.907212628473644, 221.3719603026171967 ) ) ;
#81356=B_SPLINE_CURVE_WITH_KNOTS ( 'NONE', 3,
 ( #40634, #23814, #7032, #75362, #25464, #23269, #83737, #76441, #33880, #24904 ),
 .UNSPECIFIED., .F., .F.,
 ( 4, 2, 2, 2, 4 ),
 ( 0.000000000000000000, 0.0007189769279725903399, 0.001437953855945180680, 0.002156930783917771020, 0.002875907711890361360 ),
 .UNSPECIFIED. ) ;
#81357=CIRCLE ( 'NONE', #109994, 2.000000000000001776 ) ;
#81361=DIRECTION ( 'NONE',  ( -0.8090169943749467851, 5.613683090426285025E-15, -0.5877852522924740253 ) ) ;
#81365=AXIS2_PLACEMENT_3D ( 'NONE', #48215, #109220, #14024 ) ;
#81379=DIRECTION ( 'NONE',  ( -0.000000000000000000, -1.000000000000000000, -0.000000000000000000 ) ) ;
#81380=CARTESIAN_POINT ( 'NONE',  ( 0.000000000000000000, 1524.340287715038357, 209.1218459616979999 ) ) ;
#81381=DIRECTION ( 'NONE',  ( -0.9125304618754029873, 0.000000000000000000, -0.4090087482554177756 ) ) ;
#81385=CARTESIAN_POINT ( 'NONE',  ( 32.35368859299575206, 1524.871836253796118, 217.0491380271198807 ) ) ;
#81408=ORIENTED_EDGE ( 'NONE', *, *, #55623, .T. ) ;
#81412=DIRECTION ( 'NONE',  ( 0.000000000000000000, 1.000000000000000000, 0.000000000000000000 ) ) ;
#81416=( BOUNDED_SURFACE ( )  B_SPLINE_SURFACE ( 3, 2, ( 
 ( #62704, #53169, #88410 ),
 ( #80565, #45876, #106310 ),
 ( #20624, #78356, #27953 ),
 ( #95707, #70539, #44213 ),
 ( #29594, #87880, #45330 ),
 ( #87311, #1665, #37458 ) ),
 .UNSPECIFIED., .F., .F., .F. ) 
 B_SPLINE_SURFACE_WITH_KNOTS ( ( 4, 2, 4 ),
 ( 3, 3 ),
 ( -5.095750210681870840E-17, 0.001312027981647294166, 0.002624055963294639506 ),
 ( 0.000000000000000000, 1.000000000000000000 ),
 .UNSPECIFIED. ) 
 GEOMETRIC_REPRESENTATION_ITEM ( )  RATIONAL_B_SPLINE_SURFACE ( (
 ( 1.000000000000000000, 0.9376006582765910036, 1.000000000000000000),
 ( 1.000000000000000000, 0.9569320108024047533, 1.000000000000000000),
 ( 1.000000000000000000, 0.9725743441616951923, 1.000000000000000000),
 ( 1.000000000000000000, 0.9942095667137571535, 1.000000000000000000),
 ( 1.000000000000000000, 1.000043666450562752, 1.000000000000000000),
 ( 1.000000000000000000, 1.000000000000000000, 1.000000000000000000) ) ) 
 REPRESENTATION_ITEM ( '' )  SURFACE ( )  );
#81419=CARTESIAN_POINT ( 'NONE',  ( -30.31052258194605642, 1523.604703353109699, 195.7506062427372058 ) ) ;
#81436=CARTESIAN_POINT ( 'NONE',  ( -22.75273496409615603, 1511.187213306747708, 183.6728937936775310 ) ) ;
#81438=VERTEX_POINT ( 'NONE', #31681 ) ;
#81444=EDGE_CURVE ( 'NONE', #59426, #48271, #17497, .T. ) ;
#81473=ORIENTED_EDGE ( 'NONE', *, *, #107044, .F. ) ;
#81506=EDGE_LOOP ( 'NONE', ( #38213, #65107, #69632, #44292 ) ) ;
#81528=EDGE_LOOP ( 'NONE', ( #103176, #68004, #58863, #29525, #56619 ) ) ;
#81535=DIRECTION ( 'NONE',  ( 0.4090087482554383147, 0.000000000000000000, 0.9125304618753937724 ) ) ;
#81541=EDGE_CURVE ( 'NONE', #33454, #54701, #105581, .T. ) ;
#81547=CARTESIAN_POINT ( 'NONE',  ( 33.23421991949613385, 1522.906363951597314, 200.8294566360694660 ) ) ;
#81548=AXIS2_PLACEMENT_3D ( 'NONE', #96248, #7142, #82746 ) ;
#81551=VERTEX_POINT ( 'NONE', #22429 ) ;
#81558=ADVANCED_FACE ( 'NONE', ( #56631 ), #74915, .T. ) ;
#81579=EDGE_CURVE ( 'NONE', #97968, #101207, #53774, .T. ) ;
#81584=CARTESIAN_POINT ( 'NONE',  ( -17.30126322264655769, 1523.462669333492613, 180.8506073315049605 ) ) ;
#81588=EDGE_LOOP ( 'NONE', ( #66842, #75144, #62777, #55841 ) ) ;
#81606=EDGE_LOOP ( 'NONE', ( #85202, #77686, #5004, #64607 ) ) ;
#81614=CARTESIAN_POINT ( 'NONE',  ( 32.23393008313274066, 1523.382868172864391, 201.4036600223104756 ) ) ;
#81615=ADVANCED_FACE ( 'NONE', ( #90632 ), #13910, .T. ) ;
#81616=DIRECTION ( 'NONE',  ( -0.3090169943749382919, 0.000000000000000000, 0.9510565162951565288 ) ) ;
#81636=ORIENTED_EDGE ( 'NONE', *, *, #6329, .F. ) ;
#81656=EDGE_LOOP ( 'NONE', ( #50097, #4169, #13544, #64242, #42933, #41009, #29148, #55690 ) ) ;
#81664=CARTESIAN_POINT ( 'NONE',  ( 1.336801414591168413, 1526.382868172864164, 178.6745493585861482 ) ) ;
#81669=CARTESIAN_POINT ( 'NONE',  ( 20.20959865099471031, 1512.187213306747481, 182.0120230947219966 ) ) ;
#81673=EDGE_LOOP ( 'NONE', ( #35264, #97438, #81473, #29614 ) ) ;
#81675=CARTESIAN_POINT ( 'NONE',  ( 20.17436656406300699, 1524.841055067849766, 237.7389007707603241 ) ) ;
#81678=EDGE_CURVE ( 'NONE', #83932, #64568, #66021, .T. ) ;
#81679=CARTESIAN_POINT ( 'NONE',  ( 22.75273496409577945, 1512.187213306747481, 183.6728937936772184 ) ) ;
#81688=CARTESIAN_POINT ( 'NONE',  ( 3.141363374988426660, 1525.159177407155767, 176.7077309898103010 ) ) ;
#81693=CIRCLE ( 'NONE', #108565, 2.000000000000001776 ) ;
#81710=DIRECTION ( 'NONE',  ( 0.000000000000000000, 1.000000000000000000, 0.000000000000000000 ) ) ;
#81719=CIRCLE ( 'NONE', #53147, 33.13701971169416538 ) ;
#81770=CARTESIAN_POINT ( 'NONE',  ( -30.31940284292398857, 1523.382868172864164, 222.4933038710547919 ) ) ;
#81773=CARTESIAN_POINT ( 'NONE',  ( -22.52214966618477376, 1524.244163922423695, 236.5012798002454701 ) ) ;
#81801=AXIS2_PLACEMENT_3D ( 'NONE', #83517, #33117, #101400 ) ;
#81809=CARTESIAN_POINT ( 'NONE',  ( 16.53242905777655025, 1526.073429442291854, 182.3092717672457184 ) ) ;
#81810=CARTESIAN_POINT ( 'NONE',  ( 1.590879946460525218, 1526.333389947941669, 178.3980910637225463 ) ) ;
#81818=CARTESIAN_POINT ( 'NONE',  ( 2.038847259689231084, 1522.382868172863937, 173.3106345060153046 ) ) ;
#81825=CARTESIAN_POINT ( 'NONE',  ( 0.4151546846821903003, 1501.977400791986611, 244.9330574173806951 ) ) ;
#81828=CARTESIAN_POINT ( 'NONE',  ( 16.71509328322861521, 1526.382868172863937, 234.3620852791651146 ) ) ;
#81838=ORIENTED_EDGE ( 'NONE', *, *, #39427, .T. ) ;
#81839=ORIENTED_EDGE ( 'NONE', *, *, #57111, .T. ) ;
#81842=AXIS2_PLACEMENT_3D ( 'NONE', #14071, #90228, #41912 ) ;
#81858=ORIENTED_EDGE ( 'NONE', *, *, #12447, .F. ) ;
#81876=EDGE_LOOP ( 'NONE', ( #78886, #75905, #14929 ) ) ;
#81879=ORIENTED_EDGE ( 'NONE', *, *, #21247, .T. ) ;
#81903=DIRECTION ( 'NONE',  ( 8.881784197001252323E-15, 0.000000000000000000, 1.000000000000000000 ) ) ;
#81918=EDGE_LOOP ( 'NONE', ( #64684, #39595, #11182 ) ) ;
#81922=CARTESIAN_POINT ( 'NONE',  ( -32.86802468363524099, 1523.481610118014487, 217.2040256692613980 ) ) ;
#81925=CIRCLE ( 'NONE', #89130, 0.9999999999999970024 ) ;
#81956=FACE_OUTER_BOUND ( 'NONE', #39828, .T. ) ;
#81979=CARTESIAN_POINT ( 'NONE',  ( -33.28034951413935971, 1522.382868172863937, 200.8029765415142549 ) ) ;
#81986=VERTEX_POINT ( 'NONE', #81013 ) ;
#81987=CARTESIAN_POINT ( 'NONE',  ( -16.89460221417084895, 1526.348417187220775, 183.3360764755740604 ) ) ;
#81988=CARTESIAN_POINT ( 'NONE',  ( 21.80586122363390800, 1523.954914175592421, 234.9031843411586635 ) ) ;
#81995=CARTESIAN_POINT ( 'NONE',  ( -28.27139721233049485, 1526.382868172864164, 198.6830693683576499 ) ) ;
#81998=AXIS2_PLACEMENT_3D ( 'NONE', #64364, #64916, #55955 ) ;
#82019=VECTOR ( 'NONE', #72661, 1000.000000000000000 ) ;
#82024=CARTESIAN_POINT ( 'NONE',  ( 29.36007807473302123, 1526.208281990539263, 197.7147929784462121 ) ) ;
#82029=CARTESIAN_POINT ( 'NONE',  ( -0.4151546846821903003, 1511.187213306747708, 174.3106345060153046 ) ) ;
#82037=CARTESIAN_POINT ( 'NONE',  ( -30.44527832718667071, 1526.211523310372058, 217.1519757128520212 ) ) ;
#82044=CARTESIAN_POINT ( 'NONE',  ( -3.347801439296144377, 1523.456872492435195, 176.1543725841967500 ) ) ;
#82045=VERTEX_POINT ( 'NONE', #13232 ) ;
#82049=AXIS2_PLACEMENT_3D ( 'NONE', #49326, #50979, #60492 ) ;
#82050=CARTESIAN_POINT ( 'NONE',  ( 16.73628186595838940, 1526.382868172863937, 234.1845039693043589 ) ) ;
#82055=AXIS2_PLACEMENT_3D ( 'NONE', #49348, #6768, #106490 ) ;
#82074=DIRECTION ( 'NONE',  ( 0.000000000000000000, -1.000000000000000000, 0.000000000000000000 ) ) ;
#82075=DIRECTION ( 'NONE',  ( 0.000000000000000000, 1.000000000000000000, 0.000000000000000000 ) ) ;
#82076=AXIS2_PLACEMENT_3D ( 'NONE', #44755, #20603, #27374 ) ;
#82080=EDGE_CURVE ( 'NONE', #105138, #102452, #41518, .T. ) ;
#82101=AXIS2_PLACEMENT_3D ( 'NONE', #812, #24321, #60733 ) ;
#82105=CARTESIAN_POINT ( 'NONE',  ( -20.06033034266364368, 1526.189892541618974, 185.1817216005363491 ) ) ;
#82111=ORIENTED_EDGE ( 'NONE', *, *, #60512, .F. ) ;
#82128=ORIENTED_EDGE ( 'NONE', *, *, #23951, .T. ) ;
#82132=DIRECTION ( 'NONE',  ( 0.000000000000000000, 0.000000000000000000, 1.000000000000000000 ) ) ;
#82134=AXIS2_PLACEMENT_3D ( 'NONE', #101018, #24316, #89204 ) ;
#82142=DIRECTION ( 'NONE',  ( -0.4978433412588781914, 0.000000000000000000, -0.8672669759446606230 ) ) ;
#82145=CARTESIAN_POINT ( 'NONE',  ( -17.84054674790984052, 1523.580204110583281, 180.3625987835359581 ) ) ;
#82148=ORIENTED_EDGE ( 'NONE', *, *, #76837, .F. ) ;
#82149=ORIENTED_EDGE ( 'NONE', *, *, #8708, .T. ) ;
#82151=CARTESIAN_POINT ( 'NONE',  ( 17.17241001986506888, 1518.913060387330006, 237.6251415217915337 ) ) ;
#82159=DIRECTION ( 'NONE',  ( 0.000000000000000000, 0.000000000000000000, 1.000000000000000000 ) ) ;
#82182=ORIENTED_EDGE ( 'NONE', *, *, #17853, .F. ) ;
#82185=DIRECTION ( 'NONE',  ( 0.07713599384728295205, -0.9969860201949398704, 0.008301444997532481801 ) ) ;
#82198=CARTESIAN_POINT ( 'NONE',  ( 2.038847259689231084, 1501.977400791986611, 173.3106345060153046 ) ) ;
#82206=EDGE_CURVE ( 'NONE', #83491, #9501, #90899, .T. ) ;
#82212=EDGE_CURVE ( 'NONE', #71731, #41473, #27719, .T. ) ;
#82216=AXIS2_PLACEMENT_3D ( 'NONE', #14845, #108922, #22122 ) ;
#82223=EDGE_LOOP ( 'NONE', ( #26335, #94532, #82149 ) ) ;
#82225=PRODUCT ( 'Threaded Lock Nut', 'Threaded Lock Nut', '', ( #48282 ) ) ;
#82226=( BOUNDED_SURFACE ( )  B_SPLINE_SURFACE ( 3, 2, ( 
 ( #4213, #38343, #5302 ),
 ( #104593, #107763, #73070 ),
 ( #27888, #22615, #53671 ),
 ( #98806, #11101, #78857 ),
 ( #22067, #55736, #56264 ),
 ( #13671, #2166, #81995 ) ),
 .UNSPECIFIED., .F., .F., .T. ) 
 B_SPLINE_SURFACE_WITH_KNOTS ( ( 4, 2, 4 ),
 ( 3, 3 ),
 ( 5.009014036883030485E-17, 0.001312027981647231282, 0.002624055963294412257 ),
 ( 0.000000000000000000, 1.000000000000000000 ),
 .UNSPECIFIED. ) 
 GEOMETRIC_REPRESENTATION_ITEM ( )  RATIONAL_B_SPLINE_SURFACE ( (
 ( 1.000000000000000000, 0.9376006582765964437, 1.000000000000000000),
 ( 1.000000000000000000, 0.9569320108028295246, 1.000000000000000000),
 ( 1.000000000000000000, 0.9725743441611425233, 1.000000000000000000),
 ( 1.000000000000000000, 0.9942095667143253657, 1.000000000000000000),
 ( 1.000000000000000000, 1.000043666450136204, 1.000000000000000000),
 ( 1.000000000000000000, 1.000000000000000000, 1.000000000000000000) ) ) 
 REPRESENTATION_ITEM ( '' )  SURFACE ( )  );
#82241=CIRCLE ( 'NONE', #57261, 1.000000000000000888 ) ;
#82243=ORIENTED_EDGE ( 'NONE', *, *, #76153, .T. ) ;
#82245=CARTESIAN_POINT ( 'NONE',  ( 20.71343476517535009, 1522.382868172863937, 238.3377464195763764 ) ) ;
#82249=PLANE ( 'NONE',  #100146 ) ;
#82258=DIRECTION ( 'NONE',  ( 0.4978433412588651463, 0.000000000000000000, -0.8672669759446679505 ) ) ;
#82264=CYLINDRICAL_SURFACE ( 'NONE', #14042, 2.000000000000003109 ) ;
#82268=EDGE_CURVE ( 'NONE', #31591, #23879, #65913, .T. ) ;
#82281=CARTESIAN_POINT ( 'NONE',  ( -32.78250617288050961, 1512.187213306747481, 199.9357095655695957 ) ) ;
#82282=FACE_OUTER_BOUND ( 'NONE', #11591, .T. ) ;
#82301=EDGE_LOOP ( 'NONE', ( #84434, #63731, #19610, #11940 ) ) ;
#82308=CARTESIAN_POINT ( 'NONE',  ( -30.60906614450610874, 1526.073434386619510, 216.5595830063403753 ) ) ;
#82316=CARTESIAN_POINT ( 'NONE',  ( 29.30029655192925730, 1525.907212628473872, 196.8717316207785757 ) ) ;
#82322=VERTEX_POINT ( 'NONE', #25355 ) ;
#82323=CARTESIAN_POINT ( 'NONE',  ( -16.16632277704817611, 1511.187213306747708, 181.3470724465437627 ) ) ;
#82332=CARTESIAN_POINT ( 'NONE',  ( 16.54106930751544269, 1524.860077346004800, 237.3885273948277188 ) ) ;
#82340=CARTESIAN_POINT ( 'NONE',  ( 29.00779973304137371, 1526.382868172863937, 217.2942086403122914 ) ) ;
#82343=CARTESIAN_POINT ( 'NONE',  ( -31.34491295179425663, 1525.848198008145346, 201.1913533246503789 ) ) ;
#82345=DIRECTION ( 'NONE',  ( 0.000000000000000000, 0.000000000000000000, 1.000000000000000000 ) ) ;
#82350=FACE_OUTER_BOUND ( 'NONE', #46468, .T. ) ;
#82353=EDGE_CURVE ( 'NONE', #20210, #72801, #8643, .T. ) ;
#82359=AXIS2_PLACEMENT_3D ( 'NONE', #8211, #76532, #53570 ) ;
#82365=VERTEX_POINT ( 'NONE', #79117 ) ;
#82366=CARTESIAN_POINT ( 'NONE',  ( -17.24701803732119743, 1523.844789899205125, 180.8504343893186501 ) ) ;
#82375=CARTESIAN_POINT ( 'NONE',  ( 18.66420869458052323, 1526.382868172864164, 232.7837831374276902 ) ) ;
#82378=CARTESIAN_POINT ( 'NONE',  ( -17.43739734485555459, 1526.178928173328131, 237.5162751070486422 ) ) ;
#82381=ADVANCED_FACE ( 'NONE', ( #88069 ), #31298, .F. ) ;
#82391=AXIS2_PLACEMENT_3D ( 'NONE', #40124, #13802, #38472 ) ;
#82407=FACE_OUTER_BOUND ( 'NONE', #91636, .T. ) ;
#82409=EDGE_CURVE ( 'NONE', #107214, #83466, #68253, .T. ) ;
#82410=CIRCLE ( 'NONE', #16265, 0.9999999999999481526 ) ;
#82411=CARTESIAN_POINT ( 'NONE',  ( -32.31945039880162085, 1524.082740465118604, 216.0996078590375475 ) ) ;
#82417=ORIENTED_EDGE ( 'NONE', *, *, #67354, .T. ) ;
#82418=DIRECTION ( 'NONE',  ( -0.9125304618754022101, 0.000000000000000000, -0.4090087482554195519 ) ) ;
#82442=CARTESIAN_POINT ( 'NONE',  ( 29.52630424919045637, 1525.661275128776197, 221.7199234082868884 ) ) ;
#82449=ORIENTED_EDGE ( 'NONE', *, *, #57709, .T. ) ;
#82473=CARTESIAN_POINT ( 'NONE',  ( -0.4151546846821903003, 1511.187213306747708, 243.9330574173806951 ) ) ;
#82503=EDGE_CURVE ( 'NONE', #40664, #23280, #78442, .T. ) ;
#82513=DIRECTION ( 'NONE',  ( 0.000000000000000000, 0.000000000000000000, 1.000000000000000000 ) ) ;
#82520=CARTESIAN_POINT ( 'NONE',  ( -20.39893125377176730, 1526.069472839383252, 185.1113182959119001 ) ) ;
#82532=CARTESIAN_POINT ( 'NONE',  ( 16.48400375141593344, 1525.790287071782359, 236.4799654700566975 ) ) ;
#82555=CARTESIAN_POINT ( 'NONE',  ( 32.86802468386284914, 1501.977400791986611, 201.0396662540042030 ) ) ;
#82556=EDGE_CURVE ( 'NONE', #47989, #39456, #78841, .T. ) ;
#82569=VERTEX_POINT ( 'NONE', #45253 ) ;
#82570=DIRECTION ( 'NONE',  ( -0.000000000000000000, -1.000000000000000000, -0.000000000000000000 ) ) ;
#82581=VERTEX_POINT ( 'NONE', #79388 ) ;
#82587=ORIENTED_EDGE ( 'NONE', *, *, #43482, .T. ) ;
#82596=DIRECTION ( 'NONE',  ( 0.4090087482554183862, 0.000000000000000000, -0.9125304618754026542 ) ) ;
#82606=AXIS2_PLACEMENT_3D ( 'NONE', #60890, #68731, #59771 ) ;
#82612=DIRECTION ( 'NONE',  ( -1.000000000000000000, 0.000000000000000000, 0.000000000000000000 ) ) ;
#82616=CARTESIAN_POINT ( 'NONE',  ( 31.69312280309836183, 1525.713797967456685, 221.9404206525572931 ) ) ;
#82621=AXIS2_PLACEMENT_3D ( 'NONE', #70141, #68466, #59508 ) ;
#82629=CARTESIAN_POINT ( 'NONE',  ( 31.81407709660769001, 1501.977400791986611, 196.2902540610627682 ) ) ;
#82646=DIRECTION ( 'NONE',  ( 0.000000000000000000, 0.000000000000000000, -1.000000000000000000 ) ) ;
#82659=DIRECTION ( 'NONE',  ( -0.9942586961433756976, -0.000000000000000000, -0.1070030146457317671 ) ) ;
#82684=CARTESIAN_POINT ( 'NONE',  ( -2.470955845399089856, 1523.580203803270933, 175.3687159542604377 ) ) ;
#82691=VERTEX_POINT ( 'NONE', #107200 ) ;
#82698=AXIS2_PLACEMENT_3D ( 'NONE', #76672, #26255, #42513 ) ;
#82700=ORIENTED_EDGE ( 'NONE', *, *, #32223, .T. ) ;
#82703=DIRECTION ( 'NONE',  ( -0.9786619618251632957, 0.000000000000000000, 0.2054769195713296581 ) ) ;
#82706=CARTESIAN_POINT ( 'NONE',  ( -17.84338787552430006, 1523.481610118012895, 180.3600277898067930 ) ) ;
#82712=CARTESIAN_POINT ( 'NONE',  ( -29.61692403810246077, 1526.104292489126692, 220.7563138442914408 ) ) ;
#82715=DIRECTION ( 'NONE',  ( 0.4090087482554363163, 0.000000000000000000, 0.9125304618753946606 ) ) ;
#82718=CARTESIAN_POINT ( 'NONE',  ( 31.23437356469435144, 1512.187213306747481, 195.3468678195113739 ) ) ;
#82746=DIRECTION ( 'NONE',  ( 0.9510565162951561957, 0.000000000000000000, 0.3090169943749392911 ) ) ;
#82749=CARTESIAN_POINT ( 'NONE',  ( -0.5890887500919901321, 1526.382868172863937, 174.9674887555077021 ) ) ;
#82772=DIRECTION ( 'NONE',  ( -0.000000000000000000, -1.000000000000000000, -0.000000000000000000 ) ) ;
#82773=EDGE_LOOP ( 'NONE', ( #79569, #37576, #22672 ) ) ;
#82791=CARTESIAN_POINT ( 'NONE',  ( 18.02257621027597523, 1526.382868172863937, 235.3484976865586873 ) ) ;
#82794=CARTESIAN_POINT ( 'NONE',  ( -21.44520247467892204, 1525.343727714918259, 184.8098521824372540 ) ) ;
#82798=CARTESIAN_POINT ( 'NONE',  ( -33.42844755917176514, 1522.382868172863937, 222.1271778627170761 ) ) ;
#82823=DIRECTION ( 'NONE',  ( 0.4978433412588624818, 0.000000000000000000, -0.8672669759446693938 ) ) ;
#82828=ORIENTED_EDGE ( 'NONE', *, *, #48129, .F. ) ;
#82849=EDGE_LOOP ( 'NONE', ( #36836, #98509, #8660, #25381 ) ) ;
#82852=CARTESIAN_POINT ( 'NONE',  ( 17.12015336051587511, 1526.107876515966382, 235.9348256314145829 ) ) ;
#82881=( BOUNDED_SURFACE ( )  B_SPLINE_SURFACE ( 3, 2, ( 
 ( #14242, #79402, #29942 ),
 ( #48431, #72522, #94900 ),
 ( #102181, #3483, #42845 ),
 ( #19699, #63401, #34985 ),
 ( #69165, #11321, #9246 ),
 ( #62868, #12399, #77007 ),
 ( #80162, #68613, #313 ),
 ( #53902, #68069, #37054 ),
 ( #85945, #25461, #26578 ),
 ( #28663, #2937, #79633 ) ),
 .UNSPECIFIED., .F., .F., .F. ) 
 B_SPLINE_SURFACE_WITH_KNOTS ( ( 4, 2, 2, 2, 4 ),
 ( 3, 3 ),
 ( 1.570796326794896558, 1.963495408493620697, 2.356194490192344837, 2.748893571891068976, 3.141592653589793116 ),
 ( 0.000000000000000000, 1.000000000000000000 ),
 .UNSPECIFIED. ) 
 GEOMETRIC_REPRESENTATION_ITEM ( )  RATIONAL_B_SPLINE_SURFACE ( (
 ( 1.000000000000000000, 0.7071067811865869857, 1.000000000000000000),
 ( 1.000000000000000000, 0.7166207884823135865, 1.000000000000000000),
 ( 1.000000000000000000, 0.7259222650905752250, 1.000000000000000000),
 ( 1.000000000000000000, 0.7428408967931670048, 1.000000000000000000),
 ( 1.000000000000000000, 0.7504512394537760089, 1.000000000000000000),
 ( 1.000000000000000000, 0.7630177051937124810, 1.000000000000000000),
 ( 1.000000000000000000, 0.7679730451971344962, 1.000000000000000000),
 ( 1.000000000000000000, 0.7746454561798989946, 1.000000000000000000),
 ( 1.000000000000000000, 0.7763684247033887376, 1.000000000000000000),
 ( 1.000000000000000000, 0.7763623250684346111, 1.000000000000000000) ) ) 
 REPRESENTATION_ITEM ( '' )  SURFACE ( )  );
#82886=CIRCLE ( 'NONE', #47183, 1.000000000000000888 ) ;
#82887=FACE_OUTER_BOUND ( 'NONE', #44436, .T. ) ;
#82889=CARTESIAN_POINT ( 'NONE',  ( 31.23437356469435144, 1511.187213306747708, 197.3468678195113739 ) ) ;
#82893=CARTESIAN_POINT ( 'NONE',  ( 21.32681782946750104, 1525.211473355384669, 183.8595827939377898 ) ) ;
#82912=CARTESIAN_POINT ( 'NONE',  ( 17.84338787571943641, 1501.977400791986611, 237.8836641337660467 ) ) ;
#82916=CARTESIAN_POINT ( 'NONE',  ( -21.83550407203936672, 1523.678648413191695, 183.2743720722710634 ) ) ;
#82918=CARTESIAN_POINT ( 'NONE',  ( -16.68062049856681739, 1524.382868172863937, 236.8314524626098319 ) ) ;
#82925=ORIENTED_EDGE ( 'NONE', *, *, #102669, .T. ) ;
#82926=DIRECTION ( 'NONE',  ( 0.5032920991127231014, -0.8641163480519905571, 0.000000000000000000 ) ) ;
#82945=EDGE_CURVE ( 'NONE', #6825, #32838, #40862, .T. ) ;
#82949=VERTEX_POINT ( 'NONE', #40407 ) ;
#82995=ORIENTED_EDGE ( 'NONE', *, *, #21247, .F. ) ;
#83003=CARTESIAN_POINT ( 'NONE',  ( 29.79881796581619113, 1526.748660780343471, 196.6633055964653352 ) ) ;
#83004=CARTESIAN_POINT ( 'NONE',  ( -21.84020450222076803, 1512.187213306747481, 183.2638850454220858 ) ) ;
#83020=ORIENTED_EDGE ( 'NONE', *, *, #41288, .T. ) ;
#83038=CARTESIAN_POINT ( 'NONE',  ( 31.81407709660777527, 1512.187213306747481, 221.9534378623329758 ) ) ;
#83063=CARTESIAN_POINT ( 'NONE',  ( 31.62137330307827909, 1525.231909165033585, 216.6630335337264626 ) ) ;
#83065=( BOUNDED_SURFACE ( )  B_SPLINE_SURFACE ( 3, 2, ( 
 ( #100569, #84325, #85409 ),
 ( #15450, #66997, #93805 ),
 ( #42325, #75401, #108990 ),
 ( #102223, #23307, #75928 ),
 ( #59693, #42887, #58590 ),
 ( #76479, #74846, #77045 ) ),
 .UNSPECIFIED., .F., .F., .F. ) 
 B_SPLINE_SURFACE_WITH_KNOTS ( ( 4, 2, 4 ),
 ( 3, 3 ),
 ( -2.732189474663471174E-17, 0.001312027981647287444, 0.002624055963294602209 ),
 ( 0.000000000000000000, 1.000000000000000000 ),
 .UNSPECIFIED. ) 
 GEOMETRIC_REPRESENTATION_ITEM ( )  RATIONAL_B_SPLINE_SURFACE ( (
 ( 1.000000000000000000, 0.9376006582765910036, 1.000000000000000000),
 ( 1.000000000000000000, 0.9569320108028100957, 1.000000000000000000),
 ( 1.000000000000000000, 0.9725743441611582885, 1.000000000000000000),
 ( 1.000000000000000000, 0.9942095667142945015, 1.000000000000000000),
 ( 1.000000000000000000, 1.000043666450159296, 1.000000000000000000),
 ( 1.000000000000000000, 1.000000000000000000, 1.000000000000000000) ) ) 
 REPRESENTATION_ITEM ( '' )  SURFACE ( )  );
#83069=ORIENTED_EDGE ( 'NONE', *, *, #70651, .T. ) ;
#83076=CARTESIAN_POINT ( 'NONE',  ( 16.86500409604441231, 1525.697947650497099, 236.3931732427541874 ) ) ;
#83100=( BOUNDED_SURFACE ( )  B_SPLINE_SURFACE ( 3, 2, ( 
 ( #27263, #103393, #84942 ),
 ( #103966, #76556, #110711 ),
 ( #102299, #25584, #35106 ),
 ( #18291, #1525, #93898 ),
 ( #55244, #79886, #64196 ),
 ( #89918, #28367, #30005 ),
 ( #72063, #96686, #54700 ),
 ( #2643, #54150, #106178 ),
 ( #106715, #37879, #72587 ),
 ( #79332, #88826, #98318 ) ),
 .UNSPECIFIED., .F., .F., .F. ) 
 B_SPLINE_SURFACE_WITH_KNOTS ( ( 4, 2, 2, 2, 4 ),
 ( 3, 3 ),
 ( 1.570796326794896558, 1.963495408493620697, 2.356194490192344837, 2.748893571891068976, 3.141592653589793116 ),
 ( 0.000000000000000000, 1.000000000000000000 ),
 .UNSPECIFIED. ) 
 GEOMETRIC_REPRESENTATION_ITEM ( )  RATIONAL_B_SPLINE_SURFACE ( (
 ( 1.000000000000000000, 0.7071067811865867636, 1.000000000000000000),
 ( 1.000000000000000000, 0.7166207884821557128, 1.000000000000000000),
 ( 1.000000000000000000, 0.7259222650907828367, 1.000000000000000000),
 ( 1.000000000000000000, 0.7428408967929600593, 1.000000000000000000),
 ( 1.000000000000000000, 0.7504512394524331942, 1.000000000000000000),
 ( 1.000000000000000000, 0.7630177051950730593, 1.000000000000000000),
 ( 1.000000000000000000, 0.7679730451978846739, 1.000000000000000000),
 ( 1.000000000000000000, 0.7746454561791621396, 1.000000000000000000),
 ( 1.000000000000000000, 0.7763684247039451813, 1.000000000000000000),
 ( 1.000000000000000000, 0.7763623250684347221, 1.000000000000000000) ) ) 
 REPRESENTATION_ITEM ( '' )  SURFACE ( )  );
#83119=ORIENTED_EDGE ( 'NONE', *, *, #20070, .T. ) ;
#83147=CARTESIAN_POINT ( 'NONE',  ( 3.024787391539412425E-15, 1523.409940573003951, 184.4225825198192013 ) ) ;
#83151=ORIENTED_EDGE ( 'NONE', *, *, #80522, .F. ) ;
#83154=FACE_OUTER_BOUND ( 'NONE', #100259, .T. ) ;
#83155=CARTESIAN_POINT ( 'NONE',  ( 204.2714532754875449, 1526.382868172863937, 223.7095399770875304 ) ) ;
#83163=CARTESIAN_POINT ( 'NONE',  ( 22.75273496409577945, 1512.187213306747481, 183.6728937936772184 ) ) ;
#83165=EDGE_LOOP ( 'NONE', ( #87095, #83069, #69740, #12670 ) ) ;
#83183=CIRCLE ( 'NONE', #38486, 1.000000000000057954 ) ;
#83206=CARTESIAN_POINT ( 'NONE',  ( -18.66420869458028164, 1526.382868172864164, 232.7837831374281166 ) ) ;
#83231=CARTESIAN_POINT ( 'NONE',  ( -2.470168521978401088, 1523.481610426287716, 175.3649660270905315 ) ) ;
#83238=ORIENTED_EDGE ( 'NONE', *, *, #56752, .T. ) ;
#83241=CARTESIAN_POINT ( 'NONE',  ( -20.87480701074316869, 1525.712835404586031, 184.1764597564572625 ) ) ;
#83250=DIRECTION ( 'NONE',  ( -1.734723475976805580E-13, 0.000000000000000000, 1.000000000000000000 ) ) ;
#83252=AXIS2_PLACEMENT_3D ( 'NONE', #82718, #6008, #109035 ) ;
#83260=CARTESIAN_POINT ( 'NONE',  ( -29.30029655192924309, 1525.907212628473644, 221.3719603026177367 ) ) ;
#83274=CYLINDRICAL_SURFACE ( 'NONE', #101174, 0.9999999999999927836 ) ;
#83276=CARTESIAN_POINT ( 'NONE',  ( 21.53712143570574611, 1523.621879633028584, 234.3036048850996451 ) ) ;
#83293=CARTESIAN_POINT ( 'NONE',  ( 3.297216976270555264E-15, 1524.340287715038357, 184.7892624828776320 ) ) ;
#83321=CARTESIAN_POINT ( 'NONE',  ( 33.93019615848955084, 1522.382868172863937, 220.5829544587961095 ) ) ;
#83327=EDGE_LOOP ( 'NONE', ( #64424, #21497, #3748, #59351 ) ) ;
#83342=VERTEX_POINT ( 'NONE', #84482 ) ;
#83370=DIRECTION ( 'NONE',  ( 0.4882662618185556469, -0.4884709562387110626, 0.7231819843448625829 ) ) ;
#83371=LINE ( 'NONE', #39730, #29335 ) ;
#83375=ORIENTED_EDGE ( 'NONE', *, *, #4853, .T. ) ;
#83385=VERTEX_POINT ( 'NONE', #506 ) ;
#83417=CARTESIAN_POINT ( 'NONE',  ( 32.05392771830349830, 1524.756004293091792, 202.1328669733503318 ) ) ;
#83422=PLANE ( 'NONE',  #90735 ) ;
#83433=CIRCLE ( 'NONE', #12002, 32.13701971169416538 ) ;
#83435=CARTESIAN_POINT ( 'NONE',  ( -22.74803453391479735, 1523.678648413191695, 183.6833808205264802 ) ) ;
#83437=CARTESIAN_POINT ( 'NONE',  ( -2.038847259689249736, 1522.382868172863937, 173.3106345060153046 ) ) ;
#83438=CYLINDRICAL_SURFACE ( 'NONE', #38448, 0.9999999999999942268 ) ;
#83450=B_SPLINE_CURVE_WITH_KNOTS ( 'NONE', 3,
 ( #53796, #11222, #2828, #11754 ),
 .UNSPECIFIED., .F., .F.,
 ( 4, 4 ),
 ( 0.000000000000000000, 0.0002220129587134778289 ),
 .UNSPECIFIED. ) ;
#83453=FACE_OUTER_BOUND ( 'NONE', #93554, .T. ) ;
#83456=DIRECTION ( 'NONE',  ( -0.000000000000000000, -1.000000000000000000, -0.000000000000000000 ) ) ;
#83466=VERTEX_POINT ( 'NONE', #50356 ) ;
#83473=EDGE_CURVE ( 'NONE', #3217, #89419, #6975, .T. ) ;
#83491=VERTEX_POINT ( 'NONE', #85021 ) ;
#83497=B_SPLINE_CURVE_WITH_KNOTS ( 'NONE', 3,
 ( #66919, #98839, #48462, #32739, #24326, #58509, #83690, #92639, #22099, #15913 ),
 .UNSPECIFIED., .F., .F.,
 ( 4, 2, 2, 2, 4 ),
 ( 0.000000000000000000, 0.0007403986298595332041, 0.001480797259719066408, 0.002221195889578599612, 0.002961594519438132816 ),
 .UNSPECIFIED. ) ;
#83500=DIRECTION ( 'NONE',  ( 0.000000000000000000, 1.000000000000000000, 0.000000000000000000 ) ) ;
#83502=AXIS2_PLACEMENT_3D ( 'NONE', #77378, #18541, #26972 ) ;
#83510=ORIENTED_EDGE ( 'NONE', *, *, #4958, .F. ) ;
#83517=CARTESIAN_POINT ( 'NONE',  ( 20.20959865099471031, 1522.382868172863937, 182.0120230947219966 ) ) ;
#83522=CARTESIAN_POINT ( 'NONE',  ( 29.41145171355093879, 1525.795403621571268, 221.5574853780759383 ) ) ;
#83537=CARTESIAN_POINT ( 'NONE',  ( 20.79738390328718722, 1511.187213306747708, 181.2030061003470394 ) ) ;
#83545=CIRCLE ( 'NONE', #65673, 1.000000000000000888 ) ;
#83547=VERTEX_POINT ( 'NONE', #69367 ) ;
#83548=LINE ( 'NONE', #107108, #12227 ) ;
#83550=CARTESIAN_POINT ( 'NONE',  ( -22.07691418023513918, 1523.843271061951100, 233.7988799057568201 ) ) ;
#83585=CIRCLE ( 'NONE', #101393, 0.9999999999999947820 ) ;
#83597=CARTESIAN_POINT ( 'NONE',  ( -16.48487877296663129, 1525.795403383247276, 236.4701076103954165 ) ) ;
#83605=ORIENTED_EDGE ( 'NONE', *, *, #31181, .T. ) ;
#83611=CARTESIAN_POINT ( 'NONE',  ( 21.83550407203906119, 1523.678648413191468, 183.2743720722706655 ) ) ;
#83613=CARTESIAN_POINT ( 'NONE',  ( 17.44950774654776282, 1525.163527997520305, 237.2402625269670580 ) ) ;
#83639=EDGE_CURVE ( 'NONE', #59940, #23656, #44560, .T. ) ;
#83643=FILL_AREA_STYLE ('',( #74172 ) ) ;
#83649=ORIENTED_EDGE ( 'NONE', *, *, #30950, .F. ) ;
#83672=EDGE_LOOP ( 'NONE', ( #71203, #56393, #11165, #75581 ) ) ;
#83685=CIRCLE ( 'NONE', #15714, 1.000000000000015099 ) ;
#83688=CARTESIAN_POINT ( 'NONE',  ( -21.95372433850575788, 1524.425415513989265, 233.6963910516591909 ) ) ;
#83690=CARTESIAN_POINT ( 'NONE',  ( 17.37723644544120560, 1525.394081235439444, 181.1943427199432790 ) ) ;
#83695=CARTESIAN_POINT ( 'NONE',  ( 31.33756686635629762, 1523.580204110582599, 196.3415365203907186 ) ) ;
#83701=EDGE_CURVE ( 'NONE', #81284, #24484, #30645, .T. ) ;
#83725=CARTESIAN_POINT ( 'NONE',  ( -19.53786426058999481, 1511.187213306747708, 237.7197124308268030 ) ) ;
#83729=ADVANCED_FACE ( 'NONE', ( #40144 ), #49118, .T. ) ;
#83737=CARTESIAN_POINT ( 'NONE',  ( 16.57584690634417157, 1524.538969332612623, 180.6844723161869979 ) ) ;
#83746=EDGE_CURVE ( 'NONE', #32838, #14716, #5137, .T. ) ;
#83751=CARTESIAN_POINT ( 'NONE',  ( -20.39893125376764615, 1526.069472839381206, 233.1323736274921998 ) ) ;
#83760=CARTESIAN_POINT ( 'NONE',  ( -2.737416067801649255, 1524.382868172804365, 241.6058578387446403 ) ) ;
#83764=AXIS2_PLACEMENT_3D ( 'NONE', #56811, #73063, #25788 ) ;
#83772=AXIS2_PLACEMENT_3D ( 'NONE', #102940, #59876, #41959 ) ;
#83781=CARTESIAN_POINT ( 'NONE',  ( 31.23437356469446868, 1518.913060387330006, 222.8968241038843701 ) ) ;
#83785=DIRECTION ( 'NONE',  ( 0.000000000000000000, 0.000000000000000000, 1.000000000000000000 ) ) ;
#83786=EDGE_CURVE ( 'NONE', #29284, #26062, #39088, .T. ) ;
#83794=DIRECTION ( 'NONE',  ( -0.000000000000000000, -1.000000000000000000, -0.000000000000000000 ) ) ;
#83827=CARTESIAN_POINT ( 'NONE',  ( 16.89232299734824494, 1526.349689584397083, 183.3465833397473261 ) ) ;
#83843=PLANE ( 'NONE',  #44011 ) ;
#83844=CARTESIAN_POINT ( 'NONE',  ( 2.471036798109852217, 1525.556089352344543, 176.9933267734384117 ) ) ;
#83863=CARTESIAN_POINT ( 'NONE',  ( -31.34137657907970365, 1523.481610118011986, 221.9025654077134391 ) ) ;
#83866=DIRECTION ( 'NONE',  ( -0.8672669759446666182, -0.000000000000000000, -0.4978433412588672557 ) ) ;
#83873=EDGE_CURVE ( 'NONE', #12155, #25949, #16559, .T. ) ;
#83885=DIRECTION ( 'NONE',  ( -2.664535259100376091E-15, 0.000000000000000000, -1.000000000000000000 ) ) ;
#83892=AXIS2_PLACEMENT_3D ( 'NONE', #87244, #86683, #53106 ) ;
#83893=EDGE_CURVE ( 'NONE', #94153, #44415, #101669, .T. ) ;
#83915=CIRCLE ( 'NONE', #21219, 0.9999999999999953371 ) ;
#83918=CIRCLE ( 'NONE', #98229, 30.13701971169416183 ) ;
#83932=VERTEX_POINT ( 'NONE', #86006 ) ;
#83933=ORIENTED_EDGE ( 'NONE', *, *, #32289, .F. ) ;
#83939=AXIS2_PLACEMENT_3D ( 'NONE', #84778, #26537, #84232 ) ;
#83940=LINE ( 'NONE', #109162, #9836 ) ;
#83952=VERTEX_POINT ( 'NONE', #24970 ) ;
#83979=CARTESIAN_POINT ( 'NONE',  ( -19.39983987835443457, 1501.977400791986611, 178.9515629539737631 ) ) ;
#83984=VECTOR ( 'NONE', #39699, 1000.000000000000000 ) ;
#83990=CIRCLE ( 'NONE', #89362, 1.000000000000000000 ) ;
#83992=FACE_OUTER_BOUND ( 'NONE', #78759, .T. ) ;
#83993=CARTESIAN_POINT ( 'NONE',  ( -76.99707197885182097, 1526.382868172863937, 19.35599459046246551 ) ) ;
#83995=CARTESIAN_POINT ( 'NONE',  ( -2.534335827540424191, 1523.982201850120191, 175.6705872193751929 ) ) ;
#84000=DIRECTION ( 'NONE',  ( 0.000000000000000000, 0.000000000000000000, 1.000000000000000000 ) ) ;
#84001=EDGE_LOOP ( 'NONE', ( #38614, #78706, #101911 ) ) ;
#84003=DIRECTION ( 'NONE',  ( -0.000000000000000000, -1.000000000000000000, -0.000000000000000000 ) ) ;
#84008=CARTESIAN_POINT ( 'NONE',  ( -17.44950774654834191, 1525.163527997503707, 181.0034293964202448 ) ) ;
#84011=CARTESIAN_POINT ( 'NONE',  ( 33.35590117750199113, 1523.678648413191695, 216.3310373540456339 ) ) ;
#84019=CARTESIAN_POINT ( 'NONE',  ( -19.33418355719779314, 1523.342713519623203, 239.2327152390762990 ) ) ;
#84034=FACE_OUTER_BOUND ( 'NONE', #12169, .T. ) ;
#84057=AXIS2_PLACEMENT_3D ( 'NONE', #67447, #32713, #66895 ) ;
#84064=ORIENTED_EDGE ( 'NONE', *, *, #58489, .F. ) ;
#84066=AXIS2_PLACEMENT_3D ( 'NONE', #87791, #35709, #44684 ) ;
#84074=CIRCLE ( 'NONE', #35808, 0.9999999999999991118 ) ;
#84088=VERTEX_POINT ( 'NONE', #27211 ) ;
#84093=DIRECTION ( 'NONE',  ( 0.000000000000000000, 0.000000000000000000, 1.000000000000000000 ) ) ;
#84101=CIRCLE ( 'NONE', #98405, 1.000000000000000888 ) ;
#84106=CARTESIAN_POINT ( 'NONE',  ( -21.48632729253362683, 1524.478200376951236, 234.0867245257886395 ) ) ;
#84123=CARTESIAN_POINT ( 'NONE',  ( -3.347801439296141712, 1523.382868172864164, 176.1543725841967500 ) ) ;
#84153=CARTESIAN_POINT ( 'NONE',  ( -16.48231804958369651, 1525.661276915132476, 236.6690270335203934 ) ) ;
#84161=CARTESIAN_POINT ( 'NONE',  ( 17.05907944273679178, 1524.678541297843367, 181.0477197495561370 ) ) ;
#84188=DIRECTION ( 'NONE',  ( -0.9510565162951541973, 0.000000000000000000, -0.3090169943749456194 ) ) ;
#84191=CARTESIAN_POINT ( 'NONE',  ( 17.17241001986483795, 1512.187213306747481, 179.6185504016043240 ) ) ;
#84196=DIRECTION ( 'NONE',  ( -0.000000000000000000, 1.000000000000000000, -0.000000000000000000 ) ) ;
#84198=DIRECTION ( 'NONE',  ( 0.000000000000000000, -1.000000000000000000, 0.000000000000000000 ) ) ;
#84209=CARTESIAN_POINT ( 'NONE',  ( -19.53786426058999481, 1512.187213306747481, 236.7197124308268030 ) ) ;
#84212=EDGE_LOOP ( 'NONE', ( #10625, #31896, #52469, #60555 ) ) ;
#84218=ORIENTED_EDGE ( 'NONE', *, *, #49598, .F. ) ;
#84232=DIRECTION ( 'NONE',  ( -0.6709778558543708638, 0.000000000000000000, 0.7414773880254684757 ) ) ;
#84241=DIRECTION ( 'NONE',  ( -0.4882662618185556469, -0.4884709562387110626, -0.7231819843448625829 ) ) ;
#84254=VECTOR ( 'NONE', #82074, 1000.000000000000000 ) ;
#84265=EDGE_CURVE ( 'NONE', #90367, #63483, #37135, .T. ) ;
#84275=CARTESIAN_POINT ( 'NONE',  ( -21.45462491533616856, 1525.320849883639539, 184.8030411736961298 ) ) ;
#84302=CARTESIAN_POINT ( 'NONE',  ( 31.44837959398592986, 1512.187213306747481, 220.9083067115976462 ) ) ;
#84309=CARTESIAN_POINT ( 'NONE',  ( -2.792392588003544507, 1524.382868172863937, 241.3440112565233449 ) ) ;
#84313=MECHANICAL_DESIGN_GEOMETRIC_PRESENTATION_REPRESENTATION('',(#62877),#66442);
#84317=ORIENTED_EDGE ( 'NONE', *, *, #90425, .T. ) ;
#84322=CARTESIAN_POINT ( 'NONE',  ( -31.41104781486813735, 1512.187213306747481, 215.9140555522426723 ) ) ;
#84324=AXIS2_PLACEMENT_3D ( 'NONE', #2862, #103071, #52155 ) ;
#84325=CARTESIAN_POINT ( 'NONE',  ( 2.273033093151322515, 1525.821544997590763, 240.9339456143064524 ) ) ;
#84335=ORIENTED_EDGE ( 'NONE', *, *, #25098, .F. ) ;
#84336=ORIENTED_EDGE ( 'NONE', *, *, #26404, .T. ) ;
#84338=VECTOR ( 'NONE', #85662, 1000.000000000000000 ) ;
#84339=DIRECTION ( 'NONE',  ( 0.000000000000000000, 1.000000000000000000, 0.000000000000000000 ) ) ;
#84342=DIRECTION ( 'NONE',  ( 0.000000000000000000, 1.000000000000000000, 0.000000000000000000 ) ) ;
#84348=AXIS2_PLACEMENT_3D ( 'NONE', #93603, #94165, #43780 ) ;
#84355=CARTESIAN_POINT ( 'NONE',  ( 30.61619818474186161, 1525.211477436245787, 196.6452937733279214 ) ) ;
#84359=CARTESIAN_POINT ( 'NONE',  ( -29.36670733768233887, 1526.000688113674414, 220.9053709888523827 ) ) ;
#84399=CARTESIAN_POINT ( 'NONE',  ( 3.317918599975760330, 1524.412928176729338, 176.3321646713325208 ) ) ;
#84410=VERTEX_POINT ( 'NONE', #45284 ) ;
#84412=CARTESIAN_POINT ( 'NONE',  ( -20.20959865099510111, 1512.187213306747481, 182.0120230947222524 ) ) ;
#84421=CARTESIAN_POINT ( 'NONE',  ( 3.350338079455601026, 1523.604703353109699, 242.0808062845893289 ) ) ;
#84422=FACE_OUTER_BOUND ( 'NONE', #9759, .T. ) ;
#84430=TOROIDAL_SURFACE ( 'NONE', #64809, 32.13701971169416538, 1.000000000000000000 ) ;
#84434=ORIENTED_EDGE ( 'NONE', *, *, #54340, .T. ) ;
#84469=EDGE_CURVE ( 'NONE', #71856, #36364, #89310, .T. ) ;
#84471=CARTESIAN_POINT ( 'NONE',  ( -33.28034951413935971, 1522.862737210649811, 200.8029765415142833 ) ) ;
#84482=CARTESIAN_POINT ( 'NONE',  ( -32.02808312589930040, 1511.187213306747708, 197.2787714533499752 ) ) ;
#84515=CARTESIAN_POINT ( 'NONE',  ( 30.30264253605709612, 1524.678541297860875, 196.4364760679688402 ) ) ;
#84516=CARTESIAN_POINT ( 'NONE',  ( -33.28034951413935971, 1501.977400791986611, 200.8029765415142549 ) ) ;
#84521=EDGE_LOOP ( 'NONE', ( #31817, #27838, #41899, #32726 ) ) ;
#84522=CARTESIAN_POINT ( 'NONE',  ( -32.86470156657997421, 1523.580204110582372, 201.0415738463118203 ) ) ;
#84546=CARTESIAN_POINT ( 'NONE',  ( -2.737416067801661690, 1524.382868172804365, 176.6378340846514448 ) ) ;
#84548=ADVANCED_FACE ( 'NONE', ( #35065 ), #96425, .T. ) ;
#84575=CARTESIAN_POINT ( 'NONE',  ( -2.157482617120746404, 1526.189899547014420, 240.2809648701897061 ) ) ;
#84576=ORIENTED_EDGE ( 'NONE', *, *, #70826, .F. ) ;
#84582=DIRECTION ( 'NONE',  ( 0.1070030146457386366, 0.000000000000000000, 0.9942586961433749204 ) ) ;
#84604=CARTESIAN_POINT ( 'NONE',  ( 21.42853521715711196, 1524.678541297860647, 234.0213767294899583 ) ) ;
#84611=ORIENTED_EDGE ( 'NONE', *, *, #32164, .F. ) ;
#84651=DIRECTION ( 'NONE',  ( 4.510281037539694659E-14, 0.000000000000000000, 1.000000000000000000 ) ) ;
#84653=CARTESIAN_POINT ( 'NONE',  ( -22.08327125186907125, 1523.604703353109699, 233.8169256665491105 ) ) ;
#84660=EDGE_CURVE ( 'NONE', #82365, #24499, #64309, .T. ) ;
#84681=CARTESIAN_POINT ( 'NONE',  ( 0.000000000000000000, 1523.382868172864164, 209.1218459616979999 ) ) ;
#84685=LINE ( 'NONE', #34290, #35833 ) ;
#84692=CARTESIAN_POINT ( 'NONE',  ( -30.83402112502179904, 1524.872178180563878, 196.5182538919386843 ) ) ;
#84702=( BOUNDED_SURFACE ( )  B_SPLINE_SURFACE ( 3, 2, ( 
 ( #25416, #103232, #95417 ),
 ( #34943, #61845, #10867 ),
 ( #18680, #45040, #52878 ),
 ( #1932, #86454, #10295 ),
 ( #70809, #69129, #79185 ),
 ( #60737, #25971, #94288 ),
 ( #94859, #18134, #44471 ),
 ( #78616, #27658, #59610 ),
 ( #9745, #17002, #76963 ),
 ( #51202, #43911, #78054 ),
 ( #85331, #8628, #42803 ),
 ( #37167, #88134, #71915 ),
 ( #13582, #89762, #20891 ),
 ( #81347, #64040, #4128 ) ),
 .UNSPECIFIED., .F., .F., .F. ) 
 B_SPLINE_SURFACE_WITH_KNOTS ( ( 4, 2, 2, 2, 2, 2, 4 ),
 ( 3, 3 ),
 ( 0.000000000000000000, 0.0009440840677145154007, 0.001416126101571773101, 0.001888168135429030801, 0.002360210169286288719, 0.002832252203143546202, 0.003776336270858061603 ),
 ( 0.000000000000000000, 1.000000000000000000 ),
 .UNSPECIFIED. ) 
 GEOMETRIC_REPRESENTATION_ITEM ( )  RATIONAL_B_SPLINE_SURFACE ( (
 ( 1.000000000000000000, 0.8070209408750085300, 1.000000000000000000),
 ( 1.000000000000000000, 0.8215603905277785168, 1.000000000000000000),
 ( 1.000000000000000000, 0.8340988699069226131, 1.000000000000000000),
 ( 1.000000000000000000, 0.8516751610454621479, 1.000000000000000000),
 ( 1.000000000000000000, 0.8573697395118552445, 1.000000000000000000),
 ( 1.000000000000000000, 0.8683586635697856382, 1.000000000000000000),
 ( 1.000000000000000000, 0.8736518481707646888, 1.000000000000000000),
 ( 1.000000000000000000, 0.8840377753031072317, 1.000000000000000000),
 ( 1.000000000000000000, 0.8891294171307223548, 1.000000000000000000),
 ( 1.000000000000000000, 0.8992456600573884851, 1.000000000000000000),
 ( 1.000000000000000000, 0.9042785869247129682, 1.000000000000000000),
 ( 1.000000000000000000, 0.9189749222850194244, 1.000000000000000000),
 ( 1.000000000000000000, 0.9283978182339867047, 1.000000000000000000),
 ( 1.000000000000000000, 0.9376006582765946673, 1.000000000000000000) ) ) 
 REPRESENTATION_ITEM ( '' )  SURFACE ( )  );
#84709=CARTESIAN_POINT ( 'NONE',  ( 16.85976061912555579, 1525.821544997590308, 182.0492613858612003 ) ) ;
#84717=VECTOR ( 'NONE', #66746, 1000.000000000000000 ) ;
#84720=DIRECTION ( 'NONE',  ( -0.6709778558543747495, 0.000000000000000000, 0.7414773880254650340 ) ) ;
#84726=CIRCLE ( 'NONE', #36461, 1.000000000000085043 ) ;
#84732=ORIENTED_EDGE ( 'NONE', *, *, #7293, .T. ) ;
#84749=CIRCLE ( 'NONE', #52559, 1.000000000000007994 ) ;
#84754=FACE_OUTER_BOUND ( 'NONE', #15311, .T. ) ;
#84765=DIRECTION ( 'NONE',  ( 0.9942586961433743653, 0.000000000000000000, -0.1070030146457445208 ) ) ;
#84774=FACE_OUTER_BOUND ( 'NONE', #49893, .T. ) ;
#84778=CARTESIAN_POINT ( 'NONE',  ( 18.51436573157378618, 1512.187213306747481, 237.1421867457405881 ) ) ;
#84804=DIRECTION ( 'NONE',  ( -0.000000000000000000, -1.000000000000000000, -0.000000000000000000 ) ) ;
#84809=LINE ( 'NONE', #42275, #71779 ) ;
#84812=CARTESIAN_POINT ( 'NONE',  ( -21.08094518543032336, 1525.506926151470907, 184.0391977492186015 ) ) ;
#84813=DIRECTION ( 'NONE',  ( -0.000000000000000000, -1.000000000000000000, -0.000000000000000000 ) ) ;
#84820=CARTESIAN_POINT ( 'NONE',  ( -0.4151546846821903003, 1522.382868172863937, 173.3106345060153046 ) ) ;
#84843=CARTESIAN_POINT ( 'NONE',  ( -0.8350686643532179154, 1526.382868172863937, 240.9330574173806951 ) ) ;
#84853=ADVANCED_FACE ( 'NONE', ( #55766 ), #107262, .F. ) ;
#84858=DIRECTION ( 'NONE',  ( 1.000000000000000000, -0.000000000000000000, -0.000000000000000000 ) ) ;
#84859=EDGE_CURVE ( 'NONE', #96103, #105990, #31625, .T. ) ;
#84873=EDGE_LOOP ( 'NONE', ( #70486, #109680, #27748, #94117 ) ) ;
#84884=EDGE_CURVE ( 'NONE', #24269, #5750, #91049, .T. ) ;
#84886=B_SPLINE_CURVE_WITH_KNOTS ( 'NONE', 3,
 ( #102668, #25967, #60166, #94284, #51763, #58506, #23770, #92090, #67030, #102253, #100596, #7645 ),
 .UNSPECIFIED., .F., .F.,
 ( 4, 2, 2, 2, 2, 4 ),
 ( 0.000000000000000000, 0.0007194225121792683416, 0.001079133768269217473, 0.001438845024359166388, 0.002158267536539043834, 0.002877690048718921281 ),
 .UNSPECIFIED. ) ;
#84890=EDGE_CURVE ( 'NONE', #37235, #17035, #5223, .T. ) ;
#84913=ADVANCED_FACE ( 'NONE', ( #67466 ), #24859, .T. ) ;
#84919=DIRECTION ( 'NONE',  ( 0.000000000000000000, 0.000000000000000000, -1.000000000000000000 ) ) ;
#84925=ORIENTED_EDGE ( 'NONE', *, *, #56186, .F. ) ;
#84930=CARTESIAN_POINT ( 'NONE',  ( 3.350338079455601026, 1523.604703353109699, 176.1628856388066708 ) ) ;
#84942=CARTESIAN_POINT ( 'NONE',  ( 2.792392588003544507, 1524.382868172863937, 241.3440112565233449 ) ) ;
#84945=CARTESIAN_POINT ( 'NONE',  ( 28.27139721233048419, 1526.382868172863937, 219.5606225550385489 ) ) ;
#84961=CARTESIAN_POINT ( 'NONE',  ( 31.74003925670048432, 1524.382868172804365, 216.5565202880893594 ) ) ;
#84965=CARTESIAN_POINT ( 'NONE',  ( 32.38845791999495560, 1512.187213306747481, 202.1182848005512085 ) ) ;
#84967=EDGE_LOOP ( 'NONE', ( #16304, #2431, #34886, #13979 ) ) ;
#84969=CARTESIAN_POINT ( 'NONE',  ( 29.65946186579095922, 1526.335487865669393, 201.2508909606647478 ) ) ;
#84972=CARTESIAN_POINT ( 'NONE',  ( 31.34137657934008558, 1523.382868172864164, 196.3411265156547358 ) ) ;
#84998=VECTOR ( 'NONE', #86285, 1000.000000000000000 ) ;
#85015=CARTESIAN_POINT ( 'NONE',  ( -3.143095077906852719, 1525.137881624898682, 176.7009515179215668 ) ) ;
#85021=CARTESIAN_POINT ( 'NONE',  ( 16.73628186595824019, 1526.382868172863937, 184.0591879540915272 ) ) ;
#85023=DIRECTION ( 'NONE',  ( -0.9786619618251634067, 0.000000000000000000, -0.2054769195713292418 ) ) ;
#85060=CARTESIAN_POINT ( 'NONE',  ( 2.570808432944288846, 1525.317359687841190, 241.4588331507368650 ) ) ;
#85062=CARTESIAN_POINT ( 'NONE',  ( -32.23393008293517425, 1523.462669333491021, 201.4036600224246740 ) ) ;
#85064=CARTESIAN_POINT ( 'NONE',  ( 31.63978151511877357, 1525.343710797494396, 202.0582079856336577 ) ) ;
#85065=ADVANCED_FACE ( 'NONE', ( #102956 ), #24185, .T. ) ;
#85076=AXIS2_PLACEMENT_3D ( 'NONE', #64862, #81075, #106820 ) ;
#85078=CARTESIAN_POINT ( 'NONE',  ( -17.17241001986462123, 1512.187213306747481, 237.6251415217917895 ) ) ;
#85109=B_SPLINE_CURVE_WITH_KNOTS ( 'NONE', 3,
 ( #8723, #42903, #77060, #34493, #23863, #102771, #60259, #83241, #40686, #74859 ),
 .UNSPECIFIED., .F., .F.,
 ( 4, 2, 2, 2, 4 ),
 ( 3.469446951953614189E-18, 0.0007403986298595378662, 0.001480797259719072263, 0.002221195889578606551, 0.002961594519438141056 ),
 .UNSPECIFIED. ) ;
#85121=AXIS2_PLACEMENT_3D ( 'NONE', #74391, #21170, #43194 ) ;
#85137=CARTESIAN_POINT ( 'NONE',  ( -29.33952678943212433, 1526.382868172864164, 217.1408869592854671 ) ) ;
#85141=CARTESIAN_POINT ( 'NONE',  ( -31.63978151511851777, 1525.343710797494396, 216.1854839377624842 ) ) ;
#85175=CARTESIAN_POINT ( 'NONE',  ( -2.470955850358403705, 1523.580204110582144, 242.8749759455149615 ) ) ;
#85202=ORIENTED_EDGE ( 'NONE', *, *, #55265, .T. ) ;
#85223=CARTESIAN_POINT ( 'NONE',  ( -21.38516915557942255, 1524.726013923371283, 237.8497028174240029 ) ) ;
#85235=ORIENTED_EDGE ( 'NONE', *, *, #89780, .T. ) ;
#85259=CARTESIAN_POINT ( 'NONE',  ( 16.94363731710740595, 1525.231909165033585, 181.3784879451278584 ) ) ;
#85276=ORIENTED_EDGE ( 'NONE', *, *, #36996, .F. ) ;
#85323=CARTESIAN_POINT ( 'NONE',  ( 21.41029105012001921, 1526.329757971583831, 184.2230555347920529 ) ) ;
#85331=CARTESIAN_POINT ( 'NONE',  ( 29.70307915522525732, 1525.408327360769590, 221.9454130908924583 ) ) ;
#85341=CARTESIAN_POINT ( 'NONE',  ( -31.34137657934000387, 1523.382868172864164, 221.9025654077414345 ) ) ;
#85342=CIRCLE ( 'NONE', #31722, 1.000000000000000888 ) ;
#85345=CARTESIAN_POINT ( 'NONE',  ( 32.78250617288044566, 1511.187213306747708, 218.3079823578266314 ) ) ;
#85354=( BOUNDED_SURFACE ( )  B_SPLINE_SURFACE ( 3, 2, ( 
 ( #431, #74510, #108640 ),
 ( #101738, #34550, #59228 ),
 ( #103961, #88274, #37874 ),
 ( #105637, #12664, #95565 ) ),
 .UNSPECIFIED., .F., .F., .F. ) 
 B_SPLINE_SURFACE_WITH_KNOTS ( ( 4, 4 ),
 ( 3, 3 ),
 ( 0.000000000000000000, 0.0002960034161023848394 ),
 ( 0.000000000000000000, 1.000000000000000000 ),
 .UNSPECIFIED. ) 
 GEOMETRIC_REPRESENTATION_ITEM ( )  RATIONAL_B_SPLINE_SURFACE ( (
 ( 1.000000000000000000, 0.8070209408750156355, 1.000000000000000000),
 ( 1.000000000000000000, 0.8071723757218154383, 1.000000000000000000),
 ( 1.000000000000000000, 0.8072480346917759730, 1.000000000000000000),
 ( 1.000000000000000000, 0.8072480644198091193, 1.000000000000000000) ) ) 
 REPRESENTATION_ITEM ( '' )  SURFACE ( )  );
#85360=DIRECTION ( 'NONE',  ( -0.05752486295818490941, -0.9969860201949397593, 0.05205540968523030693 ) ) ;
#85363=CARTESIAN_POINT ( 'NONE',  ( -21.42853521715671761, 1524.678541297860875, 184.2223151939084005 ) ) ;
#85364=FACE_OUTER_BOUND ( 'NONE', #64739, .T. ) ;
#85373=DIRECTION ( 'NONE',  ( -0.5877852522924746914, 0.000000000000000000, -0.8090169943749463410 ) ) ;
#85409=CARTESIAN_POINT ( 'NONE',  ( 2.596261494520237800, 1525.907212628473644, 240.7735774411711702 ) ) ;
#85418=ORIENTED_EDGE ( 'NONE', *, *, #52429, .F. ) ;
#85444=LINE ( 'NONE', #102258, #94961 ) ;
#85462=CARTESIAN_POINT ( 'NONE',  ( -17.03788438627360691, 1524.775785348137561, 237.1518578317898118 ) ) ;
#85478=CARTESIAN_POINT ( 'NONE',  ( 2.708816481117918507, 1524.478200376951463, 176.2954886323626056 ) ) ;
#85485=CYLINDRICAL_SURFACE ( 'NONE', #2075, 2.000000000000006217 ) ;
#85492=CARTESIAN_POINT ( 'NONE',  ( 28.70874162694008547, 1526.306647125542668, 220.3434987316592526 ) ) ;
#85504=CIRCLE ( 'NONE', #76572, 2.000000000000002665 ) ;
#85562=CYLINDRICAL_SURFACE ( 'NONE', #83892, 1.999999999999996225 ) ;
#85567=CARTESIAN_POINT ( 'NONE',  ( 20.92767404034498568, 1511.187213306747708, 182.8548762971663848 ) ) ;
#85572=CARTESIAN_POINT ( 'NONE',  ( -31.23437356469453263, 1523.382868172864164, 195.3468678195118287 ) ) ;
#85602=DIRECTION ( 'NONE',  ( -0.5877852522924629231, 0.000000000000000000, 0.8090169943749548898 ) ) ;
#85603=CARTESIAN_POINT ( 'NONE',  ( -16.54106930751559190, 1524.860077346004800, 180.8551645285683662 ) ) ;
#85611=LINE ( 'NONE', #66652, #26611 ) ;
#85612=DIRECTION ( 'NONE',  ( 0.000000000000000000, 1.000000000000000000, 0.000000000000000000 ) ) ;
#85647=AXIS2_PLACEMENT_3D ( 'NONE', #24310, #13500, #91881 ) ;
#85649=CARTESIAN_POINT ( 'NONE',  ( 3.347801439296141268, 1512.187213306747481, 176.1543725841967500 ) ) ;
#85654=ADVANCED_FACE ( 'NONE', ( #77142 ), #8796, .T. ) ;
#85662=DIRECTION ( 'NONE',  ( 0.000000000000000000, 1.000000000000000000, 0.000000000000000000 ) ) ;
#85668=EDGE_LOOP ( 'NONE', ( #18642, #82148, #10954, #21177 ) ) ;
#85677=( BOUNDED_SURFACE ( )  B_SPLINE_SURFACE ( 3, 2, ( 
 ( #49566, #64729, #56304 ),
 ( #90434, #66379, #83695 ),
 ( #13712, #47898, #31636 ),
 ( #74225, #41146, #6448 ) ),
 .UNSPECIFIED., .F., .F., .T. ) 
 B_SPLINE_SURFACE_WITH_KNOTS ( ( 4, 4 ),
 ( 3, 3 ),
 ( 0.000000000000000000, 0.0002960034161023845684 ),
 ( 0.000000000000000000, 1.000000000000000000 ),
 .UNSPECIFIED. ) 
 GEOMETRIC_REPRESENTATION_ITEM ( )  RATIONAL_B_SPLINE_SURFACE ( (
 ( 1.000000000000000000, 0.8070209408749979829, 1.000000000000000000),
 ( 1.000000000000000000, 0.8071723757218428608, 1.000000000000000000),
 ( 1.000000000000000000, 0.8072480346917620952, 1.000000000000000000),
 ( 1.000000000000000000, 0.8072480644198127830, 1.000000000000000000) ) ) 
 REPRESENTATION_ITEM ( '' )  SURFACE ( )  );
#85678=CARTESIAN_POINT ( 'NONE',  ( -17.84338787571902074, 1512.187213306747481, 237.8836641337663309 ) ) ;
#85691=DIRECTION ( 'NONE',  ( 0.000000000000000000, 1.000000000000000000, 0.000000000000000000 ) ) ;
#85699=ORIENTED_EDGE ( 'NONE', *, *, #88708, .F. ) ;
#85707=CARTESIAN_POINT ( 'NONE',  ( 21.53712143570577453, 1523.621879633029039, 234.3036048850995883 ) ) ;
#85718=VERTEX_POINT ( 'NONE', #6485 ) ;
#85734=ORIENTED_EDGE ( 'NONE', *, *, #80239, .T. ) ;
#85748=DIRECTION ( 'NONE',  ( -0.9942586961433764747, -0.000000000000000000, -0.1070030146457237041 ) ) ;
#85758=AXIS2_PLACEMENT_3D ( 'NONE', #56450, #82185, #38528 ) ;
#85760=CARTESIAN_POINT ( 'NONE',  ( -20.53760542139741929, 1525.821544997590081, 233.5223198772807791 ) ) ;
#85770=CARTESIAN_POINT ( 'NONE',  ( -21.12212911287052464, 1511.187213306747708, 182.4210318429776692 ) ) ;
#85777=CARTESIAN_POINT ( 'NONE',  ( 0.4151546846821903003, 1522.382868172863937, 244.9330574173806951 ) ) ;
#85789=CARTESIAN_POINT ( 'NONE',  ( 32.38845792001180968, 1523.456924617338473, 216.1254071227668589 ) ) ;
#85804=CARTESIAN_POINT ( 'NONE',  ( 30.29107790644764009, 1523.847233649538339, 195.7510835363660533 ) ) ;
#85814=CARTESIAN_POINT ( 'NONE',  ( -16.66231036550682987, 1523.604703353109699, 237.7554842931448036 ) ) ;
#85818=CARTESIAN_POINT ( 'NONE',  ( 16.66700976312913696, 1523.530935881284904, 180.4846138748685007 ) ) ;
#85841=SURFACE_STYLE_USAGE ( .BOTH. , #51700 ) ;
#85865=ORIENTED_EDGE ( 'NONE', *, *, #103228, .T. ) ;
#85892=DIRECTION ( 'NONE',  ( -0.000000000000000000, -1.000000000000000000, -0.000000000000000000 ) ) ;
#85904=CIRCLE ( 'NONE', #109173, 2.000000000000006661 ) ;
#85908=FACE_OUTER_BOUND ( 'NONE', #49422, .T. ) ;
#85911=VECTOR ( 'NONE', #100291, 1000.000000000000000 ) ;
#85913=EDGE_CURVE ( 'NONE', #53799, #56488, #37504, .T. ) ;
#85922=CARTESIAN_POINT ( 'NONE',  ( 1.393816646507353596, 1512.187213306747481, 175.1051575864439656 ) ) ;
#85941=AXIS2_PLACEMENT_3D ( 'NONE', #62683, #69972, #3316 ) ;
#85945=CARTESIAN_POINT ( 'NONE',  ( 33.93019615849225801, 1522.906561336852519, 197.6607374646082178 ) ) ;
#85948=CARTESIAN_POINT ( 'NONE',  ( 20.79738390328738973, 1511.187213306747708, 237.0406858230487899 ) ) ;
#85956=VERTEX_POINT ( 'NONE', #102048 ) ;
#85981=CARTESIAN_POINT ( 'NONE',  ( -32.48455292688703366, 1524.659148609483054, 201.1731995520806038 ) ) ;
#85993=VERTEX_POINT ( 'NONE', #9113 ) ;
#85994=VERTEX_POINT ( 'NONE', #7454 ) ;
#86006=CARTESIAN_POINT ( 'NONE',  ( 0.8350686643532192477, 1526.382868172863937, 240.9330574173806951 ) ) ;
#86022=CARTESIAN_POINT ( 'NONE',  ( -30.01482722727578434, 1525.231909165033585, 221.6074739429450915 ) ) ;
#86054=CARTESIAN_POINT ( 'NONE',  ( 2.273033093151346939, 1525.821544997590308, 177.3097463090895189 ) ) ;
#86055=PRODUCT_DEFINITION_CONTEXT ( 'detailed design', #97107, 'design' ) ;
#86057=CARTESIAN_POINT ( 'NONE',  ( -31.97190655716365626, 1524.330813522192102, 201.5540712235616638 ) ) ;
#86067=ORIENTED_EDGE ( 'NONE', *, *, #12530, .T. ) ;
#86073=CARTESIAN_POINT ( 'NONE',  ( -19.53786426059057746, 1511.187213306747708, 180.5239794925695946 ) ) ;
#86082=ADVANCED_FACE ( 'NONE', ( #51678 ), #109056, .T. ) ;
#86084=ORIENTED_EDGE ( 'NONE', *, *, #84265, .T. ) ;
#86091=DIRECTION ( 'NONE',  ( 6.938893903907222067E-15, 0.000000000000000000, 1.000000000000000000 ) ) ;
#86114=AXIS2_PLACEMENT_3D ( 'NONE', #99513, #81616, #30676 ) ;
#86128=CARTESIAN_POINT ( 'NONE',  ( -33.13357216314891929, 1523.313115944345554, 200.8872321731306272 ) ) ;
#86134=CARTESIAN_POINT ( 'NONE',  ( -2.214867471995963566, 1525.730671948510917, 176.6953685902578570 ) ) ;
#86137=CARTESIAN_POINT ( 'NONE',  ( 3.451191875628176753, 1523.678648413191695, 243.0729557893954791 ) ) ;
#86161=DIRECTION ( 'NONE',  ( 0.8386695113602913310, -0.4884709562387192228, -0.2408932868012753081 ) ) ;
#86173=CARTESIAN_POINT ( 'NONE',  ( 30.25956561551600998, 1524.775785348137788, 196.4597071787796665 ) ) ;
#86180=ORIENTED_EDGE ( 'NONE', *, *, #84890, .T. ) ;
#86181=CARTESIAN_POINT ( 'NONE',  ( -2.038646110889675178, 1525.960063244516959, 177.0579350083066004 ) ) ;
#86197=CARTESIAN_POINT ( 'NONE',  ( 18.19590854888164699, 1512.187213306747481, 238.2026672068774644 ) ) ;
#86212=CARTESIAN_POINT ( 'NONE',  ( -31.75407494088130278, 1525.055427061272439, 216.6568988463208996 ) ) ;
#86223=CARTESIAN_POINT ( 'NONE',  ( 0.000000000000000000, 1523.051704408389696, 209.1218459616979999 ) ) ;
#86252=EDGE_LOOP ( 'NONE', ( #67192, #78437, #45909, #45369 ) ) ;
#86275=ORIENTED_EDGE ( 'NONE', *, *, #1250, .T. ) ;
#86285=DIRECTION ( 'NONE',  ( 0.3090169943749447312, 0.000000000000000000, -0.9510565162951544194 ) ) ;
#86290=ORIENTED_EDGE ( 'NONE', *, *, #89272, .T. ) ;
#86294=CARTESIAN_POINT ( 'NONE',  ( 31.23437356469446158, 1523.382868172864164, 222.8968241038843416 ) ) ;
#86300=EDGE_CURVE ( 'NONE', #82949, #59940, #80440, .T. ) ;
#86301=DIRECTION ( 'NONE',  ( -0.000000000000000000, 1.000000000000000000, -0.000000000000000000 ) ) ;
#86312=DIRECTION ( 'NONE',  ( -0.9942586961433749204, -0.000000000000000000, 0.1070030146457375819 ) ) ;
#86315=ORIENTED_EDGE ( 'NONE', *, *, #47763, .F. ) ;
#86317=CARTESIAN_POINT ( 'NONE',  ( -21.45464262047638115, 1525.320827368860591, 233.4406584548679859 ) ) ;
#86340=CARTESIAN_POINT ( 'NONE',  ( 32.38114538885255200, 1523.604703353109699, 216.1203639561429100 ) ) ;
#86356=DIRECTION ( 'NONE',  ( 0.000000000000000000, 1.000000000000000000, 0.000000000000000000 ) ) ;
#86389=LINE ( 'NONE', #110491, #3692 ) ;
#86390=SURFACE_STYLE_FILL_AREA ( #94796 ) ;
#86393=ORIENTED_EDGE ( 'NONE', *, *, #1250, .F. ) ;
#86394=ORIENTED_EDGE ( 'NONE', *, *, #17853, .T. ) ;
#86396=CARTESIAN_POINT ( 'NONE',  ( 21.48632729253213114, 1524.478200376968971, 184.1569673976052570 ) ) ;
#86399=EDGE_CURVE ( 'NONE', #75960, #54639, #7133, .T. ) ;
#86416=ORIENTED_EDGE ( 'NONE', *, *, #61737, .T. ) ;
#86418=ADVANCED_FACE ( 'NONE', ( #35283 ), #97800, .F. ) ;
#86419=DIRECTION ( 'NONE',  ( 0.9942586961433758086, -0.000000000000000000, 0.1070030146457303932 ) ) ;
#86445=CARTESIAN_POINT ( 'NONE',  ( 22.69876404239850132, 1522.861859112239472, 181.3483716558253036 ) ) ;
#86454=CARTESIAN_POINT ( 'NONE',  ( 30.41961987998531569, 1524.374578187333100, 221.8533450253357842 ) ) ;
#86471=CYLINDRICAL_SURFACE ( 'NONE', #93117, 1.000000000000000888 ) ;
#86476=DIRECTION ( 'NONE',  ( 0.000000000000000000, 1.000000000000000000, 0.000000000000000000 ) ) ;
#86482=ORIENTED_EDGE ( 'NONE', *, *, #31692, .F. ) ;
#86491=CARTESIAN_POINT ( 'NONE',  ( -33.93019615848960768, 1522.382868172863937, 197.6607374646000892 ) ) ;
#86518=CARTESIAN_POINT ( 'NONE',  ( 0.000000000000000000, 1526.382868172863937, 209.1218459616979999 ) ) ;
#86523=ORIENTED_EDGE ( 'NONE', *, *, #45214, .F. ) ;
#86529=CARTESIAN_POINT ( 'NONE',  ( -32.13446200735376834, 1525.163457223744444, 201.2154439896625888 ) ) ;
#86532=DIRECTION ( 'NONE',  ( 0.9786619618251657382, 0.000000000000000000, 0.2054769195713184449 ) ) ;
#86565=CIRCLE ( 'NONE', #90146, 1.000000000000000888 ) ;
#86633=ORIENTED_EDGE ( 'NONE', *, *, #12608, .F. ) ;
#86652=DIRECTION ( 'NONE',  ( 0.8672669759446700599, -0.000000000000000000, 0.4978433412588614271 ) ) ;
#86661=DIRECTION ( 'NONE',  ( 0.9942586961433756976, 0.000000000000000000, 0.1070030146457303794 ) ) ;
#86664=DIRECTION ( 'NONE',  ( 0.000000000000000000, 1.000000000000000000, 0.000000000000000000 ) ) ;
#86677=B_SPLINE_CURVE_WITH_KNOTS ( 'NONE', 3,
 ( #98617, #107024, #22999, #73987, #81809, #74545 ),
 .UNSPECIFIED., .F., .F.,
 ( 4, 2, 4 ),
 ( -1.131363979615173359E-05, 0.001067788114096062746, 0.002146889867988277523 ),
 .UNSPECIFIED. ) ;
#86679=ORIENTED_EDGE ( 'NONE', *, *, #31652, .T. ) ;
#86682=CARTESIAN_POINT ( 'NONE',  ( -2.038646110889526852, 1525.960063244517187, 177.0579350083066856 ) ) ;
#86683=DIRECTION ( 'NONE',  ( -0.4090087482554183862, 0.000000000000000000, 0.9125304618754026542 ) ) ;
#86726=CARTESIAN_POINT ( 'NONE',  ( -32.02808312589930040, 1512.187213306747481, 198.2787714533499752 ) ) ;
#86733=CARTESIAN_POINT ( 'NONE',  ( 2.038646110889527296, 1525.960063244517187, 241.1857569150893141 ) ) ;
#86736=CARTESIAN_POINT ( 'NONE',  ( 21.86721050905302377, 1523.611961620354123, 235.0400593884480713 ) ) ;
#86746=B_SPLINE_CURVE_WITH_KNOTS ( 'NONE', 3,
 ( #29954, #37273, #80925, #20438, #72008, #53537 ),
 .UNSPECIFIED., .F., .F.,
 ( 4, 2, 4 ),
 ( 1.040834085586084257E-17, 0.001087661325621716189, 0.002175322651243421970 ),
 .UNSPECIFIED. ) ;
#86756=CARTESIAN_POINT ( 'NONE',  ( 32.30068554584615725, 1526.382868172863937, 220.2363794648143198 ) ) ;
#86764=ORIENTED_EDGE ( 'NONE', *, *, #50933, .T. ) ;
#86778=DIRECTION ( 'NONE',  ( 0.000000000000000000, 0.000000000000000000, 1.000000000000000000 ) ) ;
#86784=ORIENTED_EDGE ( 'NONE', *, *, #56186, .T. ) ;
#86803=CARTESIAN_POINT ( 'NONE',  ( -2.472529913803023227, 1523.678648413191695, 175.3762130535718597 ) ) ;
#86809=EDGE_LOOP ( 'NONE', ( #15527, #109425, #54525, #51381, #31875 ) ) ;
#86814=CIRCLE ( 'NONE', #95768, 2.000000000000003997 ) ;
#86839=AXIS2_PLACEMENT_3D ( 'NONE', #16632, #50829, #34017 ) ;
#86849=DIRECTION ( 'NONE',  ( -0.5877852522924820189, 0.000000000000000000, -0.8090169943749410120 ) ) ;
#86852=AXIS2_PLACEMENT_3D ( 'NONE', #33376, #59174, #102779 ) ;
#86853=LINE ( 'NONE', #78462, #95457 ) ;
#86868=CARTESIAN_POINT ( 'NONE',  ( -0.4151546846821903003, 1522.382868172863937, 244.9330574173806951 ) ) ;
#86869=CARTESIAN_POINT ( 'NONE',  ( -20.92528053747092542, 1525.790287071788953, 233.2531890063321498 ) ) ;
#86871=FACE_OUTER_BOUND ( 'NONE', #102924, .T. ) ;
#86880=CARTESIAN_POINT ( 'NONE',  ( -1.484157417262785383, 1526.349684470114653, 239.9035629046661597 ) ) ;
#86901=CARTESIAN_POINT ( 'NONE',  ( 22.03465957474571013, 1522.862737210650039, 235.4136513321629991 ) ) ;
#86903=ADVANCED_FACE ( 'NONE', ( #102149 ), #15384, .F. ) ;
#86912=CARTESIAN_POINT ( 'NONE',  ( -29.55269881708379742, 1525.821544997590308, 197.1295836072967234 ) ) ;
#86929=CARTESIAN_POINT ( 'NONE',  ( 18.19590854888166476, 1522.382868172863937, 238.2026672068774360 ) ) ;
#86940=CARTESIAN_POINT ( 'NONE',  ( -30.79916350759976851, 1526.104292489138288, 201.1259370313427439 ) ) ;
#86949=CARTESIAN_POINT ( 'NONE',  ( 20.92528053747592054, 1525.790287071777357, 184.9905029170446085 ) ) ;
#86996=CARTESIAN_POINT ( 'NONE',  ( 22.03465957474218229, 1522.644714754858796, 182.8300405912402766 ) ) ;
#87000=CIRCLE ( 'NONE', #92334, 1.000000000000000888 ) ;
#87010=CARTESIAN_POINT ( 'NONE',  ( 30.90487439922551616, 1525.907212628473644, 216.4335774778779466 ) ) ;
#87023=DIRECTION ( 'NONE',  ( -1.000000000000000000, 0.000000000000000000, 0.000000000000000000 ) ) ;
#87033=CARTESIAN_POINT ( 'NONE',  ( -30.31643683089974317, 1523.530935881284904, 222.4932308532208083 ) ) ;
#87047=CARTESIAN_POINT ( 'NONE',  ( -31.81407709660168948, 1522.644714754858114, 196.2902540610638766 ) ) ;
#87050=CIRCLE ( 'NONE', #60211, 1.000000000000003775 ) ;
#87067=CARTESIAN_POINT ( 'NONE',  ( 3.350338079455601026, 1523.604703353109699, 176.1628856388066708 ) ) ;
#87069=EDGE_CURVE ( 'NONE', #68807, #83932, #103675, .T. ) ;
#87080=ORIENTED_EDGE ( 'NONE', *, *, #31652, .F. ) ;
#87087=CARTESIAN_POINT ( 'NONE',  ( -31.75409331310280692, 1525.055402519434210, 201.5867938956818364 ) ) ;
#87095=ORIENTED_EDGE ( 'NONE', *, *, #109812, .T. ) ;
#87121=TOROIDAL_SURFACE ( 'NONE', #105031, 1.000000000000000000, 1.000000000000000000 ) ;
#87130=CARTESIAN_POINT ( 'NONE',  ( -30.00906687502022407, 1525.856064936166604, 221.1186969528658608 ) ) ;
#87143=( BOUNDED_SURFACE ( )  B_SPLINE_SURFACE ( 3, 2, ( 
 ( #84653, #42119, #58375 ),
 ( #83550, #32615, #15768 ),
 ( #66791, #48887, #58924 ),
 ( #108764, #100891, #93055 ),
 ( #8493, #84106, #7406 ),
 ( #32057, #109871, #76267 ),
 ( #16328, #67890, #101998 ),
 ( #25284, #59484, #93595 ),
 ( #16872, #51077, #42665 ),
 ( #86317, #61161, #1229 ),
 ( #52734, #28622, #9059 ),
 ( #70663, #44899, #79591 ),
 ( #86869, #51624, #104778 ),
 ( #44336, #85760, #103101 ) ),
 .UNSPECIFIED., .F., .F., .F. ) 
 B_SPLINE_SURFACE_WITH_KNOTS ( ( 4, 2, 2, 2, 2, 2, 4 ),
 ( 3, 3 ),
 ( 0.000000000000000000, 0.0009440840677143813933, 0.001416126101571572090, 0.001888168135428762787, 0.002360210169285953483, 0.002832252203143144180, 0.003776336270857525573 ),
 ( 0.000000000000000000, 1.000000000000000000 ),
 .UNSPECIFIED. ) 
 GEOMETRIC_REPRESENTATION_ITEM ( )  RATIONAL_B_SPLINE_SURFACE ( (
 ( 1.000000000000000000, 0.8070209408750133040, 1.000000000000000000),
 ( 1.000000000000000000, 0.8215603905301913645, 1.000000000000000000),
 ( 1.000000000000000000, 0.8340988699037210630, 1.000000000000000000),
 ( 1.000000000000000000, 0.8516751610470432166, 1.000000000000000000),
 ( 1.000000000000000000, 0.8573697395158472734, 1.000000000000000000),
 ( 1.000000000000000000, 0.8683586635657976061, 1.000000000000000000),
 ( 1.000000000000000000, 0.8736518481707038486, 1.000000000000000000),
 ( 1.000000000000000000, 0.8840377753031671837, 1.000000000000000000),
 ( 1.000000000000000000, 0.8891294171305078597, 1.000000000000000000),
 ( 1.000000000000000000, 0.8992456600575245984, 1.000000000000000000),
 ( 1.000000000000000000, 0.9042785869232097262, 1.000000000000000000),
 ( 1.000000000000000000, 0.9189749222880136958, 1.000000000000000000),
 ( 1.000000000000000000, 0.9283978182317160766, 1.000000000000000000),
 ( 1.000000000000000000, 0.9376006582765968878, 1.000000000000000000) ) ) 
 REPRESENTATION_ITEM ( '' )  SURFACE ( )  );
#87163=CARTESIAN_POINT ( 'NONE',  ( -20.49599333844833993, 1525.960063244516959, 233.8638087104925489 ) ) ;
#87165=CARTESIAN_POINT ( 'NONE',  ( -28.44685754529687571, 1526.382868172863937, 219.8746262742137105 ) ) ;
#87166=EDGE_CURVE ( 'NONE', #23656, #84410, #34993, .T. ) ;
#87191=ORIENTED_EDGE ( 'NONE', *, *, #79152, .F. ) ;
#87196=ORIENTED_EDGE ( 'NONE', *, *, #57599, .T. ) ;
#87198=CARTESIAN_POINT ( 'NONE',  ( 30.60906614450638230, 1526.073434386619738, 201.6841089170558519 ) ) ;
#87202=ADVANCED_FACE ( 'NONE', ( #3745 ), #54698, .T. ) ;
#87213=AXIS2_PLACEMENT_3D ( 'NONE', #102734, #17059, #104418 ) ;
#87223=DIRECTION ( 'NONE',  ( -0.9510565162951566398, 0.000000000000000000, -0.3090169943749382919 ) ) ;
#87233=DIRECTION ( 'NONE',  ( 0.000000000000000000, 1.000000000000000000, 0.000000000000000000 ) ) ;
#87234=EDGE_LOOP ( 'NONE', ( #78378, #91123, #79315, #22745 ) ) ;
#87244=CARTESIAN_POINT ( 'NONE',  ( 76.99707197884903564, 1524.382868172863937, 19.35599459046138193 ) ) ;
#87253=DIRECTION ( 'NONE',  ( 0.000000000000000000, 1.000000000000000000, 0.000000000000000000 ) ) ;
#87273=ORIENTED_EDGE ( 'NONE', *, *, #70687, .T. ) ;
#87276=DIRECTION ( 'NONE',  ( 0.000000000000000000, -1.000000000000000000, 0.000000000000000000 ) ) ;
#87287=VECTOR ( 'NONE', #37074, 1000.000000000000000 ) ;
#87289=CARTESIAN_POINT ( 'NONE',  ( 2.458536830555473340, 1524.871836253796118, 242.3417002918415903 ) ) ;
#87292=CARTESIAN_POINT ( 'NONE',  ( 22.69876404240100243, 1522.382868172863937, 236.8953202675778869 ) ) ;
#87309=CARTESIAN_POINT ( 'NONE',  ( 17.17241001986483795, 1511.187213306747708, 181.6185504016043240 ) ) ;
#87311=CARTESIAN_POINT ( 'NONE',  ( -1.191524307911306479, 1526.382868172864164, 239.2353018730791518 ) ) ;
#87328=FACE_OUTER_BOUND ( 'NONE', #875, .T. ) ;
#87341=ADVANCED_FACE ( 'NONE', ( #22133 ), #42202, .F. ) ;
#87350=ADVANCED_FACE ( 'NONE', ( #34973 ), #26569, .T. ) ;
#87355=CARTESIAN_POINT ( 'NONE',  ( -33.82780500856123496, 1523.429859730330918, 220.5611772381400328 ) ) ;
#87357=CARTESIAN_POINT ( 'NONE',  ( 32.13439773946879541, 1525.163527997504389, 201.2154464867858792 ) ) ;
#87365=AXIS2_PLACEMENT_3D ( 'NONE', #26047, #93271, #60240 ) ;
#87366=CARTESIAN_POINT ( 'NONE',  ( -2.493583506516910298, 1524.152349020271004, 175.5218085340932532 ) ) ;
#87392=VERTEX_POINT ( 'NONE', #83725 ) ;
#87397=AXIS2_PLACEMENT_3D ( 'NONE', #39600, #82703, #74326 ) ;
#87400=CARTESIAN_POINT ( 'NONE',  ( 2.038646110889675178, 1525.960063244516959, 241.1857569150893994 ) ) ;
#87413=FACE_OUTER_BOUND ( 'NONE', #76349, .T. ) ;
#87430=VECTOR ( 'NONE', #19907, 1000.000000000000000 ) ;
#87435=DIRECTION ( 'NONE',  ( -0.000000000000000000, -1.000000000000000000, -0.000000000000000000 ) ) ;
#87436=CARTESIAN_POINT ( 'NONE',  ( 0.000000000000000000, 1518.913060387330006, 209.1218459616979999 ) ) ;
#87447=DIRECTION ( 'NONE',  ( 0.000000000000000000, 0.000000000000000000, 1.000000000000000000 ) ) ;
#87453=AXIS2_PLACEMENT_3D ( 'NONE', #87507, #46621, #10796 ) ;
#87455=CARTESIAN_POINT ( 'NONE',  ( -33.17484411121681376, 1525.713797967456912, 217.3801513758764088 ) ) ;
#87470=ADVANCED_FACE ( 'NONE', ( #110582 ), #88655, .F. ) ;
#87478=CARTESIAN_POINT ( 'NONE',  ( -34.77865709046010778, 1512.187213306747481, 191.3609956664894014 ) ) ;
#87479=B_SPLINE_CURVE_WITH_KNOTS ( 'NONE', 3,
 ( #52910, #35532, #8661, #26004, #69726, #17598, #104396, #70842 ),
 .UNSPECIFIED., .F., .F.,
 ( 4, 2, 2, 4 ),
 ( 2.428612866367529932E-17, 0.001073044933456048563, 0.001609567400184060701, 0.002146089866912072840 ),
 .UNSPECIFIED. ) ;
#87481=CARTESIAN_POINT ( 'NONE',  ( -30.00389853323245148, 1524.843416604514459, 195.9693362516085244 ) ) ;
#87501=DIRECTION ( 'NONE',  ( 0.000000000000000000, 0.000000000000000000, -1.000000000000000000 ) ) ;
#87507=CARTESIAN_POINT ( 'NONE',  ( -32.28466283162143213, 1501.977400791986611, 219.1752493337717738 ) ) ;
#87521=CARTESIAN_POINT ( 'NONE',  ( 18.97796697799407539, 1526.382868172864164, 185.2752177337489172 ) ) ;
#87529=CARTESIAN_POINT ( 'NONE',  ( 31.81407709660777527, 1512.187213306747481, 221.9534378623329758 ) ) ;
#87534=DIRECTION ( 'NONE',  ( 0.8672669759446666182, -0.000000000000000000, 0.4978433412588672557 ) ) ;
#87540=EDGE_LOOP ( 'NONE', ( #20718, #82995, #97157, #39100 ) ) ;
#87553=EDGE_LOOP ( 'NONE', ( #25798, #33091, #850, #58759, #42937 ) ) ;
#87576=CARTESIAN_POINT ( 'NONE',  ( 30.98807061075474323, 1524.600389084707103, 221.8038906437711262 ) ) ;
#87582=CARTESIAN_POINT ( 'NONE',  ( -16.92737646175572763, 1525.317359687823455, 236.7941014278637226 ) ) ;
#87597=CARTESIAN_POINT ( 'NONE',  ( 28.44685754529808719, 1526.382868172863937, 198.3690656491830850 ) ) ;
#87610=AXIS2_PLACEMENT_3D ( 'NONE', #16285, #50489, #42076 ) ;
#87616=CARTESIAN_POINT ( 'NONE',  ( -32.99911596133329539, 1524.244163922423695, 196.1627191131780705 ) ) ;
#87645=ORIENTED_EDGE ( 'NONE', *, *, #74798, .F. ) ;
#87653=CARTESIAN_POINT ( 'NONE',  ( -31.32941717379338797, 1525.856064936177972, 201.1886153483195301 ) ) ;
#87687=CIRCLE ( 'NONE', #21460, 1.000000000000007772 ) ;
#87692=CARTESIAN_POINT ( 'NONE',  ( 19.29371659517364890, 1526.349689584397083, 233.1523940083487219 ) ) ;
#87700=CARTESIAN_POINT ( 'NONE',  ( -30.38288201977564285, 1524.477587234266139, 221.8420718908230356 ) ) ;
#87728=EDGE_CURVE ( 'NONE', #89419, #66077, #23680, .T. ) ;
#87730=CARTESIAN_POINT ( 'NONE',  ( -21.84020450222076093, 1523.481610426287716, 183.2638850454220858 ) ) ;
#87733=CARTESIAN_POINT ( 'NONE',  ( -32.92528853941070821, 1523.611961620354123, 201.0067946816169240 ) ) ;
#87751=CARTESIAN_POINT ( 'NONE',  ( 29.30029655192931415, 1525.907212628473872, 221.3719603026171399 ) ) ;
#87760=ORIENTED_EDGE ( 'NONE', *, *, #35110, .T. ) ;
#87766=EDGE_LOOP ( 'NONE', ( #109587, #64780, #102654, #108783 ) ) ;
#87772=FACE_OUTER_BOUND ( 'NONE', #64399, .T. ) ;
#87783=DIRECTION ( 'NONE',  ( 0.000000000000000000, -1.000000000000000000, 0.000000000000000000 ) ) ;
#87791=CARTESIAN_POINT ( 'NONE',  ( 49.24962907673571522, 1524.382868172863937, 407.9033880519289710 ) ) ;
#87804=ORIENTED_EDGE ( 'NONE', *, *, #52202, .T. ) ;
#87827=ORIENTED_EDGE ( 'NONE', *, *, #97353, .F. ) ;
#87828=ORIENTED_EDGE ( 'NONE', *, *, #59735, .F. ) ;
#87830=EDGE_CURVE ( 'NONE', #19317, #16710, #84685, .T. ) ;
#87832=CARTESIAN_POINT ( 'NONE',  ( -22.08622291482313926, 1523.382868172864164, 233.8253038720786776 ) ) ;
#87879=AXIS2_PLACEMENT_3D ( 'NONE', #59658, #61884, #9248 ) ;
#87880=CARTESIAN_POINT ( 'NONE',  ( -1.389373685231614308, 1526.382868172571079, 239.5386865367401299 ) ) ;
#87899=VECTOR ( 'NONE', #37193, 1000.000000000000000 ) ;
#87913=AXIS2_PLACEMENT_3D ( 'NONE', #52374, #76442, #67517 ) ;
#87923=CARTESIAN_POINT ( 'NONE',  ( -30.79697748855893735, 1526.178928173327449, 221.8439766881946014 ) ) ;
#87925=CARTESIAN_POINT ( 'NONE',  ( 32.05679137160524306, 1524.478200376950781, 201.5541812493231077 ) ) ;
#87945=ADVANCED_FACE ( 'NONE', ( #28522 ), #3649, .T. ) ;
#87951=ADVANCED_FACE ( 'NONE', ( #87328 ), #73615, .F. ) ;
#87957=ADVANCED_FACE ( 'NONE', ( #56487 ), #21182, .T. ) ;
#87959=CIRCLE ( 'NONE', #61124, 23.69926344187880929 ) ;
#87963=EDGE_CURVE ( 'NONE', #5224, #54639, #31269, .T. ) ;
#87976=VERTEX_POINT ( 'NONE', #90061 ) ;
#88004=AXIS2_PLACEMENT_3D ( 'NONE', #17210, #110758, #67679 ) ;
#88006=ORIENTED_EDGE ( 'NONE', *, *, #55075, .F. ) ;
#88013=LINE ( 'NONE', #62265, #91402 ) ;
#88033=CARTESIAN_POINT ( 'NONE',  ( -32.37018134260392088, 1512.187213306747481, 218.0712926453366833 ) ) ;
#88041=CARTESIAN_POINT ( 'NONE',  ( -29.30029655192950244, 1525.907212628473644, 196.8717316207788315 ) ) ;
#88043=CARTESIAN_POINT ( 'NONE',  ( 20.39893125377741612, 1526.069472839382115, 233.1323736274815701 ) ) ;
#88047=DIRECTION ( 'NONE',  ( 0.000000000000000000, 0.000000000000000000, -1.000000000000000000 ) ) ;
#88056=LINE ( 'NONE', #72356, #28266 ) ;
#88069=FACE_OUTER_BOUND ( 'NONE', #42583, .T. ) ;
#88071=AXIS2_PLACEMENT_3D ( 'NONE', #9339, #75986, #33976 ) ;
#88075=ORIENTED_EDGE ( 'NONE', *, *, #15689, .F. ) ;
#88076=ORIENTED_EDGE ( 'NONE', *, *, #88332, .F. ) ;
#88079=CARTESIAN_POINT ( 'NONE',  ( 20.49599333844834348, 1525.960063244517187, 184.3798832129035077 ) ) ;
#88134=CARTESIAN_POINT ( 'NONE',  ( 29.79244516856374858, 1525.556089352344770, 221.4002000438143511 ) ) ;
#88137=CARTESIAN_POINT ( 'NONE',  ( -16.86500412379770708, 1525.697946996610881, 236.3931742940298193 ) ) ;
#88161=CARTESIAN_POINT ( 'NONE',  ( 3.448830483803564828, 1512.187213306747481, 243.0842028158767789 ) ) ;
#88162=ORIENTED_EDGE ( 'NONE', *, *, #55256, .F. ) ;
#88168=CARTESIAN_POINT ( 'NONE',  ( -33.93019615849274828, 1522.906561336852974, 197.6607374646097810 ) ) ;
#88177=ORIENTED_EDGE ( 'NONE', *, *, #79257, .T. ) ;
#88201=CARTESIAN_POINT ( 'NONE',  ( -31.88715249297895227, 1525.425686270224560, 201.2219484344741147 ) ) ;
#88202=FACE_OUTER_BOUND ( 'NONE', #34401, .T. ) ;
#88210=ORIENTED_EDGE ( 'NONE', *, *, #99506, .T. ) ;
#88213=ORIENTED_EDGE ( 'NONE', *, *, #73718, .F. ) ;
#88236=CARTESIAN_POINT ( 'NONE',  ( 18.66420869458061205, 1526.382868172863937, 232.7837831374278039 ) ) ;
#88242=CARTESIAN_POINT ( 'NONE',  ( -31.16645442585705084, 1524.201670966335314, 221.8713816554661094 ) ) ;
#88268=UNCERTAINTY_MEASURE_WITH_UNIT (LENGTH_MEASURE( 1.000000000000000082E-05 ), #2428, 'distance_accuracy_value', 'NONE');
#88273=CARTESIAN_POINT ( 'NONE',  ( 34.18677586421181758, 1522.382868172863937, 198.4504086008745389 ) ) ;
#88274=CARTESIAN_POINT ( 'NONE',  ( 17.30126322264720429, 1523.462669333491704, 180.8506073315129470 ) ) ;
#88281=DIRECTION ( 'NONE',  ( 0.000000000000000000, 0.000000000000000000, 1.000000000000000000 ) ) ;
#88301=ORIENTED_EDGE ( 'NONE', *, *, #36336, .T. ) ;
#88309=DIRECTION ( 'NONE',  ( -0.8090169943749422332, 0.000000000000000000, 0.5877852522924802425 ) ) ;
#88318=CARTESIAN_POINT ( 'NONE',  ( 3.304926999371979868, 1524.538969332612623, 241.8712028721135994 ) ) ;
#88332=EDGE_CURVE ( 'NONE', #91721, #105303, #84101, .T. ) ;
#88344=AXIS2_PLACEMENT_3D ( 'NONE', #63736, #82715, #40156 ) ;
#88348=CARTESIAN_POINT ( 'NONE',  ( 173.8335085727406693, 1524.382868172863937, 317.3879012941853830 ) ) ;
#88358=CARTESIAN_POINT ( 'NONE',  ( 0.000000000000000000, 1518.913060387330006, 209.1218459616979999 ) ) ;
#88366=VECTOR ( 'NONE', #4876, 1000.000000000000000 ) ;
#88387=ADVANCED_FACE ( 'NONE', ( #30998 ), #80124, .F. ) ;
#88389=ADVANCED_FACE ( 'NONE', ( #107714 ), #49475, .T. ) ;
#88391=CARTESIAN_POINT ( 'NONE',  ( 2.478666945488134932, 1524.659148609483054, 242.4727585245961450 ) ) ;
#88400=LINE ( 'NONE', #104646, #89629 ) ;
#88408=CARTESIAN_POINT ( 'NONE',  ( -2.857351367441036238, 1525.661276915132476, 177.1476448543304514 ) ) ;
#88409=CARTESIAN_POINT ( 'NONE',  ( 0.000000000000000000, 1526.382868172863937, 242.2588656733921653 ) ) ;
#88410=CARTESIAN_POINT ( 'NONE',  ( -2.038646110889581031, 1525.960063244516959, 241.1857569150894562 ) ) ;
#88412=ADVANCED_FACE ( 'NONE', ( #65176 ), #14, .F. ) ;
#88416=CARTESIAN_POINT ( 'NONE',  ( -16.85976061912537816, 1525.821544997590536, 236.1944305375348847 ) ) ;
#88419=EDGE_CURVE ( 'NONE', #89436, #43690, #24777, .T. ) ;
#88443=CIRCLE ( 'NONE', #86839, 1.000000000000000888 ) ;
#88448=EDGE_CURVE ( 'NONE', #43187, #81049, #75230, .T. ) ;
#88457=CARTESIAN_POINT ( 'NONE',  ( -33.43367350703635310, 1524.397344074318198, 220.4773507679704494 ) ) ;
#88459=CARTESIAN_POINT ( 'NONE',  ( 31.75407494088092264, 1525.055427061254250, 201.5867930770752423 ) ) ;
#88467=DIRECTION ( 'NONE',  ( 0.000000000000000000, 0.000000000000000000, 1.000000000000000000 ) ) ;
#88474=VERTEX_POINT ( 'NONE', #34306 ) ;
#88475=DIRECTION ( 'NONE',  ( 0.000000000000000000, 0.000000000000000000, 1.000000000000000000 ) ) ;
#88478=DIRECTION ( 'NONE',  ( 0.000000000000000000, 1.000000000000000000, 0.000000000000000000 ) ) ;
#88502=VERTEX_POINT ( 'NONE', #728 ) ;
#88519=CARTESIAN_POINT ( 'NONE',  ( -30.31052258194604576, 1523.604703353109699, 195.7506062427372058 ) ) ;
#88536=CARTESIAN_POINT ( 'NONE',  ( 32.02808312589916540, 1512.187213306747481, 198.2787714533495489 ) ) ;
#88548=CIRCLE ( 'NONE', #59942, 2.000000000000001776 ) ;
#88566=DIRECTION ( 'NONE',  ( 0.2054769195713317398, -1.225281874271768203E-16, 0.9786619618251628516 ) ) ;
#88575=EDGE_LOOP ( 'NONE', ( #54133, #3568, #6691, #95447 ) ) ;
#88578=FACE_OUTER_BOUND ( 'NONE', #99737, .T. ) ;
#88590=DIRECTION ( 'NONE',  ( -0.000000000000000000, -1.000000000000000000, 0.000000000000000000 ) ) ;
#88593=CARTESIAN_POINT ( 'NONE',  ( 1.191524307911311364, 1526.382868172864164, 179.0083900503168479 ) ) ;
#88612=EDGE_CURVE ( 'NONE', #7480, #108583, #39420, .T. ) ;
#88640=FACE_OUTER_BOUND ( 'NONE', #79140, .T. ) ;
#88645=ORIENTED_EDGE ( 'NONE', *, *, #39541, .F. ) ;
#88655=( BOUNDED_SURFACE ( )  B_SPLINE_SURFACE ( 3, 2, ( 
 ( #34429, #25451, #50148 ),
 ( #16490, #42278, #58544 ),
 ( #67503, #49593, #92670 ),
 ( #7571, #50680, #84812 ),
 ( #84275, #8111, #9237 ),
 ( #93755, #76429, #102169 ),
 ( #103260, #33867, #41725 ),
 ( #110033, #17032, #68058 ),
 ( #51230, #85363, #94316 ),
 ( #102705, #75885, #68602 ),
 ( #8658, #76996, #96551 ),
 ( #9775, #44499, #71392 ),
 ( #106054, #43941, #11447 ),
 ( #71941, #54031, #18710 ) ),
 .UNSPECIFIED., .F., .F., .F. ) 
 B_SPLINE_SURFACE_WITH_KNOTS ( ( 4, 2, 2, 2, 2, 2, 4 ),
 ( 3, 3 ),
 ( 3.068292148133977548E-17, 0.0009443072508235996528, 0.001416460876235384192, 0.001888614501647168731, 0.002360768127058953270, 0.002832921752470737593, 0.003777229003294306671 ),
 ( 0.000000000000000000, 1.000000000000000000 ),
 .UNSPECIFIED. ) 
 GEOMETRIC_REPRESENTATION_ITEM ( )  RATIONAL_B_SPLINE_SURFACE ( (
 ( 1.000000000000000000, 0.9376006582765952224, 1.000000000000000000),
 ( 1.000000000000000000, 0.9283977714737551290, 1.000000000000000000),
 ( 1.000000000000000000, 0.9189750060478811822, 1.000000000000000000),
 ( 1.000000000000000000, 0.9042792056128057254, 1.000000000000000000),
 ( 1.000000000000000000, 0.8992469033844706638, 1.000000000000000000),
 ( 1.000000000000000000, 0.8891280264680628820, 1.000000000000000000),
 ( 1.000000000000000000, 0.8840337471674211134, 1.000000000000000000),
 ( 1.000000000000000000, 0.8736395124164628712, 1.000000000000000000),
 ( 1.000000000000000000, 0.8683406746553720135, 1.000000000000000000),
 ( 1.000000000000000000, 0.8573361860706717463, 1.000000000000000000),
 ( 1.000000000000000000, 0.8516508399495776871, 1.000000000000000000),
 ( 1.000000000000000000, 0.8340914917066705181, 1.000000000000000000),
 ( 1.000000000000000000, 0.8215597275861525883, 1.000000000000000000),
 ( 1.000000000000000000, 0.8070209408750226299, 1.000000000000000000) ) ) 
 REPRESENTATION_ITEM ( '' )  SURFACE ( )  );
#88657=ORIENTED_EDGE ( 'NONE', *, *, #95210, .T. ) ;
#88676=CARTESIAN_POINT ( 'NONE',  ( -2.493590731671294414, 1524.152444737676660, 242.7218577030689062 ) ) ;
#88680=AXIS2_PLACEMENT_3D ( 'NONE', #54548, #19798, #11422 ) ;
#88682=DIRECTION ( 'NONE',  ( -1.000000000000000000, 0.000000000000000000, 0.000000000000000000 ) ) ;
#88685=CARTESIAN_POINT ( 'NONE',  ( -16.49279160078807038, 1525.408337840050763, 236.9553505360240138 ) ) ;
#88703=CARTESIAN_POINT ( 'NONE',  ( 22.08622291482350519, 1512.187213306747481, 233.8253038720783366 ) ) ;
#88704=EDGE_CURVE ( 'NONE', #97242, #66900, #43464, .T. ) ;
#88705=CARTESIAN_POINT ( 'NONE',  ( -20.39146254758225751, 1526.073434386618828, 233.1306592966913627 ) ) ;
#88706=CARTESIAN_POINT ( 'NONE',  ( -30.31940284292399213, 1523.456872492435195, 222.4933038710547919 ) ) ;
#88708=EDGE_CURVE ( 'NONE', #101252, #30502, #34141, .T. ) ;
#88733=CARTESIAN_POINT ( 'NONE',  ( -17.17241001986523941, 1511.187213306747708, 181.6185504016045797 ) ) ;
#88763=CARTESIAN_POINT ( 'NONE',  ( 21.78062404853721290, 1524.843178112496162, 233.5929681532350912 ) ) ;
#88764=ORIENTED_EDGE ( 'NONE', *, *, #27652, .F. ) ;
#88765=ORIENTED_EDGE ( 'NONE', *, *, #8057, .T. ) ;
#88766=CARTESIAN_POINT ( 'NONE',  ( -33.93019615848938741, 1522.382868172863937, 220.5829544587966211 ) ) ;
#88774=AXIS2_PLACEMENT_3D ( 'NONE', #79494, #27414, #95730 ) ;
#88802=LINE ( 'NONE', #72563, #47538 ) ;
#88806=CARTESIAN_POINT ( 'NONE',  ( 21.83863729848984292, 1523.580204110584418, 183.2673815993468054 ) ) ;
#88809=ORIENTED_EDGE ( 'NONE', *, *, #38387, .F. ) ;
#88814=CIRCLE ( 'NONE', #51312, 0.9999999999999975575 ) ;
#88824=CARTESIAN_POINT ( 'NONE',  ( -34.18677586421173942, 1524.726013923371283, 219.7932833225216882 ) ) ;
#88826=CARTESIAN_POINT ( 'NONE',  ( 2.038847259689227531, 1522.382868172863937, 244.9330574173806667 ) ) ;
#88828=ORIENTED_EDGE ( 'NONE', *, *, #23589, .T. ) ;
#88833=DIRECTION ( 'NONE',  ( -0.000000000000000000, -1.000000000000000000, -0.000000000000000000 ) ) ;
#88873=B_SPLINE_CURVE_WITH_KNOTS ( 'NONE', 3,
 ( #43491, #1487, #93858, #33965 ),
 .UNSPECIFIED., .F., .F.,
 ( 4, 4 ),
 ( 0.000000000000000000, 0.0002960034161023854899 ),
 .UNSPECIFIED. ) ;
#88886=CARTESIAN_POINT ( 'NONE',  ( 0.000000000000000000, 1522.382868172863937, 240.9330574173806951 ) ) ;
#88889=DIRECTION ( 'NONE',  ( 0.3090169943749654369, -2.144236138472418401E-15, 0.9510565162951478690 ) ) ;
#88898=DIRECTION ( 'NONE',  ( -0.9125304618754029873, 0.000000000000000000, -0.4090087482554177756 ) ) ;
#88909=CARTESIAN_POINT ( 'NONE',  ( 2.407253779970412566, 1523.313115944345554, 175.0653106450178882 ) ) ;
#88955=CARTESIAN_POINT ( 'NONE',  ( -16.81049281787982252, 1526.143142182167367, 235.5964692618745175 ) ) ;
#88963=CARTESIAN_POINT ( 'NONE',  ( 31.10385014139599136, 1525.795403383247276, 216.3488197230036860 ) ) ;
#88986=ORIENTED_EDGE ( 'NONE', *, *, #43319, .F. ) ;
#88994=FACE_OUTER_BOUND ( 'NONE', #1127, .T. ) ;
#89002=CARTESIAN_POINT ( 'NONE',  ( 0.000000000000000000, 1518.913060387330006, 179.0139814193315999 ) ) ;
#89003=CARTESIAN_POINT ( 'NONE',  ( 30.79916350760221277, 1526.104292489146474, 201.1259370313290731 ) ) ;
#89008=ORIENTED_EDGE ( 'NONE', *, *, #95837, .T. ) ;
#89028=ORIENTED_EDGE ( 'NONE', *, *, #63312, .T. ) ;
#89033=CARTESIAN_POINT ( 'NONE',  ( 17.12202622828785792, 1526.104292489130330, 235.9427193670906320 ) ) ;
#89039=ORIENTED_EDGE ( 'NONE', *, *, #27652, .T. ) ;
#89041=ORIENTED_EDGE ( 'NONE', *, *, #67878, .T. ) ;
#89047=FACE_OUTER_BOUND ( 'NONE', #22882, .T. ) ;
#89048=EDGE_CURVE ( 'NONE', #29269, #39549, #12647, .T. ) ;
#89051=EDGE_CURVE ( 'NONE', #82365, #100321, #626, .T. ) ;
#89068=DIRECTION ( 'NONE',  ( 0.000000000000000000, 1.000000000000000000, 0.000000000000000000 ) ) ;
#89078=DIRECTION ( 'NONE',  ( -0.9125304618753961039, 0.000000000000000000, 0.4090087482554332632 ) ) ;
#89089=CARTESIAN_POINT ( 'NONE',  ( -20.38673671613199545, 1525.878013734321939, 236.1208636900185525 ) ) ;
#89115=CARTESIAN_POINT ( 'NONE',  ( -29.95988583836330221, 1525.317349363550193, 196.6841769033301546 ) ) ;
#89116=CIRCLE ( 'NONE', #21145, 1.000000000000004441 ) ;
#89117=CARTESIAN_POINT ( 'NONE',  ( -16.66936639838851875, 1523.456924617339610, 237.7608804993614910 ) ) ;
#89123=AXIS2_PLACEMENT_3D ( 'NONE', #73152, #107296, #67524 ) ;
#89126=CARTESIAN_POINT ( 'NONE',  ( 2.273033093151324735, 1525.821544997590536, 177.3097463090895189 ) ) ;
#89127=DIRECTION ( 'NONE',  ( 0.000000000000000000, 1.000000000000000000, 0.000000000000000000 ) ) ;
#89128=ORIENTED_EDGE ( 'NONE', *, *, #26874, .T. ) ;
#89130=AXIS2_PLACEMENT_3D ( 'NONE', #24726, #25836, #60036 ) ;
#89135=FACE_OUTER_BOUND ( 'NONE', #36547, .T. ) ;
#89173=EDGE_CURVE ( 'NONE', #83952, #106220, #66309, .T. ) ;
#89176=ORIENTED_EDGE ( 'NONE', *, *, #63832, .T. ) ;
#89193=CARTESIAN_POINT ( 'NONE',  ( 3.448830483803564828, 1511.187213306747708, 243.0842028158767789 ) ) ;
#89204=DIRECTION ( 'NONE',  ( 0.000000000000000000, 0.000000000000000000, 1.000000000000000000 ) ) ;
#89222=CARTESIAN_POINT ( 'NONE',  ( 29.71163624023450467, 1526.333389947941441, 217.1029916164621909 ) ) ;
#89225=CARTESIAN_POINT ( 'NONE',  ( 16.75454338844407687, 1526.382868173645875, 183.6974516591938880 ) ) ;
#89227=CARTESIAN_POINT ( 'NONE',  ( -6.144376325710156905, 1512.187213306747481, 247.6867189913431844 ) ) ;
#89272=EDGE_CURVE ( 'NONE', #42124, #49270, #88873, .T. ) ;
#89310=CIRCLE ( 'NONE', #92887, 2.000000000000001776 ) ;
#89312=DIRECTION ( 'NONE',  ( -0.9786619618251657382, 0.000000000000000000, 0.2054769195713179730 ) ) ;
#89323=EDGE_CURVE ( 'NONE', #73846, #32838, #46272, .T. ) ;
#89325=ORIENTED_EDGE ( 'NONE', *, *, #92098, .F. ) ;
#89359=EDGE_CURVE ( 'NONE', #54701, #40948, #83497, .T. ) ;
#89362=AXIS2_PLACEMENT_3D ( 'NONE', #85922, #104380, #79201 ) ;
#89382=CARTESIAN_POINT ( 'NONE',  ( -17.22845748920260434, 1525.848198008145346, 236.4819726785932517 ) ) ;
#89386=CARTESIAN_POINT ( 'NONE',  ( -2.664527636416262890, 1524.964230758899930, 241.7075690384371569 ) ) ;
#89398=AXIS2_PLACEMENT_3D ( 'NONE', #27444, #28556, #88467 ) ;
#89399=FACE_OUTER_BOUND ( 'NONE', #90958, .T. ) ;
#89402=ORIENTED_EDGE ( 'NONE', *, *, #79152, .T. ) ;
#89417=CARTESIAN_POINT ( 'NONE',  ( 31.97190655716449115, 1524.330813522192102, 201.5540712235606975 ) ) ;
#89419=VERTEX_POINT ( 'NONE', #82029 ) ;
#89421=DIRECTION ( 'NONE',  ( -0.000000000000000000, -1.000000000000000000, -0.000000000000000000 ) ) ;
#89426=FACE_OUTER_BOUND ( 'NONE', #83672, .T. ) ;
#89431=( BOUNDED_CURVE ( )  B_SPLINE_CURVE ( 3, ( #14915, #105833, #20684, #11757 ),
 .UNSPECIFIED., .F., .T. ) 
 B_SPLINE_CURVE_WITH_KNOTS ( ( 4, 4 ),
 ( 0.000000000000000000, 0.7048113239778114325 ),
 .UNSPECIFIED. ) 
 CURVE ( )  GEOMETRIC_REPRESENTATION_ITEM ( )  RATIONAL_B_SPLINE_CURVE ( ( 1.000000000000000000, 0.9590300661663084814, 0.9590300661663084814, 1.000000000000000000 ) ) 
 REPRESENTATION_ITEM ( '' )  );
#89436=VERTEX_POINT ( 'NONE', #41694 ) ;
#89438=VERTEX_POINT ( 'NONE', #31080 ) ;
#89439=EDGE_LOOP ( 'NONE', ( #83151, #15495, #56490 ) ) ;
#89470=ORIENTED_EDGE ( 'NONE', *, *, #106519, .F. ) ;
#89475=CIRCLE ( 'NONE', #62745, 33.13701971169416538 ) ;
#89496=CIRCLE ( 'NONE', #55552, 1.000000000000002442 ) ;
#89505=CARTESIAN_POINT ( 'NONE',  ( -17.83486663330526767, 1523.678648413191695, 180.3677388339002334 ) ) ;
#89506=DIRECTION ( 'NONE',  ( -0.000000000000000000, -1.000000000000000000, -0.000000000000000000 ) ) ;
#89508=TOROIDAL_SURFACE ( 'NONE', #69888, 30.13701971169416538, 3.000000000000000000 ) ;
#89521=DIRECTION ( 'NONE',  ( -0.4978433412588676998, 0.000000000000000000, 0.8672669759446663962 ) ) ;
#89526=CIRCLE ( 'NONE', #41256, 33.13701971169416538 ) ;
#89531=DIRECTION ( 'NONE',  ( 0.9510565162951564178, 0.000000000000000000, 0.3090169943749387915 ) ) ;
#89542=CARTESIAN_POINT ( 'NONE',  ( 17.89234610336740516, 1523.611961620354123, 237.9279674222333369 ) ) ;
#89574=CARTESIAN_POINT ( 'NONE',  ( -32.02808312589930040, 1512.187213306747481, 197.2787714533499752 ) ) ;
#89586=CARTESIAN_POINT ( 'NONE',  ( 16.89460221416486618, 1526.348417187218047, 234.9076154478274248 ) ) ;
#89597=CARTESIAN_POINT ( 'NONE',  ( 2.425477467416652377, 1523.390106123591067, 175.1521078860171770 ) ) ;
#89624=CARTESIAN_POINT ( 'NONE',  ( 16.48487881372698638, 1525.795403621570358, 236.4701071512044166 ) ) ;
#89629=VECTOR ( 'NONE', #10034, 1000.000000000000000 ) ;
#89634=CARTESIAN_POINT ( 'NONE',  ( -22.01290455779406940, 1522.906363951597314, 235.3651141902285815 ) ) ;
#89639=AXIS2_PLACEMENT_3D ( 'NONE', #20367, #54573, #78082 ) ;
#89668=CARTESIAN_POINT ( 'NONE',  ( -30.79106905599208588, 1526.107880201381477, 201.1252782592679864 ) ) ;
#89670=ORIENTED_EDGE ( 'NONE', *, *, #76306, .T. ) ;
#89688=DIRECTION ( 'NONE',  ( -0.2054769195713296581, 0.000000000000000000, -0.9786619618251632957 ) ) ;
#89709=CIRCLE ( 'NONE', #30713, 0.9999999999999975575 ) ;
#89720=ORIENTED_EDGE ( 'NONE', *, *, #110571, .T. ) ;
#89726=CARTESIAN_POINT ( 'NONE',  ( 32.52439779765787620, 1524.599984580802129, 217.0762361364453454 ) ) ;
#89729=VECTOR ( 'NONE', #49163, 1000.000000000000000 ) ;
#89741=CARTESIAN_POINT ( 'NONE',  ( -31.41104781486826880, 1511.187213306747708, 202.3296363711539527 ) ) ;
#89747=DIRECTION ( 'NONE',  ( 0.4978433412588755269, 0.000000000000000000, 0.8672669759446619553 ) ) ;
#89762=CARTESIAN_POINT ( 'NONE',  ( 29.67375891017061917, 1525.697947650418428, 221.2718125036566335 ) ) ;
#89769=CARTESIAN_POINT ( 'NONE',  ( -31.34137657934026677, 1523.481610426287716, 196.3411265156551906 ) ) ;
#89772=EDGE_CURVE ( 'NONE', #10960, #92224, #103848, .T. ) ;
#89780=EDGE_CURVE ( 'NONE', #66077, #40683, #78847, .T. ) ;
#89783=CARTESIAN_POINT ( 'NONE',  ( -32.28466283162143213, 1512.187213306747481, 219.1752493337717738 ) ) ;
#89785=CIRCLE ( 'NONE', #36091, 1.000000000000000888 ) ;
#89805=CARTESIAN_POINT ( 'NONE',  ( 32.79520279072050215, 1523.954914175595377, 217.1622232076301771 ) ) ;
#89809=EDGE_CURVE ( 'NONE', #47286, #96482, #102070, .T. ) ;
#89815=CARTESIAN_POINT ( 'NONE',  ( -20.49599333844833993, 1525.960063244516959, 233.8638087104925489 ) ) ;
#89825=DIRECTION ( 'NONE',  ( 1.734723475976805517E-14, 0.000000000000000000, 1.000000000000000000 ) ) ;
#89836=PLANE ( 'NONE',  #90401 ) ;
#89842=( NAMED_UNIT ( * ) SI_UNIT ( $, .STERADIAN. ) SOLID_ANGLE_UNIT ( ) );
#89882=CARTESIAN_POINT ( 'NONE',  ( -30.41976661596593345, 1524.374142163904025, 221.8533802443857894 ) ) ;
#89888=VERTEX_POINT ( 'NONE', #53156 ) ;
#89910=ADVANCED_FACE ( 'NONE', ( #106295 ), #56451, .F. ) ;
#89913=CARTESIAN_POINT ( 'NONE',  ( -30.31940284292427634, 1512.187213306747481, 195.7503880523418616 ) ) ;
#89918=CARTESIAN_POINT ( 'NONE',  ( 0.4992773797353766141, 1524.841055067849993, 244.1317247718872068 ) ) ;
#89927=CARTESIAN_POINT ( 'NONE',  ( -3.317918599975760330, 1524.412928176729338, 241.9115272520634790 ) ) ;
#89932=CARTESIAN_POINT ( 'NONE',  ( -30.31052258194577931, 1523.604703353109699, 222.4930856806594193 ) ) ;
#89937=EDGE_LOOP ( 'NONE', ( #108369, #96730, #108874, #98990 ) ) ;
#89939=EDGE_CURVE ( 'NONE', #100597, #21777, #60957, .T. ) ;
#89940=CARTESIAN_POINT ( 'NONE',  ( -16.69366550187188381, 1526.382868172863937, 234.5416713104940811 ) ) ;
#89941=VERTEX_POINT ( 'NONE', #83293 ) ;
#89969=DIRECTION ( 'NONE',  ( -0.000000000000000000, -1.000000000000000000, -0.000000000000000000 ) ) ;
#89999=VERTEX_POINT ( 'NONE', #73953 ) ;
#90003=CARTESIAN_POINT ( 'NONE',  ( -3.347801439296141268, 1518.913060387330006, 176.1543725841967500 ) ) ;
#90020=DIRECTION ( 'NONE',  ( -1.000000000000000000, 0.000000000000000000, 0.000000000000000000 ) ) ;
#90022=DIRECTION ( 'NONE',  ( 0.9942586961433742543, 0.000000000000000000, -0.1070030146457445069 ) ) ;
#90044=FACE_BOUND ( 'NONE', #98471, .T. ) ;
#90054=CARTESIAN_POINT ( 'NONE',  ( 31.63976464710268388, 1525.343727714918259, 216.1854883492157740 ) ) ;
#90057=EDGE_CURVE ( 'NONE', #68807, #65505, #5617, .T. ) ;
#90059=ADVANCED_FACE ( 'NONE', ( #15115 ), #66669, .T. ) ;
#90061=CARTESIAN_POINT ( 'NONE',  ( 0.000000000000000000, 1522.051704408389924, 179.0139814193315999 ) ) ;
#90067=CARTESIAN_POINT ( 'NONE',  ( -18.07041998555320106, 1523.313115944345327, 180.1545818505813941 ) ) ;
#90077=AXIS2_PLACEMENT_3D ( 'NONE', #30017, #105654, #64207 ) ;
#90081=CARTESIAN_POINT ( 'NONE',  ( 19.67623451925527434, 1525.581535527370761, 237.1855307018971928 ) ) ;
#90101=CARTESIAN_POINT ( 'NONE',  ( 20.20959865099491992, 1522.382868172863937, 236.2316688286738611 ) ) ;
#90117=VERTEX_POINT ( 'NONE', #6179 ) ;
#90136=ORIENTED_EDGE ( 'NONE', *, *, #17077, .T. ) ;
#90138=CARTESIAN_POINT ( 'NONE',  ( 17.19739463999647100, 1525.960063244516959, 236.2603809477409982 ) ) ;
#90146=AXIS2_PLACEMENT_3D ( 'NONE', #89574, #104730, #28019 ) ;
#90148=CARTESIAN_POINT ( 'NONE',  ( 29.75840146891110649, 1525.320849883649316, 196.2322090936816323 ) ) ;
#90155=CIRCLE ( 'NONE', #40136, 1.000000000000000888 ) ;
#90169=CARTESIAN_POINT ( 'NONE',  ( 29.73374635647645547, 1526.349689584397083, 217.2224056390284659 ) ) ;
#90172=CARTESIAN_POINT ( 'NONE',  ( -32.72609422369149001, 1524.152349020271004, 201.1104022277331751 ) ) ;
#90177=DIRECTION ( 'NONE',  ( 0.000000000000000000, 0.000000000000000000, 1.000000000000000000 ) ) ;
#90187=CARTESIAN_POINT ( 'NONE',  ( 18.19590854888143738, 1522.382868172863937, 180.0410247165184501 ) ) ;
#90211=ORIENTED_EDGE ( 'NONE', *, *, #48105, .F. ) ;
#90218=ADVANCED_FACE ( 'NONE', ( #99671 ), #99121, .T. ) ;
#90224=CARTESIAN_POINT ( 'NONE',  ( 21.38516915557965703, 1522.382868172863937, 180.3939891059721106 ) ) ;
#90225=DIRECTION ( 'NONE',  ( 0.000000000000000000, 0.000000000000000000, -1.000000000000000000 ) ) ;
#90228=DIRECTION ( 'NONE',  ( 0.000000000000000000, 1.000000000000000000, 0.000000000000000000 ) ) ;
#90233=ORIENTED_EDGE ( 'NONE', *, *, #10703, .F. ) ;
#90234=AXIS2_PLACEMENT_3D ( 'NONE', #96504, #11945, #38237 ) ;
#90244=CARTESIAN_POINT ( 'NONE',  ( -22.75273496409559826, 1518.913060387330006, 234.5707981297189235 ) ) ;
#90260=ORIENTED_EDGE ( 'NONE', *, *, #11687, .F. ) ;
#90269=TOROIDAL_SURFACE ( 'NONE', #40240, 2.000000000000000000, 1.000000000000000000 ) ;
#90273=VERTEX_POINT ( 'NONE', #82889 ) ;
#90290=CARTESIAN_POINT ( 'NONE',  ( -22.66254714602097664, 1523.342713519622748, 181.4291743802705810 ) ) ;
#90306=ADVANCED_FACE ( 'NONE', ( #14016 ), #27045, .F. ) ;
#90337=DIRECTION ( 'NONE',  ( -0.5877852522924820189, 0.000000000000000000, -0.8090169943749410120 ) ) ;
#90340=CARTESIAN_POINT ( 'NONE',  ( 33.93019615848955084, 1512.187213306747481, 220.5829544587961095 ) ) ;
#90343=CARTESIAN_POINT ( 'NONE',  ( 32.36539586357643827, 1523.843263703803814, 216.1095015570140276 ) ) ;
#90349=ORIENTED_EDGE ( 'NONE', *, *, #101594, .F. ) ;
#90352=FACE_OUTER_BOUND ( 'NONE', #72351, .T. ) ;
#90358=DIRECTION ( 'NONE',  ( -0.4090087482554232712, -1.225281874271768203E-16, 0.9125304618754006558 ) ) ;
#90367=VERTEX_POINT ( 'NONE', #58799 ) ;
#90374=DIRECTION ( 'NONE',  ( -0.2054769195713296304, -0.000000000000000000, -0.9786619618251631847 ) ) ;
#90377=CARTESIAN_POINT ( 'NONE',  ( -30.61115703708014024, 1523.542365884048195, 196.4197133992117870 ) ) ;
#90385=CARTESIAN_POINT ( 'NONE',  ( -17.04790460295724230, 1526.208281990537671, 182.6359253440253667 ) ) ;
#90386=CARTESIAN_POINT ( 'NONE',  ( 21.55489959617532136, 1524.059547553519451, 234.2080540443132861 ) ) ;
#90396=EDGE_LOOP ( 'NONE', ( #38380, #25179, #106867, #78106 ) ) ;
#90401=AXIS2_PLACEMENT_3D ( 'NONE', #13108, #3110, #54071 ) ;
#90410=CARTESIAN_POINT ( 'NONE',  ( 2.404972330437235684, 1525.211473355384896, 176.1486567441184832 ) ) ;
#90423=CIRCLE ( 'NONE', #24240, 33.13701971169416538 ) ;
#90425=EDGE_CURVE ( 'NONE', #82045, #94134, #682, .T. ) ;
#90434=CARTESIAN_POINT ( 'NONE',  ( 30.31644210120071747, 1523.530870145310473, 195.7504609407426983 ) ) ;
#90437=ADVANCED_FACE ( 'NONE', ( #72191 ), #81416, .F. ) ;
#90444=CARTESIAN_POINT ( 'NONE',  ( 21.84020450211271225, 1523.481610118012213, 183.2638850456620219 ) ) ;
#90451=DIRECTION ( 'NONE',  ( 1.776356839400250465E-15, 0.000000000000000000, 1.000000000000000000 ) ) ;
#90476=CARTESIAN_POINT ( 'NONE',  ( -32.38845791999504797, 1523.382868172864164, 202.1182848005516348 ) ) ;
#90486=CARTESIAN_POINT ( 'NONE',  ( 29.86461515634920971, 1525.960063244517187, 220.9690070206020494 ) ) ;
#90507=EDGE_CURVE ( 'NONE', #39464, #20284, #48613, .T. ) ;
#90526=FACE_OUTER_BOUND ( 'NONE', #80946, .T. ) ;
#90527=EDGE_LOOP ( 'NONE', ( #95797, #74334, #94803 ) ) ;
#90543=FACE_OUTER_BOUND ( 'NONE', #1506, .T. ) ;
#90550=CARTESIAN_POINT ( 'NONE',  ( -29.55269881708357715, 1525.821544997590763, 221.1141083160998448 ) ) ;
#90565=ORIENTED_EDGE ( 'NONE', *, *, #25315, .F. ) ;
#90586=DIRECTION ( 'NONE',  ( -0.000000000000000000, -1.000000000000000000, -0.000000000000000000 ) ) ;
#90587=( BOUNDED_CURVE ( )  B_SPLINE_CURVE ( 3, ( #103088, #103661, #26959, #11272 ),
 .UNSPECIFIED., .F., .F. ) 
 B_SPLINE_CURVE_WITH_KNOTS ( ( 4, 4 ),
 ( 4.712388980384689674, 6.283185307179586232 ),
 .UNSPECIFIED. ) 
 CURVE ( )  GEOMETRIC_REPRESENTATION_ITEM ( )  RATIONAL_B_SPLINE_CURVE ( ( 1.000000000000000000, 0.8047378541243649375, 0.8047378541243649375, 1.000000000000000000 ) ) 
 REPRESENTATION_ITEM ( '' )  );
#90593=CARTESIAN_POINT ( 'NONE',  ( -21.84020450211325937, 1523.481610118012441, 183.2638850456619366 ) ) ;
#90605=EDGE_CURVE ( 'NONE', #8681, #39550, #36497, .T. ) ;
#90607=FACE_OUTER_BOUND ( 'NONE', #275, .T. ) ;
#90613=CARTESIAN_POINT ( 'NONE',  ( -17.17241001986462123, 1512.187213306747481, 238.6251415217917895 ) ) ;
#90621=ORIENTED_EDGE ( 'NONE', *, *, #83639, .T. ) ;
#90628=CARTESIAN_POINT ( 'NONE',  ( 3.350338079455597917, 1523.604703353109699, 242.0808062845893289 ) ) ;
#90631=DIRECTION ( 'NONE',  ( -0.6709778558543766369, 0.000000000000000000, -0.7414773880254632576 ) ) ;
#90632=FACE_OUTER_BOUND ( 'NONE', #4142, .T. ) ;
#90638=CARTESIAN_POINT ( 'NONE',  ( 31.23437356469446868, 1518.913060387330006, 221.8968241038843701 ) ) ;
#90648=CARTESIAN_POINT ( 'NONE',  ( 2.857353854284549577, 1525.661275128775742, 177.1476418759443163 ) ) ;
#90655=LINE ( 'NONE', #78004, #46311 ) ;
#90662=CYLINDRICAL_SURFACE ( 'NONE', #50425, 0.9999999999999976685 ) ;
#90668=ORIENTED_EDGE ( 'NONE', *, *, #11999, .T. ) ;
#90682=CARTESIAN_POINT ( 'NONE',  ( 16.73628186595829703, 1526.382868172864164, 234.1845039693042452 ) ) ;
#90688=VERTEX_POINT ( 'NONE', #39532 ) ;
#90695=CARTESIAN_POINT ( 'NONE',  ( -30.90487439922522483, 1525.907212628473872, 216.4335774778785151 ) ) ;
#90698=EDGE_CURVE ( 'NONE', #82691, #49611, #101914, .T. ) ;
#90706=TOROIDAL_SURFACE ( 'NONE', #42432, 32.13701971169416538, 1.000000000000000000 ) ;
#90715=AXIS2_PLACEMENT_3D ( 'NONE', #59521, #86356, #178 ) ;
#90730=CARTESIAN_POINT ( 'NONE',  ( 31.81407709660769001, 1512.187213306747481, 196.2902540610627682 ) ) ;
#90732=CARTESIAN_POINT ( 'NONE',  ( -19.90023153800419564, 1526.278758871496166, 235.2784539741628578 ) ) ;
#90735=AXIS2_PLACEMENT_3D ( 'NONE', #50946, #34129, #554 ) ;
#90739=CYLINDRICAL_SURFACE ( 'NONE', #62161, 2.000000000000001776 ) ;
#90741=CARTESIAN_POINT ( 'NONE',  ( 21.83550407203906119, 1523.678648413191468, 183.2743720722706655 ) ) ;
#90764=CARTESIAN_POINT ( 'NONE',  ( 31.41104781486823327, 1511.187213306747708, 215.9140555522422460 ) ) ;
#90767=CARTESIAN_POINT ( 'NONE',  ( -16.87900699709518193, 1524.382868172804365, 237.0109764097493326 ) ) ;
#90784=FACE_OUTER_BOUND ( 'NONE', #102508, .T. ) ;
#90789=VECTOR ( 'NONE', #13879, 1000.000000000000000 ) ;
#90799=VERTEX_POINT ( 'NONE', #26006 ) ;
#90813=DIRECTION ( 'NONE',  ( -0.000000000000000000, -1.000000000000000000, -0.000000000000000000 ) ) ;
#90822=VECTOR ( 'NONE', #33469, 1000.000000000000114 ) ;
#90825=CARTESIAN_POINT ( 'NONE',  ( -3.347801439371857146, 1523.456924617337108, 242.0893193391915474 ) ) ;
#90829=FACE_OUTER_BOUND ( 'NONE', #81506, .T. ) ;
#90846=CARTESIAN_POINT ( 'NONE',  ( -22.41686883764639759, 1524.667648926078755, 181.9773018742353372 ) ) ;
#90853=B_SPLINE_CURVE_WITH_KNOTS ( 'NONE', 3,
 ( #41782, #42335, #92731, #7080, #17093, #16006, #33924, #110639, #76487, #75937 ),
 .UNSPECIFIED., .F., .F.,
 ( 4, 2, 2, 2, 4 ),
 ( 0.000000000000000000, 0.0007403986298595332041, 0.001480797259719066408, 0.002221195889578599612, 0.002961594519438132816 ),
 .UNSPECIFIED. ) ;
#90866=DIRECTION ( 'NONE',  ( 0.000000000000000000, 1.000000000000000000, 0.000000000000000000 ) ) ;
#90873=DIRECTION ( 'NONE',  ( -0.5877852522924785772, 0.000000000000000000, 0.8090169943749434545 ) ) ;
#90879=CIRCLE ( 'NONE', #31883, 1.000000000000000888 ) ;
#90895=CARTESIAN_POINT ( 'NONE',  ( 22.75273496409597485, 1512.187213306747481, 234.5707981297185825 ) ) ;
#90899=CIRCLE ( 'NONE', #28325, 30.13701971169416183 ) ;
#90900=DIRECTION ( 'NONE',  ( 0.000000000000000000, 0.000000000000000000, -1.000000000000000000 ) ) ;
#90906=CARTESIAN_POINT ( 'NONE',  ( -20.70484064406418412, 1525.907212628473644, 185.0411015109856692 ) ) ;
#90912=ORIENTED_EDGE ( 'NONE', *, *, #19692, .T. ) ;
#90918=CARTESIAN_POINT ( 'NONE',  ( 16.85976061912576185, 1525.821544997590308, 236.1944305375346858 ) ) ;
#90919=DIRECTION ( 'NONE',  ( 0.000000000000000000, 1.000000000000000000, 0.000000000000000000 ) ) ;
#90940=CARTESIAN_POINT ( 'NONE',  ( -30.31644210120141381, 1523.530870145310473, 195.7504609407442615 ) ) ;
#90949=CARTESIAN_POINT ( 'NONE',  ( 22.08622291482331690, 1523.456872492435195, 184.4183880513174927 ) ) ;
#90958=EDGE_LOOP ( 'NONE', ( #29503, #18862, #48141, #57472 ) ) ;
#90969=CARTESIAN_POINT ( 'NONE',  ( -30.47387511496757639, 1525.394057003703438, 196.7420889653906215 ) ) ;
#90970=ORIENTED_EDGE ( 'NONE', *, *, #43865, .T. ) ;
#91018=VERTEX_POINT ( 'NONE', #18170 ) ;
#91022=EDGE_CURVE ( 'NONE', #89999, #13894, #43253, .T. ) ;
#91047=CARTESIAN_POINT ( 'NONE',  ( 3.448830483803564828, 1511.187213306747708, 175.1594891075192209 ) ) ;
#91049=CIRCLE ( 'NONE', #21330, 1.000000000000000888 ) ;
#91061=ADVANCED_FACE ( 'NONE', ( #30295 ), #43104, .T. ) ;
#91067=ADVANCED_FACE ( 'NONE', ( #31952 ), #50061, .F. ) ;
#91094=AXIS2_PLACEMENT_3D ( 'NONE', #21190, #55400, #89531 ) ;
#91101=AXIS2_PLACEMENT_3D ( 'NONE', #101355, #51543, #52106 ) ;
#91107=CARTESIAN_POINT ( 'NONE',  ( 21.12212911287011607, 1511.187213306747708, 182.4210318429774134 ) ) ;
#91110=FACE_OUTER_BOUND ( 'NONE', #18516, .T. ) ;
#91111=AXIS2_PLACEMENT_3D ( 'NONE', #30554, #56318, #90451 ) ;
#91123=ORIENTED_EDGE ( 'NONE', *, *, #7129, .F. ) ;
#91137=EDGE_LOOP ( 'NONE', ( #62772, #71334, #25365, #95250 ) ) ;
#91164=CARTESIAN_POINT ( 'NONE',  ( -16.64885258016277803, 1526.344110814222404, 234.9109520333565797 ) ) ;
#91172=ORIENTED_EDGE ( 'NONE', *, *, #8363, .T. ) ;
#91173=AXIS2_PLACEMENT_3D ( 'NONE', #40403, #83500, #109283 ) ;
#91192=CIRCLE ( 'NONE', #19655, 1.000000000000000888 ) ;
#91212=CARTESIAN_POINT ( 'NONE',  ( 29.37542415142989327, 1526.382868172864164, 200.9849896654459087 ) ) ;
#91222=CARTESIAN_POINT ( 'NONE',  ( -20.70484064406422320, 1525.907212628473644, 185.0411015109855839 ) ) ;
#91230=CARTESIAN_POINT ( 'NONE',  ( 17.29882006758069934, 1523.542365884050241, 237.3908737315652786 ) ) ;
#91235=EDGE_CURVE ( 'NONE', #33528, #79144, #33909, .T. ) ;
#91245=DIRECTION ( 'NONE',  ( -0.5369043659965772042, -0.4884709562386981840, 0.6878443331779838799 ) ) ;
#91249=EDGE_LOOP ( 'NONE', ( #74705, #107401, #107439, #55290 ) ) ;
#91267=CARTESIAN_POINT ( 'NONE',  ( 30.01482722728456665, 1525.231909165051093, 196.6362179804465882 ) ) ;
#91290=EDGE_CURVE ( 'NONE', #61519, #72801, #56896, .T. ) ;
#91291=CARTESIAN_POINT ( 'NONE',  ( -32.10255801038886858, 1525.211477436245787, 201.2198389390407272 ) ) ;
#91296=DIRECTION ( 'NONE',  ( -0.03173147633638266629, -0.9969860201949399814, -0.07079540200725242816 ) ) ;
#91312=CARTESIAN_POINT ( 'NONE',  ( -17.05900707844612185, 1524.678872986499300, 181.0478682887629702 ) ) ;
#91335=LINE ( 'NONE', #81818, #46456 ) ;
#91356=CIRCLE ( 'NONE', #52045, 30.13701971169416183 ) ;
#91366=FACE_OUTER_BOUND ( 'NONE', #106541, .T. ) ;
#91374=CARTESIAN_POINT ( 'NONE',  ( -31.92108011125334599, 1512.187213306747481, 220.9591791661900686 ) ) ;
#91375=VECTOR ( 'NONE', #75876, 1000.000000000000000 ) ;
#91380=VERTEX_POINT ( 'NONE', #85948 ) ;
#91383=CARTESIAN_POINT ( 'NONE',  ( 18.19590854888164699, 1522.862737210649584, 238.2026672068774360 ) ) ;
#91388=EDGE_CURVE ( 'NONE', #74525, #95777, #100328, .T. ) ;
#91402=VECTOR ( 'NONE', #96395, 1000.000000000000000 ) ;
#91406=CARTESIAN_POINT ( 'NONE',  ( 0.000000000000000000, 1511.187213306747708, 209.1218459616979999 ) ) ;
#91408=DIRECTION ( 'NONE',  ( -0.2054769195713296304, 0.000000000000000000, -0.9786619618251631847 ) ) ;
#91417=DIRECTION ( 'NONE',  ( -1.040834085586083310E-14, 0.000000000000000000, 1.000000000000000000 ) ) ;
#91428=ORIENTED_EDGE ( 'NONE', *, *, #14328, .F. ) ;
#91429=CARTESIAN_POINT ( 'NONE',  ( -2.038646110889565932, 1525.960063244516959, 177.0579350083065435 ) ) ;
#91435=CARTESIAN_POINT ( 'NONE',  ( 16.83198307402578564, 1526.000688113713295, 182.3274564795797801 ) ) ;
#91460=CARTESIAN_POINT ( 'NONE',  ( 20.20959865099471031, 1511.187213306747708, 182.0120230947219966 ) ) ;
#91466=CARTESIAN_POINT ( 'NONE',  ( 32.05702909905449616, 1524.477587234266366, 216.6895769861147301 ) ) ;
#91469=CIRCLE ( 'NONE', #66482, 1.000000000000000888 ) ;
#91473=ORIENTED_EDGE ( 'NONE', *, *, #45377, .T. ) ;
#91479=CARTESIAN_POINT ( 'NONE',  ( 16.54281257266469751, 1524.843416604499225, 237.3982989049651167 ) ) ;
#91519=DIRECTION ( 'NONE',  ( -0.2054769195713179730, -0.000000000000000000, -0.9786619618251657382 ) ) ;
#91547=CARTESIAN_POINT ( 'NONE',  ( -22.08327125186908191, 1523.604703353109699, 233.8169256665491105 ) ) ;
#91565=VERTEX_POINT ( 'NONE', #47257 ) ;
#91587=CARTESIAN_POINT ( 'NONE',  ( -17.43549125882602979, 1525.211477436245787, 237.2113384875502788 ) ) ;
#91593=LINE ( 'NONE', #22701, #103327 ) ;
#91596=CARTESIAN_POINT ( 'NONE',  ( 21.38516915557965703, 1512.187213306747481, 180.3939891059721106 ) ) ;
#91603=CARTESIAN_POINT ( 'NONE',  ( -20.07149347155893437, 1526.186458717540972, 233.0642689910355898 ) ) ;
#91619=EDGE_CURVE ( 'NONE', #96103, #70084, #107515, .T. ) ;
#91636=EDGE_LOOP ( 'NONE', ( #18638, #29687, #19558, #27246, #100720 ) ) ;
#91648=B_SPLINE_CURVE_WITH_KNOTS ( 'NONE', 3,
 ( #106129, #20442, #98269, #90969, #3697, #56836, #13140, #38359, #31063, #39477 ),
 .UNSPECIFIED., .F., .F.,
 ( 4, 2, 2, 2, 4 ),
 ( 3.469446951953614189E-17, 0.0007406479101619073066, 0.001481295820323779919, 0.002221943730485652531, 0.002962591640647525143 ),
 .UNSPECIFIED. ) ;
#91654=CARTESIAN_POINT ( 'NONE',  ( 30.47385413848734004, 1525.394081235439444, 196.7421045368866146 ) ) ;
#91656=ORIENTED_EDGE ( 'NONE', *, *, #39222, .F. ) ;
#91674=CARTESIAN_POINT ( 'NONE',  ( -3.232732302729357521, 1524.860077346004800, 241.7126682117879284 ) ) ;
#91695=DIRECTION ( 'NONE',  ( 0.000000000000000000, 0.000000000000000000, -1.000000000000000000 ) ) ;
#91700=DIRECTION ( 'NONE',  ( -0.000000000000000000, -1.000000000000000000, -0.000000000000000000 ) ) ;
#91702=EDGE_CURVE ( 'NONE', #100110, #105489, #55675, .T. ) ;
#91714=CARTESIAN_POINT ( 'NONE',  ( -31.33756686635731015, 1523.580204110584191, 221.9021554030055938 ) ) ;
#91720=DIRECTION ( 'NONE',  ( 5.204170427930416866E-14, 0.000000000000000000, 1.000000000000000000 ) ) ;
#91721=VERTEX_POINT ( 'NONE', #109376 ) ;
#91722=CARTESIAN_POINT ( 'NONE',  ( 31.50799703744283420, 1526.382868172863937, 216.4233194664827238 ) ) ;
#91725=ORIENTED_EDGE ( 'NONE', *, *, #89051, .T. ) ;
#91731=CARTESIAN_POINT ( 'NONE',  ( -16.50400130224786466, 1525.907212628473644, 181.9890130758379030 ) ) ;
#91738=DIRECTION ( 'NONE',  ( -0.000000000000000000, -1.000000000000000000, -0.000000000000000000 ) ) ;
#91748=EDGE_CURVE ( 'NONE', #72812, #64568, #26973, .T. ) ;
#91758=CARTESIAN_POINT ( 'NONE',  ( 29.74444329484277105, 1526.348417187222140, 201.0223654199409111 ) ) ;
#91761=ORIENTED_EDGE ( 'NONE', *, *, #31050, .T. ) ;
#91781=VERTEX_POINT ( 'NONE', #107708 ) ;
#91808=FACE_OUTER_BOUND ( 'NONE', #5908, .T. ) ;
#91834=EDGE_CURVE ( 'NONE', #67570, #94817, #62975, .T. ) ;
#91843=CARTESIAN_POINT ( 'NONE',  ( -2.314969334973925541, 1525.402221411349728, 174.6257708845644174 ) ) ;
#91858=EDGE_CURVE ( 'NONE', #96482, #65697, #67384, .T. ) ;
#91862=B_SPLINE_CURVE_WITH_KNOTS ( 'NONE', 3,
 ( #54707, #18845, #63124, #70968, #21049, #53041 ),
 .UNSPECIFIED., .F., .F.,
 ( 4, 2, 4 ),
 ( -1.131363979615749172E-05, 0.001067788114096062963, 0.002146889867988283161 ),
 .UNSPECIFIED. ) ;
#91881=DIRECTION ( 'NONE',  ( -0.9786619618251627406, 0.000000000000000000, 0.2054769195713317953 ) ) ;
#91899=ORIENTED_EDGE ( 'NONE', *, *, #3750, .F. ) ;
#91915=FACE_OUTER_BOUND ( 'NONE', #106407, .T. ) ;
#91918=ORIENTED_EDGE ( 'NONE', *, *, #102104, .F. ) ;
#91925=DIRECTION ( 'NONE',  ( 0.000000000000000000, -1.000000000000000000, 0.000000000000000000 ) ) ;
#91927=AXIS2_PLACEMENT_3D ( 'NONE', #84191, #93677, #109959 ) ;
#91941=ORIENTED_EDGE ( 'NONE', *, *, #107044, .T. ) ;
#91945=CARTESIAN_POINT ( 'NONE',  ( -18.02257621027615642, 1526.382868172863937, 182.8951942368373977 ) ) ;
#91947=ADVANCED_FACE ( 'NONE', ( #71259 ), #22863, .F. ) ;
#91949=CARTESIAN_POINT ( 'NONE',  ( -31.81407709660786409, 1512.187213306747481, 196.2902540610632229 ) ) ;
#91956=VERTEX_POINT ( 'NONE', #90764 ) ;
#91968=EDGE_CURVE ( 'NONE', #49270, #65505, #34346, .T. ) ;
#92004=EDGE_CURVE ( 'NONE', #75732, #81986, #62902, .T. ) ;
#92012=CARTESIAN_POINT ( 'NONE',  ( 32.85805783624310550, 1523.678648413191922, 217.1983043299902647 ) ) ;
#92015=FACE_OUTER_BOUND ( 'NONE', #18493, .T. ) ;
#92019=VERTEX_POINT ( 'NONE', #35274 ) ;
#92038=ORIENTED_EDGE ( 'NONE', *, *, #8949, .T. ) ;
#92049=VECTOR ( 'NONE', #104175, 999.9999999999998863 ) ;
#92069=DIRECTION ( 'NONE',  ( 0.000000000000000000, 1.000000000000000000, 0.000000000000000000 ) ) ;
#92073=ORIENTED_EDGE ( 'NONE', *, *, #63186, .F. ) ;
#92079=ORIENTED_EDGE ( 'NONE', *, *, #30850, .F. ) ;
#92090=CARTESIAN_POINT ( 'NONE',  ( 21.59395510246053007, 1525.159177407156676, 184.7447231557273142 ) ) ;
#92098=EDGE_CURVE ( 'NONE', #23328, #63792, #33058, .T. ) ;
#92101=EDGE_CURVE ( 'NONE', #18078, #75732, #95054, .T. ) ;
#92115=EDGE_CURVE ( 'NONE', #53391, #2813, #14549, .T. ) ;
#92139=ADVANCED_FACE ( 'NONE', ( #17895 ), #80754, .T. ) ;
#92169=FACE_OUTER_BOUND ( 'NONE', #6192, .T. ) ;
#92173=AXIS2_PLACEMENT_3D ( 'NONE', #45220, #46330, #4833 ) ;
#92202=VECTOR ( 'NONE', #51864, 1000.000000000000227 ) ;
#92204=CARTESIAN_POINT ( 'NONE',  ( -17.84338787571960694, 1523.382868172864164, 180.3600277896300383 ) ) ;
#92206=ORIENTED_EDGE ( 'NONE', *, *, #84884, .F. ) ;
#92208=CARTESIAN_POINT ( 'NONE',  ( -31.23437356469455040, 1512.187213306747481, 195.3468678195118287 ) ) ;
#92209=DIRECTION ( 'NONE',  ( -0.000000000000000000, -1.000000000000000000, -0.000000000000000000 ) ) ;
#92224=VERTEX_POINT ( 'NONE', #101341 ) ;
#92242=EDGE_CURVE ( 'NONE', #39868, #2574, #87959, .T. ) ;
#92245=CARTESIAN_POINT ( 'NONE',  ( 2.458491834123362807, 1524.872178180562969, 175.9022251074391932 ) ) ;
#92252=FACE_OUTER_BOUND ( 'NONE', #46582, .T. ) ;
#92264=CARTESIAN_POINT ( 'NONE',  ( -30.61443310214863445, 1523.462669333488066, 221.8243310972612221 ) ) ;
#92270=CARTESIAN_POINT ( 'NONE',  ( 32.86802468386292730, 1512.187213306747481, 217.2040256693915410 ) ) ;
#92274=CARTESIAN_POINT ( 'NONE',  ( 33.28034951413929576, 1522.382868172863937, 217.4407153818819722 ) ) ;
#92285=CARTESIAN_POINT ( 'NONE',  ( 1.338895077072802531, 1526.382868172864164, 178.6697305272271024 ) ) ;
#92292=CARTESIAN_POINT ( 'NONE',  ( 32.86470158750944393, 1523.580203803270933, 217.2021180890986614 ) ) ;
#92294=CARTESIAN_POINT ( 'NONE',  ( -22.08327125186962192, 1523.604703353109699, 184.4267662568474009 ) ) ;
#92295=FACE_OUTER_BOUND ( 'NONE', #1485, .T. ) ;
#92322=CARTESIAN_POINT ( 'NONE',  ( 17.17241001986483795, 1512.187213306747481, 179.6185504016043240 ) ) ;
#92330=DIRECTION ( 'NONE',  ( 0.000000000000000000, 1.000000000000000000, 0.000000000000000000 ) ) ;
#92334=AXIS2_PLACEMENT_3D ( 'NONE', #85572, #91925, #15198 ) ;
#92344=ORIENTED_EDGE ( 'NONE', *, *, #19121, .F. ) ;
#92362=CARTESIAN_POINT ( 'NONE',  ( 32.36513277069983019, 1523.847248782568613, 202.1343718111426426 ) ) ;
#92384=CARTESIAN_POINT ( 'NONE',  ( -0.4681535437661719090, 1524.397344074316607, 173.8154889443011371 ) ) ;
#92397=CARTESIAN_POINT ( 'NONE',  ( -16.62424264452936029, 1524.075132568165600, 180.5391555246563087 ) ) ;
#92398=CARTESIAN_POINT ( 'NONE',  ( 22.75273496409597485, 1511.187213306747708, 234.5707981297185825 ) ) ;
#92420=DIRECTION ( 'NONE',  ( 0.000000000000000000, 0.000000000000000000, 1.000000000000000000 ) ) ;
#92435=ORIENTED_EDGE ( 'NONE', *, *, #71827, .T. ) ;
#92449=ADVANCED_FACE ( 'NONE', ( #13353 ), #47546, .T. ) ;
#92482=CARTESIAN_POINT ( 'NONE',  ( 21.83117874278439174, 1524.760046179776054, 233.6180677221980488 ) ) ;
#92488=ADVANCED_FACE ( 'NONE', ( #9805 ), #93285, .T. ) ;
#92498=EDGE_CURVE ( 'NONE', #97770, #95189, #15042, .T. ) ;
#92500=CARTESIAN_POINT ( 'NONE',  ( 0.000000000000000000, 1518.913060387330006, 209.1218459616979999 ) ) ;
#92519=EDGE_LOOP ( 'NONE', ( #2608, #5743, #98714, #79713 ) ) ;
#92539=CARTESIAN_POINT ( 'NONE',  ( 30.51231035492521571, 1526.382868172863937, 218.1578534183718432 ) ) ;
#92555=CARTESIAN_POINT ( 'NONE',  ( -33.28034951413921760, 1522.382868172863937, 217.4407153818824838 ) ) ;
#92556=ORIENTED_EDGE ( 'NONE', *, *, #28546, .F. ) ;
#92577=ORIENTED_EDGE ( 'NONE', *, *, #82353, .T. ) ;
#92603=CIRCLE ( 'NONE', #46198, 33.13701971169416538 ) ;
#92622=CARTESIAN_POINT ( 'NONE',  ( -32.97913964219445404, 1512.187213306747481, 197.9697544589750464 ) ) ;
#92624=AXIS2_PLACEMENT_3D ( 'NONE', #22267, #89506, #65433 ) ;
#92636=CARTESIAN_POINT ( 'NONE',  ( -31.81407709660760830, 1512.187213306747481, 221.9534378623334590 ) ) ;
#92639=CARTESIAN_POINT ( 'NONE',  ( 17.27380198137656109, 1525.712835404586031, 181.5601764590613243 ) ) ;
#92642=VERTEX_POINT ( 'NONE', #28263 ) ;
#92652=CARTESIAN_POINT ( 'NONE',  ( -20.71343476517491311, 1501.977400791986611, 238.3377464195766890 ) ) ;
#92657=DIRECTION ( 'NONE',  ( 0.000000000000000000, 0.000000000000000000, 1.000000000000000000 ) ) ;
#92659=CARTESIAN_POINT ( 'NONE',  ( -34.68852446352934749, 1522.382868172863709, 218.2490599186012048 ) ) ;
#92660=DIRECTION ( 'NONE',  ( 0.000000000000000000, 0.000000000000000000, -1.000000000000000000 ) ) ;
#92663=B_SPLINE_CURVE_WITH_KNOTS ( 'NONE', 3,
 ( #38939, #105627, #13728, #5355 ),
 .UNSPECIFIED., .F., .F.,
 ( 4, 4 ),
 ( 0.000000000000000000, 0.0002960034161023848394 ),
 .UNSPECIFIED. ) ;
#92670=CARTESIAN_POINT ( 'NONE',  ( -20.85167060786264770, 1525.730671948511599, 184.1901411363043906 ) ) ;
#92676=AXIS2_PLACEMENT_3D ( 'NONE', #52401, #45109, #70876 ) ;
#92708=CIRCLE ( 'NONE', #24748, 1.999999999999996669 ) ;
#92713=VERTEX_POINT ( 'NONE', #22029 ) ;
#92721=EDGE_CURVE ( 'NONE', #21131, #84410, #105779, .T. ) ;
#92724=CARTESIAN_POINT ( 'NONE',  ( -18.02257621027557377, 1524.382868172863937, 235.3484976865589147 ) ) ;
#92731=CARTESIAN_POINT ( 'NONE',  ( 2.493583506516910298, 1524.152349020271004, 242.7218833893027750 ) ) ;
#92735=DIRECTION ( 'NONE',  ( 0.000000000000000000, -0.000000000000000000, 1.000000000000000000 ) ) ;
#92736=CARTESIAN_POINT ( 'NONE',  ( 21.83550407203906119, 1523.678648413191468, 183.2743720722706655 ) ) ;
#92739=CARTESIAN_POINT ( 'NONE',  ( 31.92108011125342770, 1512.187213306747481, 197.2845127572061301 ) ) ;
#92744=DIRECTION ( 'NONE',  ( 0.4090087482554252696, 0.000000000000000000, -0.9125304618753996566 ) ) ;
#92746=CARTESIAN_POINT ( 'NONE',  ( 0.4151546846821903003, 1512.187213306747481, 242.9330574173806951 ) ) ;
#92750=DIRECTION ( 'NONE',  ( 1.734723475976805517E-15, 0.000000000000000000, 1.000000000000000000 ) ) ;
#92754=CARTESIAN_POINT ( 'NONE',  ( -28.27139721233027458, 1526.382868172864164, 219.5606225550389468 ) ) ;
#92764=DIRECTION ( 'NONE',  ( -0.4090087482554252696, 0.000000000000000000, 0.9125304618753996566 ) ) ;
#92770=DIRECTION ( 'NONE',  ( -0.5877852522924762457, 0.000000000000000000, 0.8090169943749451198 ) ) ;
#92786=VERTEX_POINT ( 'NONE', #88733 ) ;
#92789=CARTESIAN_POINT ( 'NONE',  ( -32.85805783624314813, 1523.678648413191695, 201.0453875934059340 ) ) ;
#92816=CARTESIAN_POINT ( 'NONE',  ( 18.19590854887482578, 1522.644714754858796, 180.0410247165244471 ) ) ;
#92822=ORIENTED_EDGE ( 'NONE', *, *, #14485, .T. ) ;
#92823=CARTESIAN_POINT ( 'NONE',  ( 34.61172972909617584, 1523.342713519622976, 218.2049768989050449 ) ) ;
#92826=ORIENTED_EDGE ( 'NONE', *, *, #15213, .T. ) ;
#92842=AXIS2_PLACEMENT_3D ( 'NONE', #858, #11861, #85373 ) ;
#92848=AXIS2_PLACEMENT_3D ( 'NONE', #25896, #194, #102595 ) ;
#92849=DIRECTION ( 'NONE',  ( 0.9149707217702669482, 0.000000000000000000, 0.4035202328300239172 ) ) ;
#92862=CARTESIAN_POINT ( 'NONE',  ( -32.85805783624314813, 1523.678648413191695, 201.0453875934059340 ) ) ;
#92871=( BOUNDED_SURFACE ( )  B_SPLINE_SURFACE ( 3, 2, ( 
 ( #84930, #8777, #51344 ),
 ( #25019, #102289, #93338 ),
 ( #970, #17153, #58659 ),
 ( #84399, #110699, #25571 ),
 ( #59221, #85478, #58112 ),
 ( #7686, #68726, #92245 ),
 ( #15515, #7143, #42958 ),
 ( #77119, #94432, #17711 ),
 ( #76545, #50269, #16603 ),
 ( #50801, #41844, #33991 ),
 ( #109606, #425, #33421 ),
 ( #67070, #83844, #8224 ),
 ( #41299, #34542, #102830 ),
 ( #26125, #86054, #32880 ) ),
 .UNSPECIFIED., .F., .F., .F. ) 
 B_SPLINE_SURFACE_WITH_KNOTS ( ( 4, 2, 2, 2, 2, 2, 4 ),
 ( 3, 3 ),
 ( 0.000000000000000000, 0.0009440840677143950543, 0.001416126101571592473, 0.001888168135428790109, 0.002360210169285987744, 0.002832252203143184946, 0.003776336270857580217 ),
 ( 0.000000000000000000, 1.000000000000000000 ),
 .UNSPECIFIED. ) 
 GEOMETRIC_REPRESENTATION_ITEM ( )  RATIONAL_B_SPLINE_SURFACE ( (
 ( 1.000000000000000000, 0.8070209408750023128, 1.000000000000000000),
 ( 1.000000000000000000, 0.8215603905285601138, 1.000000000000000000),
 ( 1.000000000000000000, 0.8340988699059065370, 1.000000000000000000),
 ( 1.000000000000000000, 0.8516751610459424304, 1.000000000000000000),
 ( 1.000000000000000000, 0.8573697395158380585, 1.000000000000000000),
 ( 1.000000000000000000, 0.8683586635658061548, 1.000000000000000000),
 ( 1.000000000000000000, 0.8736518481709314443, 1.000000000000000000),
 ( 1.000000000000000000, 0.8840377753029409202, 1.000000000000000000),
 ( 1.000000000000000000, 0.8891294171307203564, 1.000000000000000000),
 ( 1.000000000000000000, 0.8992456600573149883, 1.000000000000000000),
 ( 1.000000000000000000, 0.9042785869252324416, 1.000000000000000000),
 ( 1.000000000000000000, 0.9189749222839583842, 1.000000000000000000),
 ( 1.000000000000000000, 0.9283978182347611963, 1.000000000000000000),
 ( 1.000000000000000000, 0.9376006582765945563, 1.000000000000000000) ) ) 
 REPRESENTATION_ITEM ( '' )  SURFACE ( )  );
#92879=CARTESIAN_POINT ( 'NONE',  ( -32.02808312589908013, 1512.187213306747481, 219.9649204700466782 ) ) ;
#92883=ORIENTED_EDGE ( 'NONE', *, *, #56640, .F. ) ;
#92887=AXIS2_PLACEMENT_3D ( 'NONE', #4902, #15488, #82159 ) ;
#92902=ORIENTED_EDGE ( 'NONE', *, *, #5642, .T. ) ;
#92915=CARTESIAN_POINT ( 'NONE',  ( -16.62350534370865418, 1524.082740465118604, 180.5404690658195932 ) ) ;
#92920=CARTESIAN_POINT ( 'NONE',  ( -32.85805783624317655, 1523.678648413191695, 201.0453875934059056 ) ) ;
#92943=PLANE ( 'NONE',  #3827 ) ;
#92959=CARTESIAN_POINT ( 'NONE',  ( 2.470168521978401088, 1523.382868172864164, 175.3649660270905315 ) ) ;
#92973=CARTESIAN_POINT ( 'NONE',  ( -31.43069643840509642, 1526.748660780343471, 201.6857111062228967 ) ) ;
#93009=DIRECTION ( 'NONE',  ( -0.1070030146457386366, 0.000000000000000000, -0.9942586961433749204 ) ) ;
#93013=CIRCLE ( 'NONE', #101956, 2.000000000000001776 ) ;
#93015=ORIENTED_EDGE ( 'NONE', *, *, #46890, .F. ) ;
#93022=CYLINDRICAL_SURFACE ( 'NONE', #4920, 1.000000000000000888 ) ;
#93039=CARTESIAN_POINT ( 'NONE',  ( 20.70484064406403846, 1525.907212628473644, 233.2025904124105580 ) ) ;
#93041=LINE ( 'NONE', #48317, #29680 ) ;
#93054=CARTESIAN_POINT ( 'NONE',  ( 17.17241001986506888, 1512.187213306747481, 238.6251415217915337 ) ) ;
#93055=CARTESIAN_POINT ( 'NONE',  ( -21.64969004980934741, 1524.547873515822630, 234.6921391611746230 ) ) ;
#93068=FACE_OUTER_BOUND ( 'NONE', #31246, .T. ) ;
#93076=CARTESIAN_POINT ( 'NONE',  ( -32.38114538885245253, 1523.604703353109699, 216.1203639561433363 ) ) ;
#93078=ADVANCED_FACE ( 'NONE', ( #39967 ), #62172, .F. ) ;
#93094=CARTESIAN_POINT ( 'NONE',  ( 32.66476241579317730, 1526.382868172863937, 219.1158660759119243 ) ) ;
#93096=CARTESIAN_POINT ( 'NONE',  ( -30.38265071699166953, 1524.478200376968516, 196.4017061176955963 ) ) ;
#93101=AXIS2_PLACEMENT_3D ( 'NONE', #1193, #1751, #26361 ) ;
#93104=CARTESIAN_POINT ( 'NONE',  ( -16.64685983873495445, 1523.847233649538339, 237.7436688609939779 ) ) ;
#93117=AXIS2_PLACEMENT_3D ( 'NONE', #52354, #9766, #35521 ) ;
#93120=CARTESIAN_POINT ( 'NONE',  ( 17.03783583027156823, 1524.776010967676029, 237.1517449984523864 ) ) ;
#93135=ORIENTED_EDGE ( 'NONE', *, *, #67838, .T. ) ;
#93153=ORIENTED_EDGE ( 'NONE', *, *, #27349, .T. ) ;
#93155=ORIENTED_EDGE ( 'NONE', *, *, #89048, .T. ) ;
#93160=DIRECTION ( 'NONE',  ( 0.000000000000000000, 1.000000000000000000, 0.000000000000000000 ) ) ;
#93178=EDGE_CURVE ( 'NONE', #58183, #88502, #26954, .T. ) ;
#93179=CARTESIAN_POINT ( 'NONE',  ( 22.66254714602377973, 1523.342713519622293, 181.4291743802665735 ) ) ;
#93180=EDGE_CURVE ( 'NONE', #44004, #18098, #33759, .T. ) ;
#93192=ORIENTED_EDGE ( 'NONE', *, *, #67340, .F. ) ;
#93196=CARTESIAN_POINT ( 'NONE',  ( -32.02808312589930040, 1512.187213306747481, 198.2787714533499752 ) ) ;
#93201=DIRECTION ( 'NONE',  ( 0.000000000000000000, 0.000000000000000000, -1.000000000000000000 ) ) ;
#93202=DIRECTION ( 'NONE',  ( -0.4978433412588781914, 0.000000000000000000, -0.8672669759446606230 ) ) ;
#93209=EDGE_CURVE ( 'NONE', #13899, #38713, #89526, .T. ) ;
#93211=CARTESIAN_POINT ( 'NONE',  ( -33.72300830903702717, 1524.397344074318198, 219.5868698111212609 ) ) ;
#93213=( BOUNDED_SURFACE ( )  B_SPLINE_SURFACE ( 3, 2, ( 
 ( #56082, #89126, #81261 ),
 ( #41347, #11876, #65036 ),
 ( #47682, #63954, #12413 ),
 ( #13491, #81810, #5112 ),
 ( #39268, #97529, #92285 ),
 ( #63414, #88593, #98068 ) ),
 .UNSPECIFIED., .F., .F., .F. ) 
 B_SPLINE_SURFACE_WITH_KNOTS ( ( 4, 2, 4 ),
 ( 3, 3 ),
 ( -5.139118297581291017E-17, 0.001312027981647291563, 0.002624055963294634301 ),
 ( 0.000000000000000000, 1.000000000000000000 ),
 .UNSPECIFIED. ) 
 GEOMETRIC_REPRESENTATION_ITEM ( )  RATIONAL_B_SPLINE_SURFACE ( (
 ( 1.000000000000000000, 0.9376006582765908925, 1.000000000000000000),
 ( 1.000000000000000000, 0.9569320108021285298, 1.000000000000000000),
 ( 1.000000000000000000, 0.9725743441620615659, 1.000000000000000000),
 ( 1.000000000000000000, 0.9942095667133905579, 1.000000000000000000),
 ( 1.000000000000000000, 1.000043666450838531, 1.000000000000000000),
 ( 1.000000000000000000, 1.000000000000000000, 1.000000000000000000) ) ) 
 REPRESENTATION_ITEM ( '' )  SURFACE ( )  );
#93223=CARTESIAN_POINT ( 'NONE',  ( 19.98413504154914122, 1526.143142182216479, 184.9530087056776040 ) ) ;
#93225=LINE ( 'NONE', #42836, #77893 ) ;
#93226=ORIENTED_EDGE ( 'NONE', *, *, #83473, .T. ) ;
#93238=ADVANCED_FACE ( 'NONE', ( #25903 ), #57584, .T. ) ;
#93243=ORIENTED_EDGE ( 'NONE', *, *, #86399, .T. ) ;
#93254=EDGE_CURVE ( 'NONE', #32804, #1550, #18222, .T. ) ;
#93256=CARTESIAN_POINT ( 'NONE',  ( -21.83550407203936672, 1523.678648413191695, 183.2743720722710634 ) ) ;
#93258=CARTESIAN_POINT ( 'NONE',  ( -2.425477467416652377, 1523.390106123591067, 243.0915840373788228 ) ) ;
#93266=ORIENTED_EDGE ( 'NONE', *, *, #71459, .F. ) ;
#93271=DIRECTION ( 'NONE',  ( -1.000000000000000000, 0.000000000000000000, 0.000000000000000000 ) ) ;
#93280=ORIENTED_EDGE ( 'NONE', *, *, #75537, .T. ) ;
#93285=TOROIDAL_SURFACE ( 'NONE', #71849, 2.000000000000000000, 1.000000000000000000 ) ;
#93287=CARTESIAN_POINT ( 'NONE',  ( 21.96543842109161204, 1523.313115944345327, 182.9844783913649451 ) ) ;
#93295=AXIS2_PLACEMENT_3D ( 'NONE', #83979, #40324, #23518 ) ;
#93307=ADVANCED_FACE ( 'NONE', ( #70733 ), #47152, .T. ) ;
#93313=CARTESIAN_POINT ( 'NONE',  ( -20.71343476517490956, 1524.726013923371283, 238.3377464195766038 ) ) ;
#93338=CARTESIAN_POINT ( 'NONE',  ( 2.487422374635116284, 1523.954924407802764, 175.4471440611261244 ) ) ;
#93343=DIRECTION ( 'NONE',  ( 0.9774101051267758411, 0.000000000000000000, -0.2113515706023144369 ) ) ;
#93356=CARTESIAN_POINT ( 'NONE',  ( -20.20959865099451847, 1512.187213306747481, 236.2316688286741453 ) ) ;
#93357=CARTESIAN_POINT ( 'NONE',  ( -2.157496122451409537, 1526.189892541618974, 177.9627121745355396 ) ) ;
#93424=LINE ( 'NONE', #50357, #20306 ) ;
#93444=CARTESIAN_POINT ( 'NONE',  ( -21.38516915558007270, 1501.977400791986611, 180.3939891059723664 ) ) ;
#93456=CARTESIAN_POINT ( 'NONE',  ( -16.49514911236800785, 1525.343710797494396, 181.2134097543055020 ) ) ;
#93458=FACE_OUTER_BOUND ( 'NONE', #62154, .T. ) ;
#93471=EDGE_CURVE ( 'NONE', #63441, #13894, #60948, .T. ) ;
#93486=CARTESIAN_POINT ( 'NONE',  ( -33.42844755917176514, 1501.977400791986611, 222.1271778627171045 ) ) ;
#93494=EDGE_LOOP ( 'NONE', ( #27615, #99183, #41745, #2450 ) ) ;
#93495=CARTESIAN_POINT ( 'NONE',  ( 2.157482617120738855, 1526.189899547014647, 177.9627270532062937 ) ) ;
#93502=CARTESIAN_POINT ( 'NONE',  ( 2.620401159595450391, 1523.462669333491931, 176.0805060895404495 ) ) ;
#93508=DIRECTION ( 'NONE',  ( -4.857225732735055447E-14, 0.000000000000000000, 1.000000000000000000 ) ) ;
#93517=CARTESIAN_POINT ( 'NONE',  ( -1.800936940629448868, 1526.306647125542440, 239.8931631715260835 ) ) ;
#93532=CARTESIAN_POINT ( 'NONE',  ( -29.00779973304124582, 1526.382868172864164, 217.2942086403127178 ) ) ;
#93539=DIRECTION ( 'NONE',  ( 0.9942586961433749204, 0.000000000000000000, -0.1070030146457375819 ) ) ;
#93554=EDGE_LOOP ( 'NONE', ( #24707, #50358, #84336, #86290, #46158 ) ) ;
#93565=CARTESIAN_POINT ( 'NONE',  ( 0.000000000000000000, 1512.187213306747481, 209.1218459616979999 ) ) ;
#93575=DIRECTION ( 'NONE',  ( 0.000000000000000000, -1.000000000000000000, -0.000000000000000000 ) ) ;
#93580=CARTESIAN_POINT ( 'NONE',  ( 21.92333112166549469, 1524.538969332612623, 233.6740449069407077 ) ) ;
#93587=CIRCLE ( 'NONE', #59651, 2.000000000000001776 ) ;
#93595=CARTESIAN_POINT ( 'NONE',  ( -21.35000886514797003, 1525.163527997505071, 234.4063825837820048 ) ) ;
#93603=CARTESIAN_POINT ( 'NONE',  ( -22.75273496409560181, 1523.382868172864164, 234.5707981297189519 ) ) ;
#93618=DIRECTION ( 'NONE',  ( 0.000000000000000000, 0.000000000000000000, 1.000000000000000000 ) ) ;
#93633=CARTESIAN_POINT ( 'NONE',  ( 30.24842679174819082, 1524.082582765195411, 195.7700791222141845 ) ) ;
#93648=CARTESIAN_POINT ( 'NONE',  ( 16.51370628721609179, 1525.137881624894590, 181.0453264504938602 ) ) ;
#93651=DIRECTION ( 'NONE',  ( 0.000000000000000000, 0.000000000000000000, -1.000000000000000000 ) ) ;
#93657=AXIS2_PLACEMENT_3D ( 'NONE', #69368, #96761, #88898 ) ;
#93677=DIRECTION ( 'NONE',  ( -0.000000000000000000, -1.000000000000000000, -0.000000000000000000 ) ) ;
#93681=B_SPLINE_CURVE_WITH_KNOTS ( 'NONE', 3,
 ( #28202, #3035, #2486, #70802, #97072, #54543, #11954, #80269, #3584, #71909 ),
 .UNSPECIFIED., .F., .F.,
 ( 4, 2, 2, 2, 4 ),
 ( 3.122502256758252770E-17, 0.0007406479101619058971, 0.001481295820323780569, 0.002221943730485655133, 0.002962591640647529913 ),
 .UNSPECIFIED. ) ;
#93706=CARTESIAN_POINT ( 'NONE',  ( 19.53786426059039982, 1512.187213306747481, 236.7197124308265188 ) ) ;
#93716=CARTESIAN_POINT ( 'NONE',  ( 21.61625474793712343, 1526.178928173327904, 183.7635344381618268 ) ) ;
#93739=ORIENTED_EDGE ( 'NONE', *, *, #74320, .F. ) ;
#93745=CARTESIAN_POINT ( 'NONE',  ( -34.61172972909704981, 1523.342713519622976, 218.2049768989091376 ) ) ;
#93755=CARTESIAN_POINT ( 'NONE',  ( -21.59934095315038860, 1525.137881624895044, 184.7402563171935128 ) ) ;
#93775=VECTOR ( 'NONE', #67740, 1000.000000000000000 ) ;
#93805=CARTESIAN_POINT ( 'NONE',  ( 2.390047989666873818, 1526.069472839378705, 240.5369618407319763 ) ) ;
#93808=LINE ( 'NONE', #15453, #100483 ) ;
#93821=CARTESIAN_POINT ( 'NONE',  ( 17.84338787571943641, 1523.382868172864164, 237.8836641337660467 ) ) ;
#93847=EDGE_CURVE ( 'NONE', #63792, #107214, #93808, .T. ) ;
#93853=CARTESIAN_POINT ( 'NONE',  ( -29.79244380916537338, 1525.556090473913855, 221.4001982487179419 ) ) ;
#93858=CARTESIAN_POINT ( 'NONE',  ( 2.470955845399089856, 1523.580203803270933, 242.8749759691355621 ) ) ;
#93862=ORIENTED_EDGE ( 'NONE', *, *, #87166, .F. ) ;
#93874=CARTESIAN_POINT ( 'NONE',  ( -33.93019615848938741, 1512.187213306747481, 220.5829544587966211 ) ) ;
#93883=ADVANCED_FACE ( 'NONE', ( #23854 ), #58046, .F. ) ;
#93898=CARTESIAN_POINT ( 'NONE',  ( 2.580915939757335131, 1524.130440953581001, 242.3512492075526836 ) ) ;
#93905=CARTESIAN_POINT ( 'NONE',  ( 28.27139721233034209, 1526.382868172864164, 219.5606225550385204 ) ) ;
#93911=EDGE_CURVE ( 'NONE', #18098, #39550, #55830, .T. ) ;
#93922=CARTESIAN_POINT ( 'NONE',  ( 30.90487439922556945, 1525.907212628473644, 201.8101144455177689 ) ) ;
#93925=DIRECTION ( 'NONE',  ( 0.000000000000000000, 1.000000000000000000, 0.000000000000000000 ) ) ;
#93940=CIRCLE ( 'NONE', #79678, 23.69926344187880929 ) ;
#93972=EDGE_CURVE ( 'NONE', #100188, #55613, #338, .T. ) ;
#93979=EDGE_LOOP ( 'NONE', ( #70023, #19878, #55995, #78001 ) ) ;
#93984=ORIENTED_EDGE ( 'NONE', *, *, #61862, .T. ) ;
#94004=ORIENTED_EDGE ( 'NONE', *, *, #84469, .T. ) ;
#94020=EDGE_LOOP ( 'NONE', ( #65549, #49795, #95928, #95467 ) ) ;
#94021=CARTESIAN_POINT ( 'NONE',  ( -0.8350686643532192477, 1524.382868172863937, 177.3106345060153046 ) ) ;
#94024=VECTOR ( 'NONE', #62463, 1000.000000000000114 ) ;
#94037=DIRECTION ( 'NONE',  ( 0.000000000000000000, 1.000000000000000000, 0.000000000000000000 ) ) ;
#94051=EDGE_LOOP ( 'NONE', ( #69358, #12482, #97906, #44877 ) ) ;
#94052=CARTESIAN_POINT ( 'NONE',  ( 1.191524307911311586, 1526.382868172863937, 179.0083900503167911 ) ) ;
#94061=CARTESIAN_POINT ( 'NONE',  ( -16.62993785878394348, 1526.306647125543122, 183.1687632256341658 ) ) ;
#94075=DIRECTION ( 'NONE',  ( 0.000000000000000000, 1.000000000000000000, 0.000000000000000000 ) ) ;
#94080=FACE_OUTER_BOUND ( 'NONE', #46988, .T. ) ;
#94096=TOROIDAL_SURFACE ( 'NONE', #88774, 2.000000000000000000, 1.000000000000000000 ) ;
#94117=ORIENTED_EDGE ( 'NONE', *, *, #89772, .F. ) ;
#94134=VERTEX_POINT ( 'NONE', #44083 ) ;
#94137=ORIENTED_EDGE ( 'NONE', *, *, #54235, .T. ) ;
#94151=ADVANCED_FACE ( 'NONE', ( #988 ), #107915, .F. ) ;
#94153=VERTEX_POINT ( 'NONE', #86073 ) ;
#94156=CARTESIAN_POINT ( 'NONE',  ( -17.07724394729179096, 1524.330813522192102, 181.0533268958121766 ) ) ;
#94165=DIRECTION ( 'NONE',  ( 0.000000000000000000, -1.000000000000000000, 0.000000000000000000 ) ) ;
#94181=CARTESIAN_POINT ( 'NONE',  ( 32.23107245336971260, 1523.542365884047740, 216.8383915158461548 ) ) ;
#94190=VERTEX_POINT ( 'NONE', #61453 ) ;
#94202=CARTESIAN_POINT ( 'NONE',  ( 3.448830483803561719, 1523.382868172864164, 243.0842028158767789 ) ) ;
#94207=DIRECTION ( 'NONE',  ( 0.5877852522924853496, 0.000000000000000000, 0.8090169943749385695 ) ) ;
#94212=CARTESIAN_POINT ( 'NONE',  ( 16.57702445344274977, 1524.523992613119390, 180.6870595316466677 ) ) ;
#94229=AXIS2_PLACEMENT_3D ( 'NONE', #89783, #21994, #99823 ) ;
#94232=ORIENTED_EDGE ( 'NONE', *, *, #28441, .T. ) ;
#94234=CARTESIAN_POINT ( 'NONE',  ( 21.11882185302462389, 1525.651285554131618, 184.9294391855967490 ) ) ;
#94239=DIRECTION ( 'NONE',  ( -0.000000000000000000, -1.000000000000000000, -0.000000000000000000 ) ) ;
#94254=ORIENTED_EDGE ( 'NONE', *, *, #27940, .T. ) ;
#94284=CARTESIAN_POINT ( 'NONE',  ( 21.95372433850586802, 1524.425415513990629, 184.5473008717370931 ) ) ;
#94288=CARTESIAN_POINT ( 'NONE',  ( 30.83402112501738657, 1524.872178180564561, 221.7254380314573723 ) ) ;
#94296=CARTESIAN_POINT ( 'NONE',  ( -31.34137657934027388, 1523.382868172864164, 196.3411265156551906 ) ) ;
#94300=DIRECTION ( 'NONE',  ( 0.000000000000000000, 1.000000000000000000, 0.000000000000000000 ) ) ;
#94316=CARTESIAN_POINT ( 'NONE',  ( -21.51513853577911917, 1524.871836253796118, 183.6915109491697535 ) ) ;
#94317=( BOUNDED_CURVE ( )  B_SPLINE_CURVE ( 3, ( #34164, #102456, #68904, #6747 ),
 .UNSPECIFIED., .F., .F. ) 
 B_SPLINE_CURVE_WITH_KNOTS ( ( 4, 4 ),
 ( 0.000000000000000000, 0.7048113239778065475 ),
 .UNSPECIFIED. ) 
 CURVE ( )  GEOMETRIC_REPRESENTATION_ITEM ( )  RATIONAL_B_SPLINE_CURVE ( ( 1.000000000000000000, 0.9590300661663091475, 0.9590300661663091475, 1.000000000000000000 ) ) 
 REPRESENTATION_ITEM ( '' )  );
#94319=ORIENTED_EDGE ( 'NONE', *, *, #54820, .T. ) ;
#94335=VERTEX_POINT ( 'NONE', #95029 ) ;
#94342=CARTESIAN_POINT ( 'NONE',  ( 34.68852446352940433, 1501.977400791986611, 199.9946320047950223 ) ) ;
#94347=CARTESIAN_POINT ( 'NONE',  ( -2.456601303385831159, 1523.611961620354123, 242.9433449337721243 ) ) ;
#94353=ORIENTED_EDGE ( 'NONE', *, *, #70326, .F. ) ;
#94354=ORIENTED_EDGE ( 'NONE', *, *, #48204, .F. ) ;
#94361=CARTESIAN_POINT ( 'NONE',  ( -32.79520279071641653, 1523.954914175594695, 201.0814687157684091 ) ) ;
#94381=AXIS2_PLACEMENT_3D ( 'NONE', #51687, #101499, #93651 ) ;
#94382=EDGE_LOOP ( 'NONE', ( #4325, #74384, #99085, #92073 ) ) ;
#94400=AXIS2_PLACEMENT_3D ( 'NONE', #76158, #7841, #84000 ) ;
#94432=CARTESIAN_POINT ( 'NONE',  ( 2.664527636416277989, 1524.964230758899930, 176.5361228849588997 ) ) ;
#94439=DIRECTION ( 'NONE',  ( 0.4090087482554383702, 0.000000000000000000, 0.9125304618753937724 ) ) ;
#94449=AXIS2_PLACEMENT_3D ( 'NONE', #99967, #109494, #58547 ) ;
#94453=AXIS2_PLACEMENT_3D ( 'NONE', #24060, #94037, #43102 ) ;
#94503=EDGE_CURVE ( 'NONE', #76626, #32282, #28377, .T. ) ;
#94518=FACE_OUTER_BOUND ( 'NONE', #20686, .T. ) ;
#94525=ORIENTED_EDGE ( 'NONE', *, *, #102669, .F. ) ;
#94532=ORIENTED_EDGE ( 'NONE', *, *, #52210, .F. ) ;
#94546=ORIENTED_EDGE ( 'NONE', *, *, #42536, .F. ) ;
#94559=CARTESIAN_POINT ( 'NONE',  ( 30.00400320040656510, 1524.843178112495480, 195.9692341599732686 ) ) ;
#94562=EDGE_CURVE ( 'NONE', #4626, #30502, #37747, .T. ) ;
#94598=ADVANCED_FACE ( 'NONE', ( #101732 ), #92871, .F. ) ;
#94606=CARTESIAN_POINT ( 'NONE',  ( -32.28351601132079196, 1524.972613296805093, 217.0406166517271060 ) ) ;
#94619=CARTESIAN_POINT ( 'NONE',  ( 0.000000000000000000, 1511.187213306747708, 209.1218459616979999 ) ) ;
#94625=VERTEX_POINT ( 'NONE', #67618 ) ;
#94654=ORIENTED_EDGE ( 'NONE', *, *, #73891, .T. ) ;
#94663=DIRECTION ( 'NONE',  ( 0.9510565162951561957, 0.000000000000000000, 0.3090169943749392911 ) ) ;
#94664=AXIS2_PLACEMENT_3D ( 'NONE', #68776, #1017, #109653 ) ;
#94692=ORIENTED_EDGE ( 'NONE', *, *, #5258, .T. ) ;
#94696=CARTESIAN_POINT ( 'NONE',  ( 29.00779973304130266, 1526.382868172863937, 200.9494832830834810 ) ) ;
#94701=CIRCLE ( 'NONE', #78648, 1.000000000000000888 ) ;
#94713=EDGE_LOOP ( 'NONE', ( #42859, #72106, #63335, #72028 ) ) ;
#94715=CARTESIAN_POINT ( 'NONE',  ( 29.35072644275232179, 1526.211528530236592, 197.7230832643897713 ) ) ;
#94728=EDGE_CURVE ( 'NONE', #24039, #9564, #19945, .T. ) ;
#94729=CARTESIAN_POINT ( 'NONE',  ( -2.038646110889678287, 1525.960063244516959, 241.1857569150893994 ) ) ;
#94741=FACE_OUTER_BOUND ( 'NONE', #8968, .T. ) ;
#94758=CARTESIAN_POINT ( 'NONE',  ( 20.49599333844873783, 1525.960063244516959, 233.8638087104922931 ) ) ;
#94760=CARTESIAN_POINT ( 'NONE',  ( 29.85692247043846237, 1525.159196711359755, 196.1177113527152187 ) ) ;
#94768=CARTESIAN_POINT ( 'NONE',  ( -18.98249322452759813, 1526.382868172864164, 185.2725498412215188 ) ) ;
#94784=CIRCLE ( 'NONE', #109107, 2.000000000000001776 ) ;
#94786=ADVANCED_FACE ( 'NONE', ( #32759 ), #76420, .T. ) ;
#94787=CARTESIAN_POINT ( 'NONE',  ( -30.60907494343237190, 1526.073429442291854, 201.6841126651373770 ) ) ;
#94795=AXIS2_PLACEMENT_3D ( 'NONE', #12265, #31827, #98476 ) ;
#94796=FILL_AREA_STYLE ('',( #60668 ) ) ;
#94803=ORIENTED_EDGE ( 'NONE', *, *, #81678, .F. ) ;
#94817=VERTEX_POINT ( 'NONE', #7561 ) ;
#94824=AXIS2_PLACEMENT_3D ( 'NONE', #109491, #42835, #26000 ) ;
#94846=DIRECTION ( 'NONE',  ( -1.734723475976805517E-14, 0.000000000000000000, 1.000000000000000000 ) ) ;
#94849=CARTESIAN_POINT ( 'NONE',  ( 22.69876404240077505, 1522.382868172864164, 181.3483716558180276 ) ) ;
#94859=CARTESIAN_POINT ( 'NONE',  ( 30.00389853323147804, 1524.843416604514459, 222.2743556717897775 ) ) ;
#94865=CARTESIAN_POINT ( 'NONE',  ( 18.66420869458061205, 1526.382868172863937, 232.7837831374278039 ) ) ;
#94888=CARTESIAN_POINT ( 'NONE',  ( -1.191524307911315583, 1526.382868172863937, 239.2353018730792087 ) ) ;
#94891=CYLINDRICAL_SURFACE ( 'NONE', #95713, 1.999999999999995559 ) ;
#94900=CARTESIAN_POINT ( 'NONE',  ( 30.04822308544829212, 1524.382868172804365, 196.4802968571190149 ) ) ;
#94903=DIRECTION ( 'NONE',  ( 0.000000000000000000, 0.8724564897876576630, -0.4886917979948086077 ) ) ;
#94906=EDGE_CURVE ( 'NONE', #75901, #73175, #24883, .T. ) ;
#94911=AXIS2_PLACEMENT_3D ( 'NONE', #37822, #21535, #12059 ) ;
#94918=CYLINDRICAL_SURFACE ( 'NONE', #87213, 2.000000000000001776 ) ;
#94931=EDGE_LOOP ( 'NONE', ( #49577, #5980, #26239, #105742 ) ) ;
#94952=ORIENTED_EDGE ( 'NONE', *, *, #47370, .F. ) ;
#94961=VECTOR ( 'NONE', #69241, 1000.000000000000000 ) ;
#94965=DIRECTION ( 'NONE',  ( -0.000000000000000000, -1.000000000000000000, -0.000000000000000000 ) ) ;
#94981=CARTESIAN_POINT ( 'NONE',  ( -30.64459234690422207, 1525.163457223743762, 221.6135952602373891 ) ) ;
#94991=CIRCLE ( 'NONE', #25181, 1.000000000000000888 ) ;
#95013=CARTESIAN_POINT ( 'NONE',  ( -34.18677586421193837, 1522.382868172863937, 198.4504086008750505 ) ) ;
#95014=CARTESIAN_POINT ( 'NONE',  ( -21.83550407203883736, 1523.678648413191695, 234.9693198511253627 ) ) ;
#95028=( GEOMETRIC_REPRESENTATION_CONTEXT ( 3 ) GLOBAL_UNCERTAINTY_ASSIGNED_CONTEXT ( ( #110701 ) ) GLOBAL_UNIT_ASSIGNED_CONTEXT ( ( #31586, #32697, #100987 ) ) REPRESENTATION_CONTEXT ( 'NONE', 'WORKASPACE' ) );
#95029=CARTESIAN_POINT ( 'NONE',  ( 16.16632277704777110, 1511.187213306747708, 181.3470724465435637 ) ) ;
#95048=CARTESIAN_POINT ( 'NONE',  ( 29.00779973304130266, 1526.382868172863937, 200.9494832830834810 ) ) ;
#95054=CIRCLE ( 'NONE', #107597, 1.000000000000000888 ) ;
#95063=CARTESIAN_POINT ( 'NONE',  ( 1.393816646507355150, 1512.187213306747481, 243.1385343369520342 ) ) ;
#95070=CARTESIAN_POINT ( 'NONE',  ( -29.00779973304142345, 1526.382868172863937, 200.9494832830838789 ) ) ;
#95090=CARTESIAN_POINT ( 'NONE',  ( -2.646294106703095395, 1525.055402519452173, 176.5934494553323191 ) ) ;
#95091=FACE_OUTER_BOUND ( 'NONE', #43944, .T. ) ;
#95103=ORIENTED_EDGE ( 'NONE', *, *, #37265, .F. ) ;
#95108=B_SPLINE_CURVE_WITH_KNOTS ( 'NONE', 3,
 ( #75086, #49878, #103005, #94061, #25743, #75637, #51523, #59393 ),
 .UNSPECIFIED., .F., .F.,
 ( 4, 2, 2, 4 ),
 ( 0.000000000000000000, 0.001073044933456172596, 0.001609567400184299226, 0.002146089866912425856 ),
 .UNSPECIFIED. ) ;
#95124=ADVANCED_FACE ( 'NONE', ( #60756 ), #86471, .F. ) ;
#95141=CARTESIAN_POINT ( 'NONE',  ( 21.98490254033135827, 1525.713797967456912, 235.3026395021878159 ) ) ;
#95148=CARTESIAN_POINT ( 'NONE',  ( -28.35863496383681692, 1526.382868172863482, 198.5269487343526293 ) ) ;
#95175=EDGE_CURVE ( 'NONE', #89888, #83385, #103252, .T. ) ;
#95178=VERTEX_POINT ( 'NONE', #45614 ) ;
#95184=CARTESIAN_POINT ( 'NONE',  ( -21.41971086555123449, 1512.187213306747481, 185.1638823089581081 ) ) ;
#95189=VERTEX_POINT ( 'NONE', #80841 ) ;
#95194=ORIENTED_EDGE ( 'NONE', *, *, #21547, .T. ) ;
#95209=CARTESIAN_POINT ( 'NONE',  ( -2.404980717409123336, 1525.211477436245787, 176.1486445165030545 ) ) ;
#95210=EDGE_CURVE ( 'NONE', #10931, #76626, #37013, .T. ) ;
#95215=CARTESIAN_POINT ( 'NONE',  ( 3.614551905308796432E-15, 1526.382868172863937, 179.6067898016248421 ) ) ;
#95217=DIRECTION ( 'NONE',  ( 0.000000000000000000, 1.000000000000000000, 0.000000000000000000 ) ) ;
#95247=VERTEX_POINT ( 'NONE', #48354 ) ;
#95250=ORIENTED_EDGE ( 'NONE', *, *, #68617, .F. ) ;
#95274=ORIENTED_EDGE ( 'NONE', *, *, #13794, .F. ) ;
#95278=CARTESIAN_POINT ( 'NONE',  ( -19.37774363895756480, 1525.878013734321485, 181.3897518523461656 ) ) ;
#95300=EDGE_CURVE ( 'NONE', #24484, #40850, #63814, .T. ) ;
#95304=CARTESIAN_POINT ( 'NONE',  ( 32.86470156657996000, 1523.580204110581690, 217.2021180770844069 ) ) ;
#95316=CARTESIAN_POINT ( 'NONE',  ( 19.37374569213945463, 1526.382868172863937, 234.3668155954418637 ) ) ;
#95335=CARTESIAN_POINT ( 'NONE',  ( 19.53786426059039982, 1522.382868172863937, 236.7197124308265188 ) ) ;
#95342=DIRECTION ( 'NONE',  ( 0.8090169943749551118, 0.000000000000000000, 0.5877852522924625900 ) ) ;
#95348=CARTESIAN_POINT ( 'NONE',  ( -30.90487439922555879, 1525.907212628473644, 201.8101144455182521 ) ) ;
#95366=EDGE_CURVE ( 'NONE', #16677, #34471, #4096, .T. ) ;
#95376=ADVANCED_FACE ( 'NONE', ( #19686 ), #99577, .T. ) ;
#95389=ADVANCED_FACE ( 'NONE', ( #94741 ), #35644, .F. ) ;
#95408=CARTESIAN_POINT ( 'NONE',  ( 21.38516915557986309, 1522.382868172863937, 237.8497028174237471 ) ) ;
#95417=CARTESIAN_POINT ( 'NONE',  ( 31.32995031131201458, 1523.678648413191695, 221.9013357025043831 ) ) ;
#95434=ADVANCED_FACE ( 'NONE', ( #99127 ), #105919, .T. ) ;
#95439=DIRECTION ( 'NONE',  ( 0.000000000000000000, 1.000000000000000000, 0.000000000000000000 ) ) ;
#95440=CARTESIAN_POINT ( 'NONE',  ( -19.54391504031712401, 1526.306647125542668, 232.9578003497408361 ) ) ;
#95447=ORIENTED_EDGE ( 'NONE', *, *, #91834, .T. ) ;
#95449=AXIS2_PLACEMENT_3D ( 'NONE', #55462, #104196, #20717 ) ;
#95457=VECTOR ( 'NONE', #86301, 1000.000000000000000 ) ;
#95467=ORIENTED_EDGE ( 'NONE', *, *, #94503, .F. ) ;
#95484=CARTESIAN_POINT ( 'NONE',  ( -3.448830483803564828, 1511.187213306747708, 175.1594891075192209 ) ) ;
#95488=CARTESIAN_POINT ( 'NONE',  ( -31.30542346655892771, 1525.651286436460396, 201.9631088232815443 ) ) ;
#95496=ORIENTED_EDGE ( 'NONE', *, *, #104098, .F. ) ;
#95512=EDGE_CURVE ( 'NONE', #32804, #8029, #104220, .T. ) ;
#95517=FACE_OUTER_BOUND ( 'NONE', #22063, .T. ) ;
#95537=CARTESIAN_POINT ( 'NONE',  ( 21.84020450222056908, 1523.382868172864164, 234.9798068779740277 ) ) ;
#95543=LINE ( 'NONE', #44606, #2877 ) ;
#95550=ORIENTED_EDGE ( 'NONE', *, *, #74187, .T. ) ;
#95558=EDGE_CURVE ( 'NONE', #4524, #105727, #21856, .T. ) ;
#95565=CARTESIAN_POINT ( 'NONE',  ( 17.84338787571921614, 1523.382868172864164, 180.3600277896298110 ) ) ;
#95566=CARTESIAN_POINT ( 'NONE',  ( -16.66936639845670598, 1523.382868172864164, 180.4828114240741854 ) ) ;
#95617=DIRECTION ( 'NONE',  ( 0.6709778558543610938, 0.000000000000000000, -0.7414773880254772465 ) ) ;
#95634=CARTESIAN_POINT ( 'NONE',  ( -18.86688640473562373, 1511.187213306747708, 237.4611898188522332 ) ) ;
#95636=CARTESIAN_POINT ( 'NONE',  ( 19.53786426059019021, 1511.187213306747708, 181.5239794925693388 ) ) ;
#95653=VERTEX_POINT ( 'NONE', #4015 ) ;
#95671=ORIENTED_EDGE ( 'NONE', *, *, #91834, .F. ) ;
#95689=CARTESIAN_POINT ( 'NONE',  ( 3.177699364621945133, 1525.042337199240137, 241.6057670631459473 ) ) ;
#95691=FACE_OUTER_BOUND ( 'NONE', #84967, .T. ) ;
#95692=CARTESIAN_POINT ( 'NONE',  ( 20.38673671613172900, 1525.878013734320803, 236.1208636900216788 ) ) ;
#95698=CARTESIAN_POINT ( 'NONE',  ( -28.62143996450560834, 1526.335487865669165, 198.0561880438515914 ) ) ;
#95699=DIRECTION ( 'NONE',  ( -0.07713599384728302144, -0.9969860201949398704, 0.008301444997534872250 ) ) ;
#95706=CARTESIAN_POINT ( 'NONE',  ( 0.000000000000000000, 1512.187213306747481, 209.1218459616979999 ) ) ;
#95707=CARTESIAN_POINT ( 'NONE',  ( -1.689251544525047333, 1526.344110814223541, 239.7716210576163576 ) ) ;
#95713=AXIS2_PLACEMENT_3D ( 'NONE', #18711, #16492, #17596 ) ;
#95730=DIRECTION ( 'NONE',  ( 0.000000000000000000, 0.000000000000000000, 1.000000000000000000 ) ) ;
#95737=DIRECTION ( 'NONE',  ( -0.000000000000000000, -1.000000000000000000, -0.000000000000000000 ) ) ;
#95741=DIRECTION ( 'NONE',  ( 0.000000000000000000, 1.000000000000000000, 0.000000000000000000 ) ) ;
#95749=CARTESIAN_POINT ( 'NONE',  ( -31.55762699681115180, 1523.390106123591067, 221.9258384720632478 ) ) ;
#95751=CARTESIAN_POINT ( 'NONE',  ( 32.28351601132058590, 1524.972613296804866, 201.2030752716693485 ) ) ;
#95768=AXIS2_PLACEMENT_3D ( 'NONE', #40647, #74277, #58567 ) ;
#95777=VERTEX_POINT ( 'NONE', #16218 ) ;
#95797=ORIENTED_EDGE ( 'NONE', *, *, #5805, .T. ) ;
#95824=DIRECTION ( 'NONE',  ( 0.9942586961433743653, 0.000000000000000000, -0.1070030146457445208 ) ) ;
#95826=ORIENTED_EDGE ( 'NONE', *, *, #24225, .F. ) ;
#95837=EDGE_CURVE ( 'NONE', #91956, #74589, #88814, .T. ) ;
#95838=DIRECTION ( 'NONE',  ( 0.000000000000000000, 0.000000000000000000, -1.000000000000000000 ) ) ;
#95842=CARTESIAN_POINT ( 'NONE',  ( -31.97190655716442009, 1524.330813522192102, 216.6896206998355296 ) ) ;
#95850=CARTESIAN_POINT ( 'NONE',  ( 0.000000000000000000, 1512.187213306747481, 209.1218459616979999 ) ) ;
#95872=CIRCLE ( 'NONE', #40479, 1.000000000000000888 ) ;
#95873=DIRECTION ( 'NONE',  ( 0.000000000000000000, 0.000000000000000000, 1.000000000000000000 ) ) ;
#95876=ADVANCED_FACE ( 'NONE', ( #23533 ), #104336, .T. ) ;
#95906=CARTESIAN_POINT ( 'NONE',  ( 21.45464262047749671, 1525.320827368861273, 184.8030334685298044 ) ) ;
#95912=CARTESIAN_POINT ( 'NONE',  ( 1.191524307911315805, 1526.382868172863937, 239.2353018730792087 ) ) ;
#95928=ORIENTED_EDGE ( 'NONE', *, *, #36788, .F. ) ;
#95934=EDGE_CURVE ( 'NONE', #31591, #68013, #65647, .T. ) ;
#95935=DIRECTION ( 'NONE',  ( -0.000000000000000000, -1.000000000000000000, -0.000000000000000000 ) ) ;
#95942=EDGE_LOOP ( 'NONE', ( #84576, #51947, #64389, #104618 ) ) ;
#95999=CARTESIAN_POINT ( 'NONE',  ( -29.78220350812357964, 1524.382868172863937, 196.5089261231635476 ) ) ;
#96011=ORIENTED_EDGE ( 'NONE', *, *, #65850, .F. ) ;
#96014=CARTESIAN_POINT ( 'NONE',  ( 22.03465957474552184, 1512.187213306747481, 182.8300405912328301 ) ) ;
#96019=ADVANCED_FACE ( 'NONE', ( #104402 ), #7836, .T. ) ;
#96047=DIRECTION ( 'NONE',  ( 0.000000000000000000, 1.000000000000000000, 0.000000000000000000 ) ) ;
#96053=DIRECTION ( 'NONE',  ( 0.000000000000000000, 1.000000000000000000, 0.000000000000000000 ) ) ;
#96089=CARTESIAN_POINT ( 'NONE',  ( 20.12564951288285542, 1512.187213306747481, 237.5287294252014192 ) ) ;
#96098=CIRCLE ( 'NONE', #108646, 33.13701971169416538 ) ;
#96099=ORIENTED_EDGE ( 'NONE', *, *, #102990, .T. ) ;
#96103=VERTEX_POINT ( 'NONE', #56205 ) ;
#96127=CARTESIAN_POINT ( 'NONE',  ( -2.340429037510286747, 1525.425665131969026, 241.8895524149548919 ) ) ;
#96146=CARTESIAN_POINT ( 'NONE',  ( 29.33475263078180006, 1526.373507135059754, 201.1007689730743380 ) ) ;
#96152=AXIS2_PLACEMENT_3D ( 'NONE', #70148, #20782, #70700 ) ;
#96154=EDGE_CURVE ( 'NONE', #21147, #55064, #17307, .T. ) ;
#96164=CARTESIAN_POINT ( 'NONE',  ( 3.263276722441742717, 1524.760046179776054, 241.7717505690895052 ) ) ;
#96165=DIRECTION ( 'NONE',  ( 0.1070030146457217196, 0.000000000000000000, -0.9942586961433766968 ) ) ;
#96174=CYLINDRICAL_SURFACE ( 'NONE', #84066, 1.999999999999995337 ) ;
#96189=EDGE_CURVE ( 'NONE', #24269, #89941, #40527, .T. ) ;
#96233=DIRECTION ( 'NONE',  ( -0.2054769195713296304, 0.000000000000000000, -0.9786619618251631847 ) ) ;
#96242=CARTESIAN_POINT ( 'NONE',  ( 30.25425994617003767, 1522.382868172863937, 199.2916410102368729 ) ) ;
#96244=CARTESIAN_POINT ( 'NONE',  ( 21.30823923614806858, 1524.382868172804365, 233.7929508216638510 ) ) ;
#96247=AXIS2_PLACEMENT_3D ( 'NONE', #67729, #67176, #17267 ) ;
#96248=CARTESIAN_POINT ( 'NONE',  ( 32.28466283162156714, 1501.977400791986611, 219.1752493337713190 ) ) ;
#96257=ORIENTED_EDGE ( 'NONE', *, *, #6871, .T. ) ;
#96258=CARTESIAN_POINT ( 'NONE',  ( -29.40443212115373939, 1511.187213306747708, 222.0897836382247306 ) ) ;
#96265=CARTESIAN_POINT ( 'NONE',  ( 0.4151546846821903003, 1512.187213306747481, 243.9330574173806951 ) ) ;
#96284=FACE_OUTER_BOUND ( 'NONE', #9984, .T. ) ;
#96298=ORIENTED_EDGE ( 'NONE', *, *, #62445, .T. ) ;
#96302=EDGE_CURVE ( 'NONE', #49611, #17686, #74882, .T. ) ;
#96304=CARTESIAN_POINT ( 'NONE',  ( -31.02592223166947250, 1526.278758871496620, 219.9652544506489562 ) ) ;
#96319=AXIS2_PLACEMENT_3D ( 'NONE', #108496, #13861, #14416 ) ;
#96395=DIRECTION ( 'NONE',  ( -0.000000000000000000, -1.000000000000000000, -0.000000000000000000 ) ) ;
#96402=CARTESIAN_POINT ( 'NONE',  ( -34.18677586421173942, 1522.382868172863937, 219.7932833225216882 ) ) ;
#96410=CARTESIAN_POINT ( 'NONE',  ( 32.86802468386292020, 1523.382868172864164, 217.2040256693915410 ) ) ;
#96425=TOROIDAL_SURFACE ( 'NONE', #46411, 2.000000000000000000, 1.000000000000000000 ) ;
#96427=CARTESIAN_POINT ( 'NONE',  ( 19.98413504155174181, 1526.143142182265819, 233.2906832177060039 ) ) ;
#96467=CARTESIAN_POINT ( 'NONE',  ( -2.372478608332514671, 1512.187213306747481, 243.3440112565233449 ) ) ;
#96477=ORIENTED_EDGE ( 'NONE', *, *, #49662, .F. ) ;
#96480=ORIENTED_EDGE ( 'NONE', *, *, #87728, .T. ) ;
#96482=VERTEX_POINT ( 'NONE', #77961 ) ;
#96489=CARTESIAN_POINT ( 'NONE',  ( -2.470168521978398868, 1501.977400791986611, 175.3649660270905315 ) ) ;
#96496=ORIENTED_EDGE ( 'NONE', *, *, #9938, .F. ) ;
#96499=ORIENTED_EDGE ( 'NONE', *, *, #98917, .F. ) ;
#96504=CARTESIAN_POINT ( 'NONE',  ( -33.36586802512168504, 1511.187213306747708, 216.3367586934473366 ) ) ;
#96530=EDGE_CURVE ( 'NONE', #20210, #97770, #105939, .T. ) ;
#96551=CARTESIAN_POINT ( 'NONE',  ( -21.64985223704988115, 1524.547395018738143, 183.5513639746648664 ) ) ;
#96552=CARTESIAN_POINT ( 'NONE',  ( 0.8350686643532192477, 1524.382868172863937, 240.9330574173806951 ) ) ;
#96553=ADVANCED_FACE ( 'NONE', ( #56073 ), #16331, .F. ) ;
#96558=DIRECTION ( 'NONE',  ( -0.000000000000000000, -1.000000000000000000, -0.000000000000000000 ) ) ;
#96585=DIRECTION ( 'NONE',  ( -0.000000000000000000, -1.000000000000000000, -0.000000000000000000 ) ) ;
#96591=CARTESIAN_POINT ( 'NONE',  ( -3.347801439296150150, 1523.382868172864164, 242.0893193391992497 ) ) ;
#96612=VERTEX_POINT ( 'NONE', #41479 ) ;
#96613=ORIENTED_EDGE ( 'NONE', *, *, #65808, .T. ) ;
#96633=ORIENTED_EDGE ( 'NONE', *, *, #3780, .F. ) ;
#96648=ORIENTED_EDGE ( 'NONE', *, *, #1576, .T. ) ;
#96653=EDGE_LOOP ( 'NONE', ( #62368, #56336, #25114, #33228 ) ) ;
#96661=EDGE_CURVE ( 'NONE', #61894, #67570, #83433, .T. ) ;
#96666=ORIENTED_EDGE ( 'NONE', *, *, #106740, .F. ) ;
#96669=ORIENTED_EDGE ( 'NONE', *, *, #92115, .F. ) ;
#96675=CARTESIAN_POINT ( 'NONE',  ( -30.99338347248506409, 1526.382868172863937, 199.8717226395886257 ) ) ;
#96682=CARTESIAN_POINT ( 'NONE',  ( -29.00779973304124937, 1526.382868172863937, 217.2942086403127178 ) ) ;
#96683=DIRECTION ( 'NONE',  ( -0.8090169943749507819, 0.000000000000000000, -0.5877852522924685852 ) ) ;
#96685=EDGE_CURVE ( 'NONE', #40573, #41312, #87050, .T. ) ;
#96686=CARTESIAN_POINT ( 'NONE',  ( 2.127574403376955026, 1524.244163922423013, 244.5104606571598538 ) ) ;
#96690=EDGE_CURVE ( 'NONE', #71185, #24039, #38767, .T. ) ;
#96694=DIRECTION ( 'NONE',  ( -0.000000000000000000, -1.000000000000000000, -0.000000000000000000 ) ) ;
#96696=DIRECTION ( 'NONE',  ( 0.8672669759446636206, 0.000000000000000000, 0.4978433412588729734 ) ) ;
#96707=VECTOR ( 'NONE', #33367, 1000.000000000000000 ) ;
#96723=CARTESIAN_POINT ( 'NONE',  ( -20.70484064406422320, 1525.907212628473644, 185.0411015109855839 ) ) ;
#96730=ORIENTED_EDGE ( 'NONE', *, *, #82212, .F. ) ;
#96741=VECTOR ( 'NONE', #22147, 1000.000000000000114 ) ;
#96746=CARTESIAN_POINT ( 'NONE',  ( 31.23437356469435144, 1511.187213306747708, 195.3468678195113739 ) ) ;
#96747=EDGE_LOOP ( 'NONE', ( #61633, #86764, #99705 ) ) ;
#96755=ORIENTED_EDGE ( 'NONE', *, *, #93209, .F. ) ;
#96756=CARTESIAN_POINT ( 'NONE',  ( -2.622430729443011366, 1523.621879633029266, 176.0901726876731743 ) ) ;
#96758=AXIS2_PLACEMENT_3D ( 'NONE', #19670, #9613, #45465 ) ;
#96761=DIRECTION ( 'NONE',  ( 0.4090087482554177756, 1.419034154957278791E-15, -0.9125304618754029873 ) ) ;
#96762=ORIENTED_EDGE ( 'NONE', *, *, #95837, .F. ) ;
#96770=ORIENTED_EDGE ( 'NONE', *, *, #11981, .T. ) ;
#96773=PLANE ( 'NONE',  #106522 ) ;
#96775=CIRCLE ( 'NONE', #62848, 1.000000000000000888 ) ;
#96797=ADVANCED_FACE ( 'NONE', ( #20653 ), #27803, .F. ) ;
#96800=CARTESIAN_POINT ( 'NONE',  ( 2.410659749415533071, 1525.163457223744217, 242.1267480251479753 ) ) ;
#96803=CARTESIAN_POINT ( 'NONE',  ( 22.69876404238873846, 1522.861859112239017, 236.8953202675596401 ) ) ;
#96814=CARTESIAN_POINT ( 'NONE',  ( -32.02808312589908013, 1522.382868172863937, 219.9649204700466782 ) ) ;
#96815=CARTESIAN_POINT ( 'NONE',  ( 0.8350686643532192477, 1526.382868172863937, 240.9330574173806951 ) ) ;
#96833=FACE_OUTER_BOUND ( 'NONE', #36931, .T. ) ;
#96836=CARTESIAN_POINT ( 'NONE',  ( 32.16776790210105474, 1524.538969332612623, 216.0987814432344578 ) ) ;
#96865=CARTESIAN_POINT ( 'NONE',  ( 0.4151546846821903003, 1511.187213306747708, 242.9330574173806951 ) ) ;
#96867=CARTESIAN_POINT ( 'NONE',  ( 31.65140982495767830, 1525.320827368860819, 202.0582358972276609 ) ) ;
#96887=ORIENTED_EDGE ( 'NONE', *, *, #108297, .F. ) ;
#96889=CARTESIAN_POINT ( 'NONE',  ( 17.30126322281391893, 1523.382868172863937, 237.3930845920473303 ) ) ;
#96892=ORIENTED_EDGE ( 'NONE', *, *, #6253, .T. ) ;
#96939=DIRECTION ( 'NONE',  ( -0.9125304618753937724, 0.000000000000000000, 0.4090087482554383147 ) ) ;
#96942=VECTOR ( 'NONE', #71983, 1000.000000000000000 ) ;
#96950=DIRECTION ( 'NONE',  ( 0.000000000000000000, 0.000000000000000000, 1.000000000000000000 ) ) ;
#96977=B_SPLINE_CURVE_WITH_KNOTS ( 'NONE', 3,
 ( #11467, #26022, #18729, #52382 ),
 .UNSPECIFIED., .F., .F.,
 ( 4, 4 ),
 ( 0.000000000000000000, 0.0002220129587134776392 ),
 .UNSPECIFIED. ) ;
#96986=CARTESIAN_POINT ( 'NONE',  ( 19.92151515271066842, 1526.208281990539717, 233.5199663060478201 ) ) ;
#96990=CARTESIAN_POINT ( 'NONE',  ( 33.36586802512179162, 1523.382868172864164, 216.3367586934468818 ) ) ;
#96993=CARTESIAN_POINT ( 'NONE',  ( -3.348647037815419836, 1523.530870145310246, 176.1572109406604625 ) ) ;
#96998=DIRECTION ( 'NONE',  ( 1.387778780781444413E-14, 0.000000000000000000, 1.000000000000000000 ) ) ;
#97021=EDGE_LOOP ( 'NONE', ( #7868, #54767, #107369, #5388, #47010 ) ) ;
#97023=ORIENTED_EDGE ( 'NONE', *, *, #102697, .F. ) ;
#97070=CARTESIAN_POINT ( 'NONE',  ( 29.30029655192942073, 1525.907212628473644, 196.8717316207784620 ) ) ;
#97072=CARTESIAN_POINT ( 'NONE',  ( -32.10254378951861298, 1525.211473355384669, 217.0238571822993379 ) ) ;
#97084=CARTESIAN_POINT ( 'NONE',  ( 29.35747451428154875, 1526.382868173645647, 217.1997937176751350 ) ) ;
#97104=CARTESIAN_POINT ( 'NONE',  ( -17.84338787571901364, 1523.382868172864164, 237.8836641337663309 ) ) ;
#97107=APPLICATION_CONTEXT ( 'automotive_design' ) ;
#97108=DIRECTION ( 'NONE',  ( 0.000000000000000000, 1.000000000000000000, 0.000000000000000000 ) ) ;
#97111=CARTESIAN_POINT ( 'NONE',  ( -29.78220350812360806, 1526.382868172863937, 196.5089261231637181 ) ) ;
#97155=CARTESIAN_POINT ( 'NONE',  ( 21.30909630337538729, 1524.964158026965833, 233.9181086290231235 ) ) ;
#97157=ORIENTED_EDGE ( 'NONE', *, *, #71499, .F. ) ;
#97183=VERTEX_POINT ( 'NONE', #51393 ) ;
#97193=CARTESIAN_POINT ( 'NONE',  ( -3.347801439296141268, 1512.187213306747481, 242.0893193391992497 ) ) ;
#97199=ORIENTED_EDGE ( 'NONE', *, *, #93972, .F. ) ;
#97218=DIRECTION ( 'NONE',  ( 0.9510565162951496454, 0.000000000000000000, -0.3090169943749593862 ) ) ;
#97219=ORIENTED_EDGE ( 'NONE', *, *, #75435, .T. ) ;
#97242=VERTEX_POINT ( 'NONE', #110745 ) ;
#97259=ORIENTED_EDGE ( 'NONE', *, *, #76038, .F. ) ;
#97261=CARTESIAN_POINT ( 'NONE',  ( 30.31940284292409515, 1518.913060387330006, 195.7503880523414352 ) ) ;
#97273=EDGE_CURVE ( 'NONE', #30516, #13874, #33471, .T. ) ;
#97279=DIRECTION ( 'NONE',  ( 0.000000000000000000, 0.000000000000000000, -1.000000000000000000 ) ) ;
#97284=CARTESIAN_POINT ( 'NONE',  ( -0.8350686643532190256, 1526.382868172863937, 240.9330574173806951 ) ) ;
#97287=AXIS2_PLACEMENT_3D ( 'NONE', #20592, #52585, #106278 ) ;
#97332=CARTESIAN_POINT ( 'NONE',  ( 2.708183792730093131, 1524.374142163904480, 241.9870236838057735 ) ) ;
#97335=CARTESIAN_POINT ( 'NONE',  ( 21.13130013988323341, 1524.397344074318880, 237.4101150494052490 ) ) ;
#97342=CARTESIAN_POINT ( 'NONE',  ( -19.37374569213963582, 1526.382868172863937, 183.8768763279542213 ) ) ;
#97353=EDGE_CURVE ( 'NONE', #1550, #49802, #10236, .T. ) ;
#97354=FACE_OUTER_BOUND ( 'NONE', #18823, .T. ) ;
#97357=CIRCLE ( 'NONE', #49111, 1.000000000000000888 ) ;
#97358=CARTESIAN_POINT ( 'NONE',  ( -17.04790460295919630, 1526.208281990536761, 235.6077665793768574 ) ) ;
#97365=EDGE_LOOP ( 'NONE', ( #27079, #52380, #49176, #37672 ) ) ;
#97381=CARTESIAN_POINT ( 'NONE',  ( 3.347801439372898979, 1523.456924617337336, 242.0893193391914622 ) ) ;
#97383=CIRCLE ( 'NONE', #6181, 2.000000000000001776 ) ;
#97390=ORIENTED_EDGE ( 'NONE', *, *, #78951, .F. ) ;
#97399=CARTESIAN_POINT ( 'NONE',  ( -30.51126001304308133, 1526.382868172863937, 219.8557927178091518 ) ) ;
#97404=FACE_OUTER_BOUND ( 'NONE', #63797, .T. ) ;
#97408=CARTESIAN_POINT ( 'NONE',  ( 30.61611611309609415, 1526.069472839382797, 201.6871119896542268 ) ) ;
#97431=FACE_OUTER_BOUND ( 'NONE', #12274, .T. ) ;
#97438=ORIENTED_EDGE ( 'NONE', *, *, #59635, .F. ) ;
#97442=EDGE_CURVE ( 'NONE', #4434, #69179, #51399, .T. ) ;
#97445=CARTESIAN_POINT ( 'NONE',  ( 17.19739463999658113, 1525.960063244516959, 236.2603809477409982 ) ) ;
#97455=ORIENTED_EDGE ( 'NONE', *, *, #54235, .F. ) ;
#97458=CARTESIAN_POINT ( 'NONE',  ( -29.65946186579084909, 1526.335487865669165, 216.9928009627314225 ) ) ;
#97477=CIRCLE ( 'NONE', #49216, 0.9999999999999940048 ) ;
#97480=( BOUNDED_SURFACE ( )  B_SPLINE_SURFACE ( 3, 2, ( 
 ( #91429, #4665, #107674 ),
 ( #55644, #38804, #99247 ),
 ( #72979, #22524, #6313 ),
 ( #74635, #108770, #64043 ),
 ( #14150, #13585, #49434 ),
 ( #15242, #107117, #40460 ) ),
 .UNSPECIFIED., .F., .F., .F. ) 
 B_SPLINE_SURFACE_WITH_KNOTS ( ( 4, 2, 4 ),
 ( 3, 3 ),
 ( -2.471980953266950110E-17, 0.001312027981647300671, 0.002624055963294626061 ),
 ( 0.000000000000000000, 1.000000000000000000 ),
 .UNSPECIFIED. ) 
 GEOMETRIC_REPRESENTATION_ITEM ( )  RATIONAL_B_SPLINE_SURFACE ( (
 ( 1.000000000000000000, 0.9376006582765911146, 1.000000000000000000),
 ( 1.000000000000000000, 0.9569320108021848181, 1.000000000000000000),
 ( 1.000000000000000000, 0.9725743441619884022, 1.000000000000000000),
 ( 1.000000000000000000, 0.9942095667134637216, 1.000000000000000000),
 ( 1.000000000000000000, 1.000043666450783464, 1.000000000000000000),
 ( 1.000000000000000000, 1.000000000000000000, 1.000000000000000000) ) ) 
 REPRESENTATION_ITEM ( '' )  SURFACE ( )  );
#97495=CARTESIAN_POINT ( 'NONE',  ( -21.98490254032901703, 1525.713797967457367, 235.3026395021805683 ) ) ;
#97510=CYLINDRICAL_SURFACE ( 'NONE', #30045, 33.13701971169416538 ) ;
#97522=CARTESIAN_POINT ( 'NONE',  ( -17.30126322281348195, 1523.382868172863937, 237.3930845920475292 ) ) ;
#97529=CARTESIAN_POINT ( 'NONE',  ( 1.389373685229310817, 1526.382868172571079, 178.7050053866609858 ) ) ;
#97551=ADVANCED_FACE ( 'NONE', ( #50013 ), #8460, .T. ) ;
#97553=DIRECTION ( 'NONE',  ( 0.000000000000000000, 0.000000000000000000, 1.000000000000000000 ) ) ;
#97577=EDGE_LOOP ( 'NONE', ( #94137, #49445, #103322, #101558, #6405 ) ) ;
#97593=EDGE_CURVE ( 'NONE', #30075, #91018, #71845, .T. ) ;
#97602=ORIENTED_EDGE ( 'NONE', *, *, #14869, .T. ) ;
#97603=CARTESIAN_POINT ( 'NONE',  ( -17.73223409949403617, 1524.152444737676660, 180.4731695944016678 ) ) ;
#97616=CARTESIAN_POINT ( 'NONE',  ( 22.03465957474570658, 1522.382868172863937, 235.4136513321629991 ) ) ;
#97626=CARTESIAN_POINT ( 'NONE',  ( -17.62880125161998990, 1524.547395018738143, 237.6137924969227413 ) ) ;
#97631=CARTESIAN_POINT ( 'NONE',  ( 16.64885258016843039, 1526.344110814223086, 183.3327398900455592 ) ) ;
#97649=DIRECTION ( 'NONE',  ( -0.9786619618251627406, 0.000000000000000000, -0.2054769195713317953 ) ) ;
#97652=B_SPLINE_CURVE_WITH_KNOTS ( 'NONE', 3,
 ( #86181, #77789, #102961, #25699, #1098, #35226 ),
 .UNSPECIFIED., .F., .F.,
 ( 4, 2, 4 ),
 ( 2.850771429603742560E-17, 0.001087661325621715322, 0.002175322651243402454 ),
 .UNSPECIFIED. ) ;
#97660=DIRECTION ( 'NONE',  ( 1.000000000000000000, -0.000000000000000000, 1.224646799147353207E-16 ) ) ;
#97693=ADVANCED_FACE ( 'NONE', ( #1268 ), #39237, .F. ) ;
#97705=ORIENTED_EDGE ( 'NONE', *, *, #66682, .T. ) ;
#97720=AXIS2_PLACEMENT_3D ( 'NONE', #70767, #84342, #70219 ) ;
#97723=ORIENTED_EDGE ( 'NONE', *, *, #83746, .F. ) ;
#97727=FACE_OUTER_BOUND ( 'NONE', #23776, .T. ) ;
#97757=AXIS2_PLACEMENT_3D ( 'NONE', #101069, #43405, #9247 ) ;
#97770=VERTEX_POINT ( 'NONE', #4032 ) ;
#97776=CARTESIAN_POINT ( 'NONE',  ( -2.664388089261293668, 1523.844789899201942, 242.1314412270628793 ) ) ;
#97800=CYLINDRICAL_SURFACE ( 'NONE', #41107, 1.000000000000000888 ) ;
#97807=ORIENTED_EDGE ( 'NONE', *, *, #37201, .T. ) ;
#97818=CARTESIAN_POINT ( 'NONE',  ( -30.31052258194577931, 1523.604703353109699, 222.4930856806594193 ) ) ;
#97830=AXIS2_PLACEMENT_3D ( 'NONE', #70039, #68928, #104151 ) ;
#97839=CARTESIAN_POINT ( 'NONE',  ( 17.17241001986506888, 1511.187213306747708, 238.6251415217915337 ) ) ;
#97842=EDGE_LOOP ( 'NONE', ( #12796, #68629, #102235, #83020 ) ) ;
#97867=CARTESIAN_POINT ( 'NONE',  ( 32.38601978689629135, 1523.530870145309336, 202.1199661129109586 ) ) ;
#97869=CIRCLE ( 'NONE', #78218, 30.13701971169416183 ) ;
#97872=EDGE_LOOP ( 'NONE', ( #39907, #1233, #44137, #51863 ) ) ;
#97878=EDGE_CURVE ( 'NONE', #54701, #95653, #54323, .T. ) ;
#97890=CARTESIAN_POINT ( 'NONE',  ( -32.36513376976815692, 1523.847233649538339, 202.1343711220893908 ) ) ;
#97906=ORIENTED_EDGE ( 'NONE', *, *, #21343, .F. ) ;
#97911=ORIENTED_EDGE ( 'NONE', *, *, #93972, .T. ) ;
#97913=ORIENTED_EDGE ( 'NONE', *, *, #105810, .T. ) ;
#97919=CARTESIAN_POINT ( 'NONE',  ( -18.19590854888186726, 1522.862737210650039, 180.0410247165186490 ) ) ;
#97928=DIRECTION ( 'NONE',  ( 0.000000000000000000, 0.000000000000000000, 1.000000000000000000 ) ) ;
#97933=FACE_OUTER_BOUND ( 'NONE', #58052, .T. ) ;
#97956=DIRECTION ( 'NONE',  ( 0.000000000000000000, 0.000000000000000000, 1.000000000000000000 ) ) ;
#97968=VERTEX_POINT ( 'NONE', #109105 ) ;
#97973=ORIENTED_EDGE ( 'NONE', *, *, #77539, .F. ) ;
#97977=ADVANCED_FACE ( 'NONE', ( #108535 ), #37095, .T. ) ;
#97988=EDGE_CURVE ( 'NONE', #80761, #6825, #67660, .T. ) ;
#97990=VERTEX_POINT ( 'NONE', #40780 ) ;
#97993=CARTESIAN_POINT ( 'NONE',  ( -29.17014196280706173, 1526.382868172863482, 217.2191814580075970 ) ) ;
#98027=EDGE_CURVE ( 'NONE', #66323, #39930, #15550, .T. ) ;
#98029=CARTESIAN_POINT ( 'NONE',  ( -22.69876404239284184, 1522.861859112240154, 236.8953202675672287 ) ) ;
#98038=CARTESIAN_POINT ( 'NONE',  ( -31.33756689035240584, 1523.580203803270933, 221.9021554055879619 ) ) ;
#98052=EDGE_CURVE ( 'NONE', #42640, #22416, #69245, .T. ) ;
#98057=CARTESIAN_POINT ( 'NONE',  ( 18.19590854888146225, 1522.862737210649811, 180.0410247165184217 ) ) ;
#98058=CARTESIAN_POINT ( 'NONE',  ( -17.84338787552398031, 1523.481610118015169, 237.8836641335898605 ) ) ;
#98064=CARTESIAN_POINT ( 'NONE',  ( 17.83486663330486621, 1523.678648413191695, 180.3677388339000061 ) ) ;
#98068=CARTESIAN_POINT ( 'NONE',  ( 1.191524307911312031, 1526.382868172864164, 179.0083900503168479 ) ) ;
#98069=CARTESIAN_POINT ( 'NONE',  ( -21.84020450222019605, 1523.481610426287716, 234.9798068779743403 ) ) ;
#98099=( BOUNDED_CURVE ( )  B_SPLINE_CURVE ( 3, ( #97284, #105709, #28991, #63178 ),
 .UNSPECIFIED., .F., .F. ) 
 B_SPLINE_CURVE_WITH_KNOTS ( ( 4, 4 ),
 ( 4.712388980384689674, 6.283185307179586232 ),
 .UNSPECIFIED. ) 
 CURVE ( )  GEOMETRIC_REPRESENTATION_ITEM ( )  RATIONAL_B_SPLINE_CURVE ( ( 1.000000000000000000, 0.8047378541243649375, 0.8047378541243649375, 1.000000000000000000 ) ) 
 REPRESENTATION_ITEM ( '' )  );
#98106=CARTESIAN_POINT ( 'NONE',  ( -20.49599333844893678, 1525.960063244516959, 184.3798832129038203 ) ) ;
#98117=CARTESIAN_POINT ( 'NONE',  ( 32.80316127680803362, 1523.919934424249959, 217.1667916731834680 ) ) ;
#98132=EDGE_CURVE ( 'NONE', #61894, #44756, #60450, .T. ) ;
#98144=CARTESIAN_POINT ( 'NONE',  ( -21.41758936356537646, 1524.330813522192102, 184.2067724269699056 ) ) ;
#98151=CARTESIAN_POINT ( 'NONE',  ( -2.038646110889678287, 1525.960063244516959, 241.1857569150893994 ) ) ;
#98153=CIRCLE ( 'NONE', #33721, 1.000000000000005551 ) ;
#98163=CARTESIAN_POINT ( 'NONE',  ( 29.74444329484895988, 1526.348417187218956, 217.2213265034476137 ) ) ;
#98168=DIRECTION ( 'NONE',  ( -0.7414773880254679206, 0.000000000000000000, 0.6709778558543715299 ) ) ;
#98169=ADVANCED_FACE ( 'NONE', ( #9803 ), #94918, .T. ) ;
#98185=CARTESIAN_POINT ( 'NONE',  ( -3.448830483803564828, 1518.913060387330006, 175.1594891075192209 ) ) ;
#98191=PLANE ( 'NONE',  #28700 ) ;
#98196=ADVANCED_FACE ( 'NONE', ( #50706 ), #10351, .T. ) ;
#98203=CARTESIAN_POINT ( 'NONE',  ( -20.53760542139809075, 1525.821544997590081, 184.7213720461156186 ) ) ;
#98213=CARTESIAN_POINT ( 'NONE',  ( -18.66420869458026388, 1526.382868172863937, 232.7837831374280881 ) ) ;
#98216=DIRECTION ( 'NONE',  ( 0.000000000000000000, 1.000000000000000000, 0.000000000000000000 ) ) ;
#98229=AXIS2_PLACEMENT_3D ( 'NONE', #98618, #4576, #83885 ) ;
#98248=CARTESIAN_POINT ( 'NONE',  ( 21.26060865160083679, 1525.055402519434438, 233.8824188859621813 ) ) ;
#98252=CARTESIAN_POINT ( 'NONE',  ( -17.17241001986523941, 1512.187213306747481, 179.6185504016045797 ) ) ;
#98264=EDGE_LOOP ( 'NONE', ( #47, #95826, #49742, #106734 ) ) ;
#98269=CARTESIAN_POINT ( 'NONE',  ( -30.17514886432853061, 1525.712830164893376, 196.9772668248565139 ) ) ;
#98270=VERTEX_POINT ( 'NONE', #83611 ) ;
#98279=CARTESIAN_POINT ( 'NONE',  ( 28.97303002314067655, 1526.186458717542337, 197.4313369063826542 ) ) ;
#98288=ADVANCED_FACE ( 'NONE', ( #81956 ), #47821, .F. ) ;
#98299=DIRECTION ( 'NONE',  ( -0.000000000000000000, -1.000000000000000000, -0.000000000000000000 ) ) ;
#98318=CARTESIAN_POINT ( 'NONE',  ( 2.372478608332517336, 1522.382868172863937, 243.3440112565233449 ) ) ;
#98320=DIRECTION ( 'NONE',  ( 0.9125304618754024322, 0.000000000000000000, -0.4090087482554191078 ) ) ;
#98326=CARTESIAN_POINT ( 'NONE',  ( 2.157496122451417531, 1526.189892541619429, 240.2809797488604033 ) ) ;
#98327=CARTESIAN_POINT ( 'NONE',  ( -2.691662542991861695, 1524.776010967675575, 241.8130992650591224 ) ) ;
#98340=AXIS2_PLACEMENT_3D ( 'NONE', #72769, #78979, #71139 ) ;
#98345=FACE_OUTER_BOUND ( 'NONE', #40981, .T. ) ;
#98381=EDGE_LOOP ( 'NONE', ( #21673, #107810, #68914 ) ) ;
#98388=AXIS2_PLACEMENT_3D ( 'NONE', #26321, #9528, #59413 ) ;
#98405=AXIS2_PLACEMENT_3D ( 'NONE', #70851, #97660, #104961 ) ;
#98414=EDGE_LOOP ( 'NONE', ( #44792, #29271, #108623, #103905, #105180 ) ) ;
#98419=VECTOR ( 'NONE', #45327, 1000.000000000000114 ) ;
#98426=CARTESIAN_POINT ( 'NONE',  ( 32.38114538885250226, 1523.604703353109699, 202.1233279672528624 ) ) ;
#98433=FACE_OUTER_BOUND ( 'NONE', #84521, .T. ) ;
#98435=ADVANCED_FACE ( 'NONE', ( #58988 ), #27036, .F. ) ;
#98457=CARTESIAN_POINT ( 'NONE',  ( -17.84338787571961049, 1523.382868172864164, 180.3600277896300383 ) ) ;
#98469=ORIENTED_EDGE ( 'NONE', *, *, #35983, .T. ) ;
#98471=EDGE_LOOP ( 'NONE', ( #12310, #102861 ) ) ;
#98472=AXIS2_PLACEMENT_3D ( 'NONE', #38184, #28133, #2419 ) ;
#98476=DIRECTION ( 'NONE',  ( 2.775557561562888827E-14, 0.000000000000000000, 1.000000000000000000 ) ) ;
#98487=AXIS2_PLACEMENT_3D ( 'NONE', #41884, #76043, #68222 ) ;
#98489=CARTESIAN_POINT ( 'NONE',  ( 18.10570579381780476, 1525.713797967456458, 238.1210409130211474 ) ) ;
#98492=TOROIDAL_SURFACE ( 'NONE', #21589, 2.000000000000000000, 1.000000000000000000 ) ;
#98493=DIRECTION ( 'NONE',  ( -0.7414773880254664773, 0.000000000000000000, 0.6709778558543730842 ) ) ;
#98509=ORIENTED_EDGE ( 'NONE', *, *, #104907, .F. ) ;
#98519=ADVANCED_FACE ( 'NONE', ( #2964 ), #72361, .T. ) ;
#98534=CARTESIAN_POINT ( 'NONE',  ( 16.53175237173092782, 1526.069472839378477, 235.9420435487000702 ) ) ;
#98545=ORIENTED_EDGE ( 'NONE', *, *, #90507, .T. ) ;
#98555=CARTESIAN_POINT ( 'NONE',  ( 29.70307219812704247, 1525.408337840049853, 196.2982874201323114 ) ) ;
#98561=ORIENTED_EDGE ( 'NONE', *, *, #106857, .T. ) ;
#98584=CARTESIAN_POINT ( 'NONE',  ( 0.4151546846821903003, 1522.382868172863937, 242.9330574173806951 ) ) ;
#98607=EDGE_CURVE ( 'NONE', #13899, #67344, #58608, .T. ) ;
#98617=CARTESIAN_POINT ( 'NONE',  ( 16.73628186595824019, 1526.382868172863937, 184.0591879540915272 ) ) ;
#98618=CARTESIAN_POINT ( 'NONE',  ( 0.000000000000000000, 1526.382868172863937, 209.1218459616979999 ) ) ;
#98639=CARTESIAN_POINT ( 'NONE',  ( 33.28034951413924603, 1512.187213306747481, 200.8029765415137433 ) ) ;
#98650=CARTESIAN_POINT ( 'NONE',  ( -49.24962907673571522, 1524.382868172863937, 10.34030387146701813 ) ) ;
#98656=CIRCLE ( 'NONE', #102247, 1.000000000000005551 ) ;
#98669=ORIENTED_EDGE ( 'NONE', *, *, #44798, .T. ) ;
#98676=AXIS2_PLACEMENT_3D ( 'NONE', #32349, #66528, #33992 ) ;
#98702=CARTESIAN_POINT ( 'NONE',  ( -21.33281718256877824, 1523.429859730331145, 180.4846393450511641 ) ) ;
#98706=EDGE_CURVE ( 'NONE', #94134, #30502, #42043, .T. ) ;
#98712=FACE_OUTER_BOUND ( 'NONE', #16230, .T. ) ;
#98714=ORIENTED_EDGE ( 'NONE', *, *, #76957, .F. ) ;
#98716=DIRECTION ( 'NONE',  ( 0.000000000000000000, 1.000000000000000000, 0.000000000000000000 ) ) ;
#98721=CARTESIAN_POINT ( 'NONE',  ( 16.50400130224746675, 1525.907212628473644, 181.9890130758377609 ) ) ;
#98726=ORIENTED_EDGE ( 'NONE', *, *, #47009, .T. ) ;
#98735=AXIS2_PLACEMENT_3D ( 'NONE', #60337, #51365, #42980 ) ;
#98738=CYLINDRICAL_SURFACE ( 'NONE', #80702, 1.000000000000000888 ) ;
#98743=ADVANCED_FACE ( 'NONE', ( #88994 ), #65758, .F. ) ;
#98747=LINE ( 'NONE', #47255, #38993 ) ;
#98751=DIRECTION ( 'NONE',  ( -0.000000000000000000, -1.000000000000000000, -0.000000000000000000 ) ) ;
#98752=CIRCLE ( 'NONE', #52265, 1.000000000000000888 ) ;
#98755=CARTESIAN_POINT ( 'NONE',  ( 31.31962774233649682, 1525.556090473913628, 216.7000093993642906 ) ) ;
#98801=VERTEX_POINT ( 'NONE', #67424 ) ;
#98806=CARTESIAN_POINT ( 'NONE',  ( -28.62766089293194227, 1526.344110814219903, 198.0439708942000721 ) ) ;
#98816=ORIENTED_EDGE ( 'NONE', *, *, #94906, .T. ) ;
#98839=CARTESIAN_POINT ( 'NONE',  ( 17.78793234590488481, 1523.919934424249959, 180.4102106179817042 ) ) ;
#98852=CARTESIAN_POINT ( 'NONE',  ( -3.350338079455601026, 1523.604703353109699, 176.1628856388066708 ) ) ;
#98871=VERTEX_POINT ( 'NONE', #35451 ) ;
#98891=VERTEX_POINT ( 'NONE', #1879 ) ;
#98916=CARTESIAN_POINT ( 'NONE',  ( 29.79881796581619469, 1526.748660780343698, 221.5803863269301246 ) ) ;
#98917=EDGE_CURVE ( 'NONE', #64661, #2574, #9690, .T. ) ;
#98918=FACE_OUTER_BOUND ( 'NONE', #34507, .T. ) ;
#98938=CARTESIAN_POINT ( 'NONE',  ( 20.71343476517512272, 1512.187213306747481, 179.9059455038194528 ) ) ;
#98946=CIRCLE ( 'NONE', #79310, 2.000000000000001776 ) ;
#98969=DIRECTION ( 'NONE',  ( -0.9942586961433752535, 0.000000000000000000, 0.1070030146457353060 ) ) ;
#98988=CARTESIAN_POINT ( 'NONE',  ( -32.38114538885259464, 1523.604703353109699, 202.1233279672532888 ) ) ;
#98990=ORIENTED_EDGE ( 'NONE', *, *, #60466, .F. ) ;
#99009=CARTESIAN_POINT ( 'NONE',  ( -31.31962989722713786, 1525.556089352344770, 216.7000087461251212 ) ) ;
#99018=B_SPLINE_CURVE_WITH_KNOTS ( 'NONE', 3,
 ( #27254, #28358, #1516, #972, #62556, #35649, #103384, #77659, #18281, #35097, #19948, #52475 ),
 .UNSPECIFIED., .F., .F.,
 ( 4, 2, 2, 2, 2, 4 ),
 ( 0.000000000000000000, 0.0007194225121792270335, 0.001079133768269161528, 0.001438845024359096348, 0.002158267536538997864, 0.002877690048718900030 ),
 .UNSPECIFIED. ) ;
#99027=CIRCLE ( 'NONE', #72293, 1.000000000000000888 ) ;
#99078=( BOUNDED_CURVE ( )  B_SPLINE_CURVE ( 3, ( #82916, #73982, #99701, #40359 ),
 .UNSPECIFIED., .F., .F. ) 
 B_SPLINE_CURVE_WITH_KNOTS ( ( 4, 4 ),
 ( 2.436781329611982017, 3.141592653589793116 ),
 .UNSPECIFIED. ) 
 CURVE ( )  GEOMETRIC_REPRESENTATION_ITEM ( )  RATIONAL_B_SPLINE_CURVE ( ( 1.000000000000000000, 0.9590300661663084814, 0.9590300661663084814, 1.000000000000000000 ) ) 
 REPRESENTATION_ITEM ( '' )  );
#99085=ORIENTED_EDGE ( 'NONE', *, *, #34595, .F. ) ;
#99094=VECTOR ( 'NONE', #73896, 1000.000000000000000 ) ;
#99110=ORIENTED_EDGE ( 'NONE', *, *, #63930, .F. ) ;
#99120=CARTESIAN_POINT ( 'NONE',  ( -31.55060375016910257, 1525.712835404586031, 201.2105082957782543 ) ) ;
#99121=CYLINDRICAL_SURFACE ( 'NONE', #52063, 4.000000000000003553 ) ;
#99125=CARTESIAN_POINT ( 'NONE',  ( 21.54890432409654011, 1524.816846803860471, 183.6629423615462429 ) ) ;
#99127=FACE_OUTER_BOUND ( 'NONE', #43687, .T. ) ;
#99140=CARTESIAN_POINT ( 'NONE',  ( -16.92737834736502833, 1525.317349363549965, 181.4495812669162831 ) ) ;
#99145=DIRECTION ( 'NONE',  ( 0.000000000000000000, 1.000000000000000000, 0.000000000000000000 ) ) ;
#99147=CARTESIAN_POINT ( 'NONE',  ( -17.29882006758053592, 1523.542365884048650, 237.3908737315615269 ) ) ;
#99178=VECTOR ( 'NONE', #81214, 1000.000000000000000 ) ;
#99179=CARTESIAN_POINT ( 'NONE',  ( -32.38114538885245963, 1523.604703353109699, 216.1203639561433647 ) ) ;
#99183=ORIENTED_EDGE ( 'NONE', *, *, #83786, .T. ) ;
#99203=EDGE_LOOP ( 'NONE', ( #57494, #50721, #86523, #75015 ) ) ;
#99209=CARTESIAN_POINT ( 'NONE',  ( -3.347801439296148818, 1523.382868172864164, 242.0893193391992497 ) ) ;
#99219=ORIENTED_EDGE ( 'NONE', *, *, #80073, .T. ) ;
#99223=CARTESIAN_POINT ( 'NONE',  ( -17.22845782853304542, 1525.848196786131211, 181.7617168241399952 ) ) ;
#99231=CARTESIAN_POINT ( 'NONE',  ( -22.14913372576182127, 1525.402221411349728, 182.5746398196750988 ) ) ;
#99247=CARTESIAN_POINT ( 'NONE',  ( -2.390047989678332208, 1526.069472839386663, 177.7067300826772964 ) ) ;
#99262=FACE_OUTER_BOUND ( 'NONE', #21653, .T. ) ;
#99288=CARTESIAN_POINT ( 'NONE',  ( -20.49599333844887639, 1525.960063244516959, 184.3798832129037351 ) ) ;
#99294=CARTESIAN_POINT ( 'NONE',  ( 31.81407709660769001, 1522.382868172863937, 196.2902540610627682 ) ) ;
#99302=CARTESIAN_POINT ( 'NONE',  ( 16.52275002910640112, 1525.042412244750039, 237.2696364103756252 ) ) ;
#99303=ADVANCED_FACE ( 'NONE', ( #94518 ), #77200, .F. ) ;
#99309=CARTESIAN_POINT ( 'NONE',  ( -18.19590854888185305, 1512.187213306747481, 180.0410247165186490 ) ) ;
#99332=ORIENTED_EDGE ( 'NONE', *, *, #48004, .T. ) ;
#99336=ORIENTED_EDGE ( 'NONE', *, *, #70910, .T. ) ;
#99337=FACE_OUTER_BOUND ( 'NONE', #18474, .T. ) ;
#99350=ORIENTED_EDGE ( 'NONE', *, *, #50862, .F. ) ;
#99369=DIRECTION ( 'NONE',  ( 0.7414773880254711402, 0.000000000000000000, 0.6709778558543678662 ) ) ;
#99388=CARTESIAN_POINT ( 'NONE',  ( -173.8335085727391913, 1524.382868172863937, 317.3879012941878273 ) ) ;
#99389=CARTESIAN_POINT ( 'NONE',  ( -0.4151546846821903003, 1511.187213306747708, 242.9330574173806951 ) ) ;
#99395=ADVANCED_FACE ( 'NONE', ( #36281 ), #104592, .T. ) ;
#99429=CARTESIAN_POINT ( 'NONE',  ( -16.53242905777631222, 1526.073429442291854, 235.9344201561504804 ) ) ;
#99433=CARTESIAN_POINT ( 'NONE',  ( -19.38211899475871647, 1526.344110814221267, 232.9251177427894390 ) ) ;
#99442=FACE_OUTER_BOUND ( 'NONE', #31322, .T. ) ;
#99467=VERTEX_POINT ( 'NONE', #84820 ) ;
#99506=EDGE_CURVE ( 'NONE', #23328, #22416, #21002, .T. ) ;
#99513=CARTESIAN_POINT ( 'NONE',  ( 33.23571934791672788, 1512.187213306747481, 219.4842663281462478 ) ) ;
#99537=ORIENTED_EDGE ( 'NONE', *, *, #7129, .T. ) ;
#99562=ORIENTED_EDGE ( 'NONE', *, *, #26080, .T. ) ;
#99573=FACE_OUTER_BOUND ( 'NONE', #106795, .T. ) ;
#99575=DIRECTION ( 'NONE',  ( 0.000000000000000000, 1.000000000000000000, 0.000000000000000000 ) ) ;
#99576=FACE_OUTER_BOUND ( 'NONE', #46398, .T. ) ;
#99577=TOROIDAL_SURFACE ( 'NONE', #79946, 32.13701971169416538, 1.000000000000000000 ) ;
#99581=CARTESIAN_POINT ( 'NONE',  ( 18.19590854887586318, 1522.644714754857659, 238.2026672068722064 ) ) ;
#99584=DIRECTION ( 'NONE',  ( -0.000000000000000000, -1.000000000000000000, -0.000000000000000000 ) ) ;
#99595=AXIS2_PLACEMENT_3D ( 'NONE', #2614, #106687, #63627 ) ;
#99596=CARTESIAN_POINT ( 'NONE',  ( 29.33952678944442027, 1526.382868172864164, 201.1028049641010114 ) ) ;
#99611=DIRECTION ( 'NONE',  ( 0.000000000000000000, 1.000000000000000000, 0.000000000000000000 ) ) ;
#99620=VECTOR ( 'NONE', #106298, 1000.000000000000000 ) ;
#99653=AXIS2_PLACEMENT_3D ( 'NONE', #72901, #108692, #90225 ) ;
#99660=DIRECTION ( 'NONE',  ( 0.000000000000000000, 1.000000000000000000, 0.000000000000000000 ) ) ;
#99665=CARTESIAN_POINT ( 'NONE',  ( 32.37018134260397062, 1511.187213306747708, 200.1723992780595438 ) ) ;
#99671=FACE_OUTER_BOUND ( 'NONE', #11758, .T. ) ;
#99675=CARTESIAN_POINT ( 'NONE',  ( 21.76694865736958562, 1524.152444737676205, 183.4045613090604832 ) ) ;
#99679=DIRECTION ( 'NONE',  ( 0.6709778558543718630, 0.000000000000000000, -0.7414773880254675875 ) ) ;
#99684=DIRECTION ( 'NONE',  ( 0.000000000000000000, 1.000000000000000000, 0.000000000000000000 ) ) ;
#99691=CARTESIAN_POINT ( 'NONE',  ( -17.12660205615338427, 1524.374578187333100, 180.9416429095477099 ) ) ;
#99699=CARTESIAN_POINT ( 'NONE',  ( -17.29393938232439965, 1523.621879633028811, 237.3864571009502242 ) ) ;
#99701=CARTESIAN_POINT ( 'NONE',  ( -22.03465957474588066, 1522.862737210650039, 182.8300405912331428 ) ) ;
#99705=ORIENTED_EDGE ( 'NONE', *, *, #11077, .T. ) ;
#99708=CARTESIAN_POINT ( 'NONE',  ( -21.83550407203883736, 1523.678648413191695, 234.9693198511253627 ) ) ;
#99709=ORIENTED_EDGE ( 'NONE', *, *, #65857, .T. ) ;
#99737=EDGE_LOOP ( 'NONE', ( #16980, #82417, #66704, #94654 ) ) ;
#99756=ORIENTED_EDGE ( 'NONE', *, *, #36336, .F. ) ;
#99759=CARTESIAN_POINT ( 'NONE',  ( 18.07041998555298434, 1523.313115944345327, 238.0891100728146625 ) ) ;
#99787=CARTESIAN_POINT ( 'NONE',  ( -21.13130013988163114, 1524.397344074317971, 180.8335768739890455 ) ) ;
#99791=CIRCLE ( 'NONE', #51526, 2.000000000000001776 ) ;
#99793=ORIENTED_EDGE ( 'NONE', *, *, #104995, .T. ) ;
#99808=CARTESIAN_POINT ( 'NONE',  ( 16.85976061912560908, 1525.821544997590536, 182.0492613858611719 ) ) ;
#99814=ORIENTED_EDGE ( 'NONE', *, *, #71695, .F. ) ;
#99821=EDGE_CURVE ( 'NONE', #7253, #23788, #90879, .T. ) ;
#99823=DIRECTION ( 'NONE',  ( 0.000000000000000000, 0.000000000000000000, 1.000000000000000000 ) ) ;
#99825=TOROIDAL_SURFACE ( 'NONE', #37270, 32.13701971169416538, 1.000000000000000000 ) ;
#99840=CARTESIAN_POINT ( 'NONE',  ( 1.484142863822459857, 1526.349689584397083, 239.9035297921357142 ) ) ;
#99845=DIRECTION ( 'NONE',  ( -0.000000000000000000, -1.000000000000000000, -0.000000000000000000 ) ) ;
#99867=ORIENTED_EDGE ( 'NONE', *, *, #35083, .T. ) ;
#99880=SURFACE_STYLE_USAGE ( .BOTH. , #66333 ) ;
#99893=CIRCLE ( 'NONE', #33716, 32.13701971169416538 ) ;
#99903=EDGE_CURVE ( 'NONE', #97183, #81284, #98747, .T. ) ;
#99923=CARTESIAN_POINT ( 'NONE',  ( 29.36670733768142227, 1526.000688113686692, 197.3383209345576006 ) ) ;
#99929=DIRECTION ( 'NONE',  ( -0.9942586961433742543, 0.000000000000000000, 0.1070030146457445069 ) ) ;
#99939=LINE ( 'NONE', #40046, #9795 ) ;
#99945=CARTESIAN_POINT ( 'NONE',  ( -3.347801439296141712, 1523.382868172864164, 176.1543725841967500 ) ) ;
#99949=FACE_OUTER_BOUND ( 'NONE', #64107, .T. ) ;
#99959=AXIS2_PLACEMENT_3D ( 'NONE', #17672, #77076, #33382 ) ;
#99967=CARTESIAN_POINT ( 'NONE',  ( 0.000000000000000000, 1512.187213306747481, 209.1218459616979999 ) ) ;
#99969=CARTESIAN_POINT ( 'NONE',  ( 32.39779788405888894, 1524.816846803860926, 201.1912884557872303 ) ) ;
#99976=CIRCLE ( 'NONE', #41000, 30.13701971169416183 ) ;
#99987=EDGE_LOOP ( 'NONE', ( #72267, #69744, #90668, #30883 ) ) ;
#99990=CARTESIAN_POINT ( 'NONE',  ( -20.21716934224603079, 1526.104292489135332, 233.6939662645372380 ) ) ;
#100008=ORIENTED_EDGE ( 'NONE', *, *, #58396, .T. ) ;
#100023=ORIENTED_EDGE ( 'NONE', *, *, #33566, .F. ) ;
#100026=EDGE_LOOP ( 'NONE', ( #81839, #64530, #61072 ) ) ;
#100035=CIRCLE ( 'NONE', #3523, 2.000000000000003553 ) ;
#100043=VECTOR ( 'NONE', #96694, 1000.000000000000000 ) ;
#100050=CIRCLE ( 'NONE', #12464, 0.9999999999999935607 ) ;
#100071=CARTESIAN_POINT ( 'NONE',  ( 19.53786426059039982, 1512.187213306747481, 236.7197124308265188 ) ) ;
#100079=ADVANCED_FACE ( 'NONE', ( #82887 ), #40837, .T. ) ;
#100089=CARTESIAN_POINT ( 'NONE',  ( -22.69876404240119072, 1501.977400791986611, 181.3483716558183119 ) ) ;
#100110=VERTEX_POINT ( 'NONE', #87309 ) ;
#100114=LINE ( 'NONE', #100648, #54567 ) ;
#100119=DIRECTION ( 'NONE',  ( 0.9125304618753903307, 0.000000000000000000, -0.4090087482554460863 ) ) ;
#100125=ORIENTED_EDGE ( 'NONE', *, *, #106394, .T. ) ;
#100126=CARTESIAN_POINT ( 'NONE',  ( 33.72300830903717639, 1524.397344074318198, 219.5868698111207777 ) ) ;
#100135=CARTESIAN_POINT ( 'NONE',  ( 2.470168521978402421, 1523.481610426287716, 175.3649660270905599 ) ) ;
#100146=AXIS2_PLACEMENT_3D ( 'NONE', #30178, #14481, #98493 ) ;
#100159=LINE ( 'NONE', #49775, #62665 ) ;
#100166=FACE_OUTER_BOUND ( 'NONE', #16596, .T. ) ;
#100176=TOROIDAL_SURFACE ( 'NONE', #89398, 1.000000000000000000, 1.000000000000000000 ) ;
#100179=EDGE_CURVE ( 'NONE', #20284, #102300, #80906, .T. ) ;
#100184=DIRECTION ( 'NONE',  ( 0.4090087482554316534, -0.000000000000000000, 0.9125304618753967700 ) ) ;
#100188=VERTEX_POINT ( 'NONE', #89505 ) ;
#100236=CARTESIAN_POINT ( 'NONE',  ( 16.50400130224771544, 1525.907212628473644, 236.2546788475581820 ) ) ;
#100238=PLANE ( 'NONE',  #93295 ) ;
#100252=CARTESIAN_POINT ( 'NONE',  ( 21.63718167644599433, 1524.600389084706649, 183.5694068101082621 ) ) ;
#100259=EDGE_LOOP ( 'NONE', ( #68761, #18111, #103064, #90260 ) ) ;
#100262=B_SPLINE_CURVE_WITH_KNOTS ( 'NONE', 3,
 ( #81149, #38056, #56521, #31299, #72234, #30747, #80612, #81688, #108002, #90648, #21211, #38592 ),
 .UNSPECIFIED., .F., .F.,
 ( 4, 2, 2, 2, 2, 4 ),
 ( 0.000000000000000000, 0.0007194225121803531943, 0.001079133768270215156, 0.001438845024360077118, 0.002158267536539286262, 0.002877690048718495406 ),
 .UNSPECIFIED. ) ;
#100268=CARTESIAN_POINT ( 'NONE',  ( -17.42134197181179545, 1525.253996226947947, 181.0775359434758229 ) ) ;
#100274=DIRECTION ( 'NONE',  ( 4.440892098500626162E-15, 0.000000000000000000, 1.000000000000000000 ) ) ;
#100276=CARTESIAN_POINT ( 'NONE',  ( 32.38845791999494850, 1523.456872492435195, 202.1182848005511801 ) ) ;
#100278=CARTESIAN_POINT ( 'NONE',  ( -20.37381179411450560, 1524.397344074318880, 237.9604625470747123 ) ) ;
#100291=DIRECTION ( 'NONE',  ( -1.000000000000000000, 0.000000000000000000, 0.000000000000000000 ) ) ;
#100304=VERTEX_POINT ( 'NONE', #20622 ) ;
#100321=VERTEX_POINT ( 'NONE', #94888 ) ;
#100328=CIRCLE ( 'NONE', #87879, 33.13701971169416538 ) ;
#100334=ADVANCED_FACE ( 'NONE', ( #52905 ), #108511, .T. ) ;
#100336=CARTESIAN_POINT ( 'NONE',  ( 29.99674465255694500, 1524.860077346005028, 222.2674750195774322 ) ) ;
#100363=DIRECTION ( 'NONE',  ( -0.000000000000000000, -1.000000000000000000, -0.000000000000000000 ) ) ;
#100368=EDGE_CURVE ( 'NONE', #47286, #79230, #47964, .T. ) ;
#100391=AXIS2_PLACEMENT_3D ( 'NONE', #42494, #91245, #50371 ) ;
#100392=CARTESIAN_POINT ( 'NONE',  ( -29.99620953741480278, 1526.382868172863937, 219.7462484079463252 ) ) ;
#100399=DIRECTION ( 'NONE',  ( -3.469446951953611033E-15, 0.000000000000000000, 1.000000000000000000 ) ) ;
#100410=CARTESIAN_POINT ( 'NONE',  ( 31.30542346655888863, 1525.651286436460396, 216.2805831001146259 ) ) ;
#100420=CARTESIAN_POINT ( 'NONE',  ( 21.05711716160284652, 1526.748660780343698, 184.6313866553783498 ) ) ;
#100424=CARTESIAN_POINT ( 'NONE',  ( 17.50735355147223160, 1524.972613296789177, 237.3782595154142996 ) ) ;
#100483=VECTOR ( 'NONE', #7618, 999.9999999999998863 ) ;
#100491=CARTESIAN_POINT ( 'NONE',  ( -21.91520783698913633, 1524.538768545233779, 233.6709662800621459 ) ) ;
#100497=CIRCLE ( 'NONE', #104014, 1.000000000000000000 ) ;
#100499=DIRECTION ( 'NONE',  ( -0.9942586961433764747, 0.000000000000000000, -0.1070030146457237041 ) ) ;
#100508=CARTESIAN_POINT ( 'NONE',  ( 29.78220350812350858, 1524.382868172863937, 221.7347658002326227 ) ) ;
#100526=ORIENTED_EDGE ( 'NONE', *, *, #43179, .T. ) ;
#100536=CARTESIAN_POINT ( 'NONE',  ( -33.93019615848960768, 1522.382868172863937, 197.6607374646001176 ) ) ;
#100554=CARTESIAN_POINT ( 'NONE',  ( -2.314969334973923765, 1525.402221411349728, 243.6179210388351066 ) ) ;
#100566=LINE ( 'NONE', #56936, #30115 ) ;
#100569=CARTESIAN_POINT ( 'NONE',  ( 2.038646110889569485, 1525.960063244516959, 241.1857569150894278 ) ) ;
#100587=VERTEX_POINT ( 'NONE', #64068 ) ;
#100594=CARTESIAN_POINT ( 'NONE',  ( 33.35590117750194139, 1523.678648413191695, 201.9126545693500816 ) ) ;
#100596=CARTESIAN_POINT ( 'NONE',  ( 20.91563430996840012, 1525.795403621570813, 184.9927170714047691 ) ) ;
#100597=VERTEX_POINT ( 'NONE', #10324 ) ;
#100600=CARTESIAN_POINT ( 'NONE',  ( -29.13898522073073494, 1526.069472839383479, 221.1027213634203576 ) ) ;
#100609=VERTEX_POINT ( 'NONE', #105504 ) ;
#100614=CARTESIAN_POINT ( 'NONE',  ( -17.84054676580398180, 1523.580203803270933, 237.8810931560536801 ) ) ;
#100644=VERTEX_POINT ( 'NONE', #106053 ) ;
#100648=CARTESIAN_POINT ( 'NONE',  ( 32.97913964219439720, 1511.187213306747708, 220.2739374644211807 ) ) ;
#100652=CARTESIAN_POINT ( 'NONE',  ( 19.39983987835127976, 1522.861859112239699, 178.9515629539953636 ) ) ;
#100654=EDGE_CURVE ( 'NONE', #105727, #47062, #71265, .T. ) ;
#100672=CARTESIAN_POINT ( 'NONE',  ( -31.81407709660760830, 1501.977400791986611, 221.9534378623334590 ) ) ;
#100673=DIRECTION ( 'NONE',  ( 0.000000000000000000, 1.000000000000000000, 0.000000000000000000 ) ) ;
#100677=CARTESIAN_POINT ( 'NONE',  ( -21.83863729848776458, 1523.580204110582372, 234.9763103240451301 ) ) ;
#100686=CARTESIAN_POINT ( 'NONE',  ( -21.92333112166566167, 1524.538969332612623, 184.5696470164554341 ) ) ;
#100694=EDGE_CURVE ( 'NONE', #53518, #83932, #42148, .T. ) ;
#100715=FACE_OUTER_BOUND ( 'NONE', #90527, .T. ) ;
#100720=ORIENTED_EDGE ( 'NONE', *, *, #37738, .F. ) ;
#100724=CARTESIAN_POINT ( 'NONE',  ( -31.44837959398574867, 1512.187213306747481, 220.9083067115980725 ) ) ;
#100730=EDGE_CURVE ( 'NONE', #95247, #47770, #30077, .T. ) ;
#100733=ORIENTED_EDGE ( 'NONE', *, *, #96661, .F. ) ;
#100747=CARTESIAN_POINT ( 'NONE',  ( 33.28034951413933129, 1512.187213306747481, 217.4407153818819722 ) ) ;
#100752=ORIENTED_EDGE ( 'NONE', *, *, #22937, .T. ) ;
#100761=ADVANCED_FACE ( 'NONE', ( #62286 ), #97510, .T. ) ;
#100779=CARTESIAN_POINT ( 'NONE',  ( -2.038847259681869417, 1522.861859112239017, 173.3106345060298281 ) ) ;
#100785=ORIENTED_EDGE ( 'NONE', *, *, #46715, .F. ) ;
#100788=EDGE_CURVE ( 'NONE', #70084, #75960, #19122, .T. ) ;
#100789=DIRECTION ( 'NONE',  ( 0.000000000000000000, 0.000000000000000000, -1.000000000000000000 ) ) ;
#100796=CARTESIAN_POINT ( 'NONE',  ( 3.350338079455597029, 1523.604703353109699, 176.1628856388066708 ) ) ;
#100799=CIRCLE ( 'NONE', #7854, 1.000000000000000888 ) ;
#100809=CARTESIAN_POINT ( 'NONE',  ( 204.2714532754872323, 1526.382868172863937, 194.5341519463041777 ) ) ;
#100830=EDGE_CURVE ( 'NONE', #10931, #21131, #29743, .T. ) ;
#100834=ORIENTED_EDGE ( 'NONE', *, *, #52202, .F. ) ;
#100847=( BOUNDED_CURVE ( )  B_SPLINE_CURVE ( 3, ( #72679, #47474, #46939, #4901 ),
 .UNSPECIFIED., .F., .T. ) 
 B_SPLINE_CURVE_WITH_KNOTS ( ( 4, 4 ),
 ( 0.000000000000000000, 0.7048113239778087680 ),
 .UNSPECIFIED. ) 
 CURVE ( )  GEOMETRIC_REPRESENTATION_ITEM ( )  RATIONAL_B_SPLINE_CURVE ( ( 1.000000000000000000, 0.9590300661663088144, 0.9590300661663088144, 1.000000000000000000 ) ) 
 REPRESENTATION_ITEM ( '' )  );
#100849=CYLINDRICAL_SURFACE ( 'NONE', #56126, 1.000000000000000888 ) ;
#100852=CARTESIAN_POINT ( 'NONE',  ( 18.02257621027597523, 1526.382868172863937, 235.3484976865586873 ) ) ;
#100855=AXIS2_PLACEMENT_3D ( 'NONE', #92879, #81710, #73338 ) ;
#100891=CARTESIAN_POINT ( 'NONE',  ( -21.50855465201878403, 1524.374578187332872, 234.1183740972438159 ) ) ;
#100901=CARTESIAN_POINT ( 'NONE',  ( 0.000000000000000000, 1523.409940573003951, 209.1218459616979999 ) ) ;
#100931=CARTESIAN_POINT ( 'NONE',  ( 21.80961449745507963, 1523.919934424249959, 234.9115581881929415 ) ) ;
#100932=B_SPLINE_CURVE_WITH_KNOTS ( 'NONE', 3,
 ( #21338, #89668, #23960, #32925, #49755, #75515 ),
 .UNSPECIFIED., .F., .F.,
 ( 4, 2, 4 ),
 ( 1.040834085586084257E-17, 0.001087661325621706431, 0.002175322651243402454 ),
 .UNSPECIFIED. ) ;
#100946=DIRECTION ( 'NONE',  ( 0.9510565162951566398, 0.000000000000000000, 0.3090169943749382919 ) ) ;
#100959=CARTESIAN_POINT ( 'NONE',  ( 17.26794000855596423, 1525.730671215505254, 236.6572858183501751 ) ) ;
#100969=EDGE_CURVE ( 'NONE', #81049, #104688, #51560, .T. ) ;
#100983=EDGE_CURVE ( 'NONE', #22899, #15596, #10394, .T. ) ;
#100986=CARTESIAN_POINT ( 'NONE',  ( -20.20959865099451847, 1512.187213306747481, 236.2316688286741453 ) ) ;
#100987=( NAMED_UNIT ( * ) SI_UNIT ( $, .STERADIAN. ) SOLID_ANGLE_UNIT ( ) );
#100995=ORIENTED_EDGE ( 'NONE', *, *, #55740, .F. ) ;
#101003=CARTESIAN_POINT ( 'NONE',  ( 0.4151546846821903003, 1501.977400791986611, 173.3106345060153046 ) ) ;
#101011=DIRECTION ( 'NONE',  ( 0.8672669759446595128, 0.000000000000000000, -0.4978433412588795237 ) ) ;
#101018=CARTESIAN_POINT ( 'NONE',  ( 0.000000000000000000, 1512.187213306747481, 209.1218459616979999 ) ) ;
#101020=CIRCLE ( 'NONE', #33086, 2.000000000000000444 ) ;
#101042=CARTESIAN_POINT ( 'NONE',  ( 17.17241001986506177, 1523.382868172864164, 238.6251415217915053 ) ) ;
#101043=CARTESIAN_POINT ( 'NONE',  ( 31.02592223166964658, 1526.278758871496620, 219.9652544506485015 ) ) ;
#101059=EDGE_CURVE ( 'NONE', #47770, #71731, #110309, .T. ) ;
#101062=TOROIDAL_SURFACE ( 'NONE', #74252, 1.000000000000000000, 1.000000000000000000 ) ;
#101064=ORIENTED_EDGE ( 'NONE', *, *, #22830, .F. ) ;
#101069=CARTESIAN_POINT ( 'NONE',  ( 16.16632277704800558, 1512.187213306747481, 236.8966194768523508 ) ) ;
#101080=DIRECTION ( 'NONE',  ( -1.040834085586083310E-14, 0.000000000000000000, 1.000000000000000000 ) ) ;
#101085=CARTESIAN_POINT ( 'NONE',  ( -20.28160989816897697, 1526.000688113710567, 233.4099348502813314 ) ) ;
#101124=DIRECTION ( 'NONE',  ( -1.000000000000000000, 0.000000000000000000, 0.000000000000000000 ) ) ;
#101129=DIRECTION ( 'NONE',  ( -0.9125304618754024322, 0.000000000000000000, -0.4090087482554191078 ) ) ;
#101136=DIRECTION ( 'NONE',  ( -0.000000000000000000, -1.000000000000000000, -0.000000000000000000 ) ) ;
#101153=DIRECTION ( 'NONE',  ( 0.000000000000000000, 1.000000000000000000, 0.000000000000000000 ) ) ;
#101157=CARTESIAN_POINT ( 'NONE',  ( -17.84338787571901364, 1523.382868172864164, 237.8836641337663309 ) ) ;
#101173=AXIS2_PLACEMENT_3D ( 'NONE', #92208, #108463, #66492 ) ;
#101174=AXIS2_PLACEMENT_3D ( 'NONE', #14946, #58637, #92770 ) ;
#101203=ORIENTED_EDGE ( 'NONE', *, *, #105133, .T. ) ;
#101207=VERTEX_POINT ( 'NONE', #75078 ) ;
#101245=CARTESIAN_POINT ( 'NONE',  ( -2.596261494520144986, 1525.907212628473872, 177.4701144822249148 ) ) ;
#101252=VERTEX_POINT ( 'NONE', #109228 ) ;
#101256=ORIENTED_EDGE ( 'NONE', *, *, #9770, .T. ) ;
#101260=VERTEX_POINT ( 'NONE', #109764 ) ;
#101280=EDGE_CURVE ( 'NONE', #89888, #14943, #41542, .T. ) ;
#101295=CARTESIAN_POINT ( 'NONE',  ( 32.20549126534967854, 1524.425415513989037, 202.1446967539542641 ) ) ;
#101299=ADVANCED_FACE ( 'NONE', ( #89399 ), #28307, .T. ) ;
#101321=CARTESIAN_POINT ( 'NONE',  ( -2.057041824809803465, 1523.342713519622976, 173.3972930408659749 ) ) ;
#101333=CARTESIAN_POINT ( 'NONE',  ( -17.72016947434968159, 1524.201816949777822, 180.4881000152817876 ) ) ;
#101334=CARTESIAN_POINT ( 'NONE',  ( 3.347801439296140380, 1523.382868172864164, 176.1543725841967216 ) ) ;
#101336=DIRECTION ( 'NONE',  ( 0.9977304882603014180, 0.06733403890946067227, 0.000000000000000000 ) ) ;
#101338=LINE ( 'NONE', #16236, #76799 ) ;
#101341=CARTESIAN_POINT ( 'NONE',  ( -16.66936639845670243, 1512.187213306747481, 180.4828114240741854 ) ) ;
#101344=CARTESIAN_POINT ( 'NONE',  ( -20.64339891394538284, 1523.429859730330236, 238.2599442700839063 ) ) ;
#101355=CARTESIAN_POINT ( 'NONE',  ( 16.78480385485693560, 1526.748660780343471, 236.7163225783321820 ) ) ;
#101363=CARTESIAN_POINT ( 'NONE',  ( -29.35747451428025556, 1526.382868172571307, 217.1997937176765276 ) ) ;
#101366=VECTOR ( 'NONE', #21268, 1000.000000000000000 ) ;
#101368=EDGE_CURVE ( 'NONE', #91018, #58921, #96977, .T. ) ;
#101392=ORIENTED_EDGE ( 'NONE', *, *, #36371, .T. ) ;
#101393=AXIS2_PLACEMENT_3D ( 'NONE', #5788, #81361, #90873 ) ;
#101399=ADVANCED_FACE ( 'NONE', ( #8409 ), #55259, .T. ) ;
#101400=DIRECTION ( 'NONE',  ( 0.5877852522924673639, 0.000000000000000000, -0.8090169943749514481 ) ) ;
#101402=CARTESIAN_POINT ( 'NONE',  ( -3.350338079455597029, 1523.604703353109699, 242.0808062845893289 ) ) ;
#101442=ORIENTED_EDGE ( 'NONE', *, *, #37764, .F. ) ;
#101458=ADVANCED_FACE ( 'NONE', ( #4977 ), #67717, .T. ) ;
#101461=EDGE_CURVE ( 'NONE', #47496, #36172, #110620, .T. ) ;
#101475=AXIS2_PLACEMENT_3D ( 'NONE', #88409, #72722, #106844 ) ;
#101479=CARTESIAN_POINT ( 'NONE',  ( -31.00891611928356895, 1524.547873515804895, 196.4334223138416462 ) ) ;
#101492=CARTESIAN_POINT ( 'NONE',  ( -17.17241001986462123, 1512.187213306747481, 238.6251415217917895 ) ) ;
#101496=CARTESIAN_POINT ( 'NONE',  ( 17.78112816951787067, 1523.954914175594240, 180.4163678545431537 ) ) ;
#101499=DIRECTION ( 'NONE',  ( -0.000000000000000000, -1.000000000000000000, -0.000000000000000000 ) ) ;
#101502=CARTESIAN_POINT ( 'NONE',  ( 16.62424264452790723, 1524.075132568164463, 237.7045363987409701 ) ) ;
#101507=LINE ( 'NONE', #52663, #44655 ) ;
#101534=EDGE_LOOP ( 'NONE', ( #21385, #30890, #63871, #109225, #93862 ) ) ;
#101544=CARTESIAN_POINT ( 'NONE',  ( -17.17241001986523941, 1511.187213306747708, 179.6185504016045797 ) ) ;
#101545=CARTESIAN_POINT ( 'NONE',  ( -32.97913964219423377, 1511.187213306747708, 220.2739374644216355 ) ) ;
#101552=FACE_OUTER_BOUND ( 'NONE', #29127, .T. ) ;
#101558=ORIENTED_EDGE ( 'NONE', *, *, #11684, .T. ) ;
#101560=DIRECTION ( 'NONE',  ( -0.000000000000000000, -1.000000000000000000, -0.000000000000000000 ) ) ;
#101594=EDGE_CURVE ( 'NONE', #85718, #82045, #108958, .T. ) ;
#101597=CARTESIAN_POINT ( 'NONE',  ( -34.09079054513854601, 1524.667648926078982, 217.9059385276673879 ) ) ;
#101609=EDGE_LOOP ( 'NONE', ( #106480, #56972, #95103, #80959, #24360 ) ) ;
#101623=ORIENTED_EDGE ( 'NONE', *, *, #20070, .F. ) ;
#101627=ORIENTED_EDGE ( 'NONE', *, *, #72062, .F. ) ;
#101669=CIRCLE ( 'NONE', #28406, 1.000000000000000888 ) ;
#101680=EDGE_CURVE ( 'NONE', #35166, #4524, #48046, .T. ) ;
#101696=EDGE_CURVE ( 'NONE', #74476, #55773, #102403, .T. ) ;
#101700=ORIENTED_EDGE ( 'NONE', *, *, #48220, .T. ) ;
#101703=( BOUNDED_SURFACE ( )  B_SPLINE_SURFACE ( 3, 2, ( 
 ( #103745, #61233, #95348 ),
 ( #86940, #10231, #33767 ),
 ( #67963, #42537, #14567 ),
 ( #76143, #67757, #75059 ),
 ( #41994, #108639, #110288 ),
 ( #58795, #15110, #66119 ) ),
 .UNSPECIFIED., .F., .F., .T. ) 
 B_SPLINE_SURFACE_WITH_KNOTS ( ( 4, 2, 4 ),
 ( 3, 3 ),
 ( -2.081668171172168513E-17, 0.001312027981647304791, 0.002624055963294630398 ),
 ( 0.000000000000000000, 1.000000000000000000 ),
 .UNSPECIFIED. ) 
 GEOMETRIC_REPRESENTATION_ITEM ( )  RATIONAL_B_SPLINE_SURFACE ( (
 ( 1.000000000000000000, 0.9376006582765912256, 1.000000000000000000),
 ( 1.000000000000000000, 0.9569320108022220106, 1.000000000000000000),
 ( 1.000000000000000000, 0.9725743441619391083, 1.000000000000000000),
 ( 1.000000000000000000, 0.9942095667135121273, 1.000000000000000000),
 ( 1.000000000000000000, 1.000043666450747049, 1.000000000000000000),
 ( 1.000000000000000000, 1.000000000000000000, 1.000000000000000000) ) ) 
 REPRESENTATION_ITEM ( '' )  SURFACE ( )  );
#101705=VERTEX_POINT ( 'NONE', #62611 ) ;
#101706=CARTESIAN_POINT ( 'NONE',  ( -3.141363374988426660, 1525.159177407155767, 241.5359609335856419 ) ) ;
#101732=FACE_OUTER_BOUND ( 'NONE', #87234, .T. ) ;
#101738=CARTESIAN_POINT ( 'NONE',  ( 16.66701395081345538, 1523.530870145311155, 180.4846106723501578 ) ) ;
#101752=CARTESIAN_POINT ( 'NONE',  ( -18.86688640473562373, 1512.187213306747481, 237.4611898188522332 ) ) ;
#101760=CARTESIAN_POINT ( 'NONE',  ( 31.50799703744294789, 1524.382868172863937, 216.4233194664825248 ) ) ;
#101768=CARTESIAN_POINT ( 'NONE',  ( 17.17241001986483795, 1511.187213306747708, 179.6185504016043240 ) ) ;
#101771=CARTESIAN_POINT ( 'NONE',  ( -21.84020450211261277, 1523.481610118012895, 234.9798068777343474 ) ) ;
#101785=PLANE ( 'NONE',  #107015 ) ;
#101811=DIRECTION ( 'NONE',  ( -0.01594118961724032973, -0.9969860201949399814, 0.07592597717146747083 ) ) ;
#101815=ORIENTED_EDGE ( 'NONE', *, *, #50282, .F. ) ;
#101828=ADVANCED_FACE ( 'NONE', ( #72102 ), #26485, .T. ) ;
#101852=CARTESIAN_POINT ( 'NONE',  ( 2.646294106703178439, 1525.055402519451945, 241.6502424680635954 ) ) ;
#101853=ORIENTED_EDGE ( 'NONE', *, *, #9938, .T. ) ;
#101856=CARTESIAN_POINT ( 'NONE',  ( 32.15938645527133843, 1524.538768545233779, 202.1426263946930533 ) ) ;
#101869=LINE ( 'NONE', #33564, #38549 ) ;
#101881=CARTESIAN_POINT ( 'NONE',  ( -2.383407846124329765, 1522.906363951597314, 174.9517353176864844 ) ) ;
#101889=DIRECTION ( 'NONE',  ( 0.3090169943749423997, 0.000000000000000000, 0.9510565162951553075 ) ) ;
#101902=DIRECTION ( 'NONE',  ( 1.776356839400250465E-15, 0.000000000000000000, 1.000000000000000000 ) ) ;
#101911=ORIENTED_EDGE ( 'NONE', *, *, #49377, .F. ) ;
#101914=B_SPLINE_CURVE_WITH_KNOTS ( 'NONE', 3,
 ( #65851, #47934, #4289, #107832, #5373, #99969, #31120, #14861, #40628, #5931 ),
 .UNSPECIFIED., .F., .F.,
 ( 4, 2, 2, 2, 4 ),
 ( 3.469446951953614189E-18, 0.0007406479101618155831, 0.001481295820323627697, 0.002221943730485440027, 0.002962591640647251924 ),
 .UNSPECIFIED. ) ;
#101922=CARTESIAN_POINT ( 'NONE',  ( 0.4151546846821903003, 1522.382868172863937, 244.9330574173806951 ) ) ;
#101929=CARTESIAN_POINT ( 'NONE',  ( -30.31118248176270669, 1526.186458717542337, 216.6939452248811335 ) ) ;
#101937=EDGE_LOOP ( 'NONE', ( #34539, #60722, #58123, #54211 ) ) ;
#101956=AXIS2_PLACEMENT_3D ( 'NONE', #101544, #93160, #37129 ) ;
#101972=ORIENTED_EDGE ( 'NONE', *, *, #32256, .F. ) ;
#101981=EDGE_CURVE ( 'NONE', #911, #40948, #65969, .T. ) ;
#101998=CARTESIAN_POINT ( 'NONE',  ( -21.46337646344873562, 1524.972613296804184, 234.5040406280893706 ) ) ;
#102002=ORIENTED_EDGE ( 'NONE', *, *, #76957, .T. ) ;
#102015=DIRECTION ( 'NONE',  ( 0.000000000000000000, 0.000000000000000000, 1.000000000000000000 ) ) ;
#102016=ORIENTED_EDGE ( 'NONE', *, *, #103879, .T. ) ;
#102019=CARTESIAN_POINT ( 'NONE',  ( -173.8335085727391913, 1526.382868172863937, 317.3879012941878273 ) ) ;
#102026=CIRCLE ( 'NONE', #164, 2.000000000000001776 ) ;
#102030=CARTESIAN_POINT ( 'NONE',  ( 0.4151546846821903003, 1511.187213306747708, 174.3106345060153046 ) ) ;
#102046=ADVANCED_FACE ( 'NONE', ( #20975 ), #63785, .F. ) ;
#102047=CARTESIAN_POINT ( 'NONE',  ( -18.66420869458074705, 1526.382868172864164, 185.4599087859683095 ) ) ;
#102048=CARTESIAN_POINT ( 'NONE',  ( -29.30029655192939586, 1525.907212628473872, 196.8717316207790589 ) ) ;
#102052=ADVANCED_FACE ( 'NONE', ( #16820 ), #8441, .F. ) ;
#102056=EDGE_CURVE ( 'NONE', #30516, #6988, #38146, .T. ) ;
#102067=CARTESIAN_POINT ( 'NONE',  ( -30.90487439922565116, 1525.907212628473644, 201.8101144455181952 ) ) ;
#102070=CIRCLE ( 'NONE', #85941, 0.9999999999999988898 ) ;
#102079=ORIENTED_EDGE ( 'NONE', *, *, #77220, .T. ) ;
#102104=EDGE_CURVE ( 'NONE', #101260, #94134, #92708, .T. ) ;
#102108=DIRECTION ( 'NONE',  ( 0.000000000000000000, 1.000000000000000000, 0.000000000000000000 ) ) ;
#102128=CARTESIAN_POINT ( 'NONE',  ( 22.14913372576365802, 1525.402221411349956, 182.5746398196713187 ) ) ;
#102149=FACE_OUTER_BOUND ( 'NONE', #81588, .T. ) ;
#102151=DIRECTION ( 'NONE',  ( 0.000000000000000000, -1.000000000000000000, -0.000000000000000000 ) ) ;
#102162=AXIS2_PLACEMENT_3D ( 'NONE', #4918, #39059, #65407 ) ;
#102169=CARTESIAN_POINT ( 'NONE',  ( -21.28825147355507497, 1525.253972588461920, 183.8869829075299549 ) ) ;
#102172=CARTESIAN_POINT ( 'NONE',  ( -31.23437356469425907, 1518.913060387330006, 222.8968241038848248 ) ) ;
#102181=CARTESIAN_POINT ( 'NONE',  ( 31.02592223166955421, 1526.278758871496620, 198.2784374727472709 ) ) ;
#102207=CARTESIAN_POINT ( 'NONE',  ( -2.127574403380531720, 1524.244163922423695, 244.5104606571523789 ) ) ;
#102223=CARTESIAN_POINT ( 'NONE',  ( 1.488474718494355198, 1526.348417187218502, 239.9133697138477146 ) ) ;
#102231=EDGE_LOOP ( 'NONE', ( #27660, #12730, #6848, #14327 ) ) ;
#102235=ORIENTED_EDGE ( 'NONE', *, *, #48798, .F. ) ;
#102247=AXIS2_PLACEMENT_3D ( 'NONE', #83435, #91296, #48767 ) ;
#102253=CARTESIAN_POINT ( 'NONE',  ( 21.10561344245438065, 1525.661275128775742, 184.9336819308397537 ) ) ;
#102254=ORIENTED_EDGE ( 'NONE', *, *, #74428, .F. ) ;
#102258=CARTESIAN_POINT ( 'NONE',  ( 16.66936639845652834, 1518.913060387330006, 237.7608804993219280 ) ) ;
#102268=CIRCLE ( 'NONE', #54047, 24.33258347882036432 ) ;
#102276=CARTESIAN_POINT ( 'NONE',  ( -16.85976061912534263, 1525.821544997590536, 236.1944305375347994 ) ) ;
#102289=CARTESIAN_POINT ( 'NONE',  ( 2.664388089274176696, 1523.844789899199895, 176.1122506963328931 ) ) ;
#102299=CARTESIAN_POINT ( 'NONE',  ( 0.7251570665222376588, 1526.278758871496848, 241.9800489742293053 ) ) ;
#102300=VERTEX_POINT ( 'NONE', #16150 ) ;
#102301=EDGE_LOOP ( 'NONE', ( #97219, #72085, #31879, #71339 ) ) ;
#102331=EDGE_CURVE ( 'NONE', #87392, #38412, #37338, .T. ) ;
#102332=CARTESIAN_POINT ( 'NONE',  ( -32.38601544705579727, 1523.530935881284904, 216.1237228173876304 ) ) ;
#102339=VECTOR ( 'NONE', #50788, 1000.000000000000000 ) ;
#102385=ORIENTED_EDGE ( 'NONE', *, *, #87830, .T. ) ;
#102387=CARTESIAN_POINT ( 'NONE',  ( -32.78250617288034618, 1511.187213306747708, 218.3079823578271430 ) ) ;
#102395=CARTESIAN_POINT ( 'NONE',  ( 20.71343476517512627, 1524.726013923371283, 179.9059455038195381 ) ) ;
#102403=B_SPLINE_CURVE_WITH_KNOTS ( 'NONE', 3,
 ( #105122, #11063, #36811, #71002, #62039, #96164, #88318, #69889, #46344, #37365 ),
 .UNSPECIFIED., .F., .F.,
 ( 4, 2, 2, 2, 4 ),
 ( 0.000000000000000000, 0.0007189769279726045429, 0.001437953855945209086, 0.002156930783917813520, 0.002875907711890418172 ),
 .UNSPECIFIED. ) ;
#102411=CARTESIAN_POINT ( 'NONE',  ( 30.29139619032462249, 1523.843263703802677, 195.7510757159135721 ) ) ;
#102412=CARTESIAN_POINT ( 'NONE',  ( 28.81652261710051022, 1526.349684470114198, 220.0454371960102549 ) ) ;
#102415=CARTESIAN_POINT ( 'NONE',  ( 2.471035510942662050, 1525.556090473913628, 241.2503633023762575 ) ) ;
#102420=CARTESIAN_POINT ( 'NONE',  ( 31.79838993233245859, 1525.159177407155312, 202.0929476855948224 ) ) ;
#102452=VERTEX_POINT ( 'NONE', #91222 ) ;
#102456=CARTESIAN_POINT ( 'NONE',  ( -22.03465957474533710, 1522.862737210649584, 235.4136513321633117 ) ) ;
#102463=CARTESIAN_POINT ( 'NONE',  ( -18.15646965371402644, 1522.906363951597314, 238.1669781545290903 ) ) ;
#102483=CARTESIAN_POINT ( 'NONE',  ( -31.12456774391152337, 1525.960063244516959, 217.0912716842400698 ) ) ;
#102490=DIRECTION ( 'NONE',  ( 0.000000000000000000, 0.07083107041538988513, -0.9974883254774514763 ) ) ;
#102508=EDGE_LOOP ( 'NONE', ( #81858, #72670, #84335, #92206 ) ) ;
#102509=ORIENTED_EDGE ( 'NONE', *, *, #59852, .T. ) ;
#102523=ORIENTED_EDGE ( 'NONE', *, *, #42986, .T. ) ;
#102536=AXIS2_PLACEMENT_3D ( 'NONE', #19701, #1832, #53904 ) ;
#102550=CARTESIAN_POINT ( 'NONE',  ( 173.8335085727383955, 1524.382868172863937, 100.8557906292069930 ) ) ;
#102574=DIRECTION ( 'NONE',  ( 1.000000000000000000, -0.000000000000000000, 0.000000000000000000 ) ) ;
#102576=ORIENTED_EDGE ( 'NONE', *, *, #97273, .F. ) ;
#102595=DIRECTION ( 'NONE',  ( 0.000000000000000000, 0.000000000000000000, -1.000000000000000000 ) ) ;
#102597=CARTESIAN_POINT ( 'NONE',  ( 17.42134945962404657, 1525.253972588461465, 181.0775141427824337 ) ) ;
#102603=CARTESIAN_POINT ( 'NONE',  ( -1.491506560153236682, 1511.187213306747708, 242.6732489767341576 ) ) ;
#102605=CIRCLE ( 'NONE', #93657, 1.000000000000001332 ) ;
#102618=CARTESIAN_POINT ( 'NONE',  ( 21.95754362317981290, 1524.412928176728883, 184.5446601790259820 ) ) ;
#102619=ORIENTED_EDGE ( 'NONE', *, *, #65180, .T. ) ;
#102631=DIRECTION ( 'NONE',  ( 0.000000000000000000, 0.000000000000000000, -1.000000000000000000 ) ) ;
#102635=ORIENTED_EDGE ( 'NONE', *, *, #109619, .F. ) ;
#102651=ORIENTED_EDGE ( 'NONE', *, *, #65051, .F. ) ;
#102654=ORIENTED_EDGE ( 'NONE', *, *, #64704, .F. ) ;
#102663=CARTESIAN_POINT ( 'NONE',  ( 21.30823923614893189, 1524.382868172804365, 184.4507411017295908 ) ) ;
#102668=CARTESIAN_POINT ( 'NONE',  ( 22.08327125186925954, 1523.604703353109699, 184.4267662568470598 ) ) ;
#102669=EDGE_CURVE ( 'NONE', #39464, #42444, #99976, .T. ) ;
#102673=( BOUNDED_CURVE ( )  B_SPLINE_CURVE ( 3, ( #26237, #102395, #103499, #32982 ),
 .UNSPECIFIED., .F., .F. ) 
 B_SPLINE_CURVE_WITH_KNOTS ( ( 4, 4 ),
 ( 3.141592653589793116, 4.712388980384689674 ),
 .UNSPECIFIED. ) 
 CURVE ( )  GEOMETRIC_REPRESENTATION_ITEM ( )  RATIONAL_B_SPLINE_CURVE ( ( 1.000000000000000000, 0.8047378541243649375, 0.8047378541243649375, 1.000000000000000000 ) ) 
 REPRESENTATION_ITEM ( '' )  );
#102681=CARTESIAN_POINT ( 'NONE',  ( -22.08327125186908191, 1523.604703353109699, 233.8169256665491105 ) ) ;
#102693=CARTESIAN_POINT ( 'NONE',  ( 28.27139721233038827, 1526.382868172863937, 198.6830693683571667 ) ) ;
#102697=EDGE_CURVE ( 'NONE', #29992, #51216, #80339, .T. ) ;
#102705=CARTESIAN_POINT ( 'NONE',  ( -21.92050665148230237, 1524.523992613103019, 184.5693265961525640 ) ) ;
#102727=VECTOR ( 'NONE', #957, 1000.000000000000000 ) ;
#102734=CARTESIAN_POINT ( 'NONE',  ( 0.4151546846821903003, 1501.977400791986611, 175.3106345060153046 ) ) ;
#102746=DIRECTION ( 'NONE',  ( 0.000000000000000000, 1.000000000000000000, 0.000000000000000000 ) ) ;
#102756=CARTESIAN_POINT ( 'NONE',  ( 16.66700976312933946, 1523.530935881284904, 237.7590780485273569 ) ) ;
#102762=ORIENTED_EDGE ( 'NONE', *, *, #30691, .T. ) ;
#102766=CIRCLE ( 'NONE', #65248, 2.000000000000000444 ) ;
#102771=CARTESIAN_POINT ( 'NONE',  ( -21.32683180188266192, 1525.211477436245787, 183.8595778313278686 ) ) ;
#102776=CIRCLE ( 'NONE', #61664, 0.9999999999999411582 ) ;
#102779=DIRECTION ( 'NONE',  ( 0.000000000000000000, -0.07083107041561081951, -0.9974883254774358221 ) ) ;
#102780=CARTESIAN_POINT ( 'NONE',  ( 2.640434834157888933, 1526.748660780343471, 241.3121066639437515 ) ) ;
#102798=CARTESIAN_POINT ( 'NONE',  ( -30.36938634820402072, 1525.506926151471134, 221.4200516883777823 ) ) ;
#102799=AXIS2_PLACEMENT_3D ( 'NONE', #43056, #35193, #36295 ) ;
#102813=VECTOR ( 'NONE', #52147, 1000.000000000000000 ) ;
#102830=CARTESIAN_POINT ( 'NONE',  ( 2.136371150128812957, 1525.856065479248173, 176.8742974859703452 ) ) ;
#102843=ORIENTED_EDGE ( 'NONE', *, *, #80838, .F. ) ;
#102861=ORIENTED_EDGE ( 'NONE', *, *, #100983, .T. ) ;
#102866=EDGE_LOOP ( 'NONE', ( #83649, #13303, #66144, #38976 ) ) ;
#102874=DIRECTION ( 'NONE',  ( -0.9510565162951566398, 0.000000000000000000, -0.3090169943749382919 ) ) ;
#102884=AXIS2_PLACEMENT_3D ( 'NONE', #105078, #66953, #109492 ) ;
#102902=EDGE_LOOP ( 'NONE', ( #24503, #43419, #80533, #57254 ) ) ;
#102911=CARTESIAN_POINT ( 'NONE',  ( -2.570808432944301725, 1525.317359687841417, 176.7848587726591632 ) ) ;
#102913=CARTESIAN_POINT ( 'NONE',  ( 0.000000000000000000, 1526.382868172863937, 209.1218459616979999 ) ) ;
#102924=EDGE_LOOP ( 'NONE', ( #75076, #39299, #40129 ) ) ;
#102928=FACE_OUTER_BOUND ( 'NONE', #17056, .T. ) ;
#102933=AXIS2_PLACEMENT_3D ( 'NONE', #98650, #57235, #49365 ) ;
#102940=CARTESIAN_POINT ( 'NONE',  ( 0.000000000000000000, 1512.187213306747481, 209.1218459616979999 ) ) ;
#102947=ADVANCED_FACE ( 'NONE', ( #93458 ), #17959, .F. ) ;
#102955=EDGE_CURVE ( 'NONE', #85994, #71507, #107107, .T. ) ;
#102956=FACE_OUTER_BOUND ( 'NONE', #53189, .T. ) ;
#102958=CARTESIAN_POINT ( 'NONE',  ( -2.470168521978396203, 1512.187213306747481, 175.3649660270905315 ) ) ;
#102961=CARTESIAN_POINT ( 'NONE',  ( -1.770994272916314172, 1526.211528530236592, 177.6852349320064945 ) ) ;
#102978=CARTESIAN_POINT ( 'NONE',  ( -3.263276722441742717, 1524.760046179776054, 176.4719413543065514 ) ) ;
#102990=EDGE_CURVE ( 'NONE', #5947, #71944, #12771, .T. ) ;
#102999=CARTESIAN_POINT ( 'NONE',  ( -32.13439773946823408, 1525.163527997504616, 217.0282454366101206 ) ) ;
#103005=CARTESIAN_POINT ( 'NONE',  ( -16.56943046651996099, 1526.189899547014875, 182.6454527705575970 ) ) ;
#103009=DIRECTION ( 'NONE',  ( -0.000000000000000000, -1.000000000000000000, -0.000000000000000000 ) ) ;
#103037=EDGE_LOOP ( 'NONE', ( #6493, #99814, #30733, #41203 ) ) ;
#103060=ORIENTED_EDGE ( 'NONE', *, *, #25434, .T. ) ;
#103064=ORIENTED_EDGE ( 'NONE', *, *, #57709, .F. ) ;
#103071=DIRECTION ( 'NONE',  ( -0.4090087482554295439, 0.000000000000000000, -0.9125304618753977692 ) ) ;
#103088=CARTESIAN_POINT ( 'NONE',  ( 0.8350686643532190256, 1526.382868172863937, 177.3106345060153046 ) ) ;
#103101=CARTESIAN_POINT ( 'NONE',  ( -20.49599333844820137, 1525.960063244516959, 233.8638087104926058 ) ) ;
#103105=ORIENTED_EDGE ( 'NONE', *, *, #43319, .T. ) ;
#103128=CARTESIAN_POINT ( 'NONE',  ( -17.19739463999666285, 1525.960063244516959, 181.9833109756550584 ) ) ;
#103131=CARTESIAN_POINT ( 'NONE',  ( 0.000000000000000000, 1526.382868172863937, 240.9330574173806951 ) ) ;
#103158=CARTESIAN_POINT ( 'NONE',  ( 17.34064570863430887, 1525.506926151471589, 181.3217111118486571 ) ) ;
#103166=DIRECTION ( 'NONE',  ( -0.8200914087126657259, -0.4884709562387143933, -0.2980708074718346201 ) ) ;
#103176=ORIENTED_EDGE ( 'NONE', *, *, #39710, .F. ) ;
#103197=ORIENTED_EDGE ( 'NONE', *, *, #11712, .T. ) ;
#103221=DIRECTION ( 'NONE',  ( 0.8672669759446699489, 0.000000000000000000, 0.4978433412588613716 ) ) ;
#103222=CARTESIAN_POINT ( 'NONE',  ( 22.03465957474550407, 1522.382868172863937, 182.8300405912328586 ) ) ;
#103227=CARTESIAN_POINT ( 'NONE',  ( 0.000000000000000000, 1523.409940573003951, 233.8211094035767985 ) ) ;
#103228=EDGE_CURVE ( 'NONE', #88474, #100188, #4640, .T. ) ;
#103229=CARTESIAN_POINT ( 'NONE',  ( 30.01999557802941254, 1525.848196786131666, 221.1300219709211490 ) ) ;
#103232=CARTESIAN_POINT ( 'NONE',  ( 30.60461244942487014, 1523.621879633028811, 221.8232741897816993 ) ) ;
#103252=LINE ( 'NONE', #838, #55670 ) ;
#103258=CARTESIAN_POINT ( 'NONE',  ( -17.16388877745028907, 1523.678648413191695, 238.6174304775216228 ) ) ;
#103260=CARTESIAN_POINT ( 'NONE',  ( -21.66438254905709826, 1525.042337199240137, 184.7096065694357208 ) ) ;
#103265=CARTESIAN_POINT ( 'NONE',  ( -22.08523692261585580, 1523.530935881284904, 184.4211863326293326 ) ) ;
#103269=CIRCLE ( 'NONE', #78277, 2.000000000000001776 ) ;
#103286=CARTESIAN_POINT ( 'NONE',  ( 20.58427237330526438, 1512.187213306747481, 216.4826520421586338 ) ) ;
#103287=CARTESIAN_POINT ( 'NONE',  ( -173.8335085727399871, 1524.382868172863937, 100.8557906292094231 ) ) ;
#103290=DIRECTION ( 'NONE',  ( 0.000000000000000000, 1.000000000000000000, 0.000000000000000000 ) ) ;
#103308=B_SPLINE_CURVE_WITH_KNOTS ( 'NONE', 3,
 ( #80228, #107626, #21387, #46099, #4624, #39319 ),
 .UNSPECIFIED., .F., .F.,
 ( 4, 2, 4 ),
 ( 2.797157557069881010E-17, 0.001087661325621672604, 0.002175322651243317019 ),
 .UNSPECIFIED. ) ;
#103322=ORIENTED_EDGE ( 'NONE', *, *, #68117, .T. ) ;
#103323=CIRCLE ( 'NONE', #92624, 32.13701971169416538 ) ;
#103327=VECTOR ( 'NONE', #56899, 1000.000000000000000 ) ;
#103333=CARTESIAN_POINT ( 'NONE',  ( -204.2714532754873744, 1526.382868172863937, 223.7095399770904010 ) ) ;
#103346=ORIENTED_EDGE ( 'NONE', *, *, #324, .F. ) ;
#103355=CARTESIAN_POINT ( 'NONE',  ( -30.16752008203960500, 1524.964158026965833, 221.7255342961994700 ) ) ;
#103370=CARTESIAN_POINT ( 'NONE',  ( 32.38845791999500534, 1518.913060387330006, 216.1254071228445639 ) ) ;
#103384=CARTESIAN_POINT ( 'NONE',  ( -29.99674465255699474, 1524.860077346004800, 195.9762169038188517 ) ) ;
#103385=CARTESIAN_POINT ( 'NONE',  ( -20.69714284706251917, 1525.848196786131211, 233.9618279170393009 ) ) ;
#103393=CARTESIAN_POINT ( 'NONE',  ( 2.792392588003326903, 1526.382868172863937, 241.3440112565233164 ) ) ;
#103395=CARTESIAN_POINT ( 'NONE',  ( -32.38845791999504797, 1512.187213306747481, 202.1182848005516348 ) ) ;
#103401=VECTOR ( 'NONE', #62888, 1000.000000000000114 ) ;
#103406=AXIS2_PLACEMENT_3D ( 'NONE', #50430, #59936, #100789 ) ;
#103447=EDGE_CURVE ( 'NONE', #36569, #82691, #31393, .T. ) ;
#103460=ADVANCED_FACE ( 'NONE', ( #26951 ), #52714, .T. ) ;
#103461=ORIENTED_EDGE ( 'NONE', *, *, #9797, .F. ) ;
#103470=CARTESIAN_POINT ( 'NONE',  ( -2.311632204762886111, 1525.506926151471362, 176.4384886094890987 ) ) ;
#103493=ADVANCED_FACE ( 'NONE', ( #89047 ), #25152, .T. ) ;
#103499=CARTESIAN_POINT ( 'NONE',  ( 19.59884465730813830, 1526.382868172863937, 181.1441328703420481 ) ) ;
#103510=DIRECTION ( 'NONE',  ( -0.06728379684272094152, -0.9969860201949397593, -0.03862338952348134263 ) ) ;
#103514=CARTESIAN_POINT ( 'NONE',  ( 30.15968401513964636, 1524.412455883367556, 195.8336456173444162 ) ) ;
#103516=CARTESIAN_POINT ( 'NONE',  ( -16.57542919120515279, 1524.538768545233779, 180.6931493670368525 ) ) ;
#103524=DIRECTION ( 'NONE',  ( 0.000000000000000000, 0.000000000000000000, 1.000000000000000000 ) ) ;
#103531=PLANE ( 'NONE',  #51196 ) ;
#103563=CARTESIAN_POINT ( 'NONE',  ( -32.22536377336270164, 1523.621879633028811, 216.8351145222434013 ) ) ;
#103582=AXIS2_PLACEMENT_3D ( 'NONE', #61142, #70092, #86849 ) ;
#103587=CIRCLE ( 'NONE', #21078, 1.000000000000000888 ) ;
#103636=ORIENTED_EDGE ( 'NONE', *, *, #104861, .T. ) ;
#103652=CARTESIAN_POINT ( 'NONE',  ( -21.38516915558007270, 1512.187213306747481, 180.3939891059723664 ) ) ;
#103658=CIRCLE ( 'NONE', #105433, 0.9999999999999015232 ) ;
#103661=CARTESIAN_POINT ( 'NONE',  ( 0.5890887500919903541, 1526.382868172863937, 174.9674887555077021 ) ) ;
#103675=( BOUNDED_CURVE ( )  B_SPLINE_CURVE ( 3, ( #85777, #77393, #21162, #96815 ),
 .UNSPECIFIED., .F., .F. ) 
 B_SPLINE_CURVE_WITH_KNOTS ( ( 4, 4 ),
 ( 3.141592653589793116, 4.712388980384689674 ),
 .UNSPECIFIED. ) 
 CURVE ( )  GEOMETRIC_REPRESENTATION_ITEM ( )  RATIONAL_B_SPLINE_CURVE ( ( 1.000000000000000000, 0.8047378541243649375, 0.8047378541243649375, 1.000000000000000000 ) ) 
 REPRESENTATION_ITEM ( '' )  );
#103684=FACE_OUTER_BOUND ( 'NONE', #106165, .T. ) ;
#103685=CARTESIAN_POINT ( 'NONE',  ( -1.771001175045461062, 1526.211523310372513, 240.5584728653311970 ) ) ;
#103711=CARTESIAN_POINT ( 'NONE',  ( 20.55201027734738872, 1526.382868172863937, 236.4070436938629030 ) ) ;
#103713=CARTESIAN_POINT ( 'NONE',  ( 29.52630218505380810, 1525.661276915132476, 196.5237718006094099 ) ) ;
#103745=CARTESIAN_POINT ( 'NONE',  ( -31.12456774391182535, 1525.960063244516959, 201.1524202391566121 ) ) ;
#103757=CARTESIAN_POINT ( 'NONE',  ( 22.04658049762480942, 1524.075132568165373, 184.4787145761434601 ) ) ;
#103761=DIRECTION ( 'NONE',  ( -0.000000000000000000, -1.000000000000000000, -0.000000000000000000 ) ) ;
#103782=DIRECTION ( 'NONE',  ( 0.000000000000000000, 1.000000000000000000, 0.000000000000000000 ) ) ;
#103806=CARTESIAN_POINT ( 'NONE',  ( 31.32995031131202524, 1523.678648413191695, 221.9013357025044115 ) ) ;
#103827=ORIENTED_EDGE ( 'NONE', *, *, #13996, .F. ) ;
#103831=CARTESIAN_POINT ( 'NONE',  ( 29.13505175353622079, 1526.073429442291854, 197.1475357601794940 ) ) ;
#103848=CIRCLE ( 'NONE', #55603, 33.13701971169416538 ) ;
#103851=CARTESIAN_POINT ( 'NONE',  ( -31.40702543711151762, 1523.611961620354123, 196.3340613265682464 ) ) ;
#103878=VERTEX_POINT ( 'NONE', #37976 ) ;
#103879=EDGE_CURVE ( 'NONE', #5789, #8681, #52857, .T. ) ;
#103905=ORIENTED_EDGE ( 'NONE', *, *, #11687, .T. ) ;
#103935=CARTESIAN_POINT ( 'NONE',  ( 21.83863729849015911, 1523.580204110582144, 234.9763103240493081 ) ) ;
#103941=DIRECTION ( 'NONE',  ( -0.000000000000000000, 1.000000000000000000, -0.000000000000000000 ) ) ;
#103952=CIRCLE ( 'NONE', #75363, 1.000000000000007994 ) ;
#103957=CARTESIAN_POINT ( 'NONE',  ( -32.36284091029009602, 1525.878013734320348, 199.2622049721628628 ) ) ;
#103961=CARTESIAN_POINT ( 'NONE',  ( 16.66936639839085643, 1523.456924617336881, 180.4828114240358161 ) ) ;
#103966=CARTESIAN_POINT ( 'NONE',  ( 0.7800921441517267851, 1526.382868172863937, 241.4567505818334610 ) ) ;
#103967=EDGE_LOOP ( 'NONE', ( #46866, #24744, #29590, #9168, #96755, #57546, #86084, #37257 ) ) ;
#103996=AXIS2_PLACEMENT_3D ( 'NONE', #77962, #24769, #51119 ) ;
#104006=ORIENTED_EDGE ( 'NONE', *, *, #101368, .T. ) ;
#104010=DIRECTION ( 'NONE',  ( 0.7414773880254775795, -1.225281874271768203E-16, 0.6709778558543607607 ) ) ;
#104014=AXIS2_PLACEMENT_3D ( 'NONE', #66130, #14021, #7292 ) ;
#104015=DIRECTION ( 'NONE',  ( 0.000000000000000000, 1.000000000000000000, 0.000000000000000000 ) ) ;
#104030=CIRCLE ( 'NONE', #7477, 1.000000000000000666 ) ;
#104041=ORIENTED_EDGE ( 'NONE', *, *, #1576, .F. ) ;
#104050=EDGE_CURVE ( 'NONE', #15491, #92642, #107554, .T. ) ;
#104064=ORIENTED_EDGE ( 'NONE', *, *, #42395, .T. ) ;
#104080=CARTESIAN_POINT ( 'NONE',  ( 2.691689582132314573, 1524.775785348137561, 241.8132190896513407 ) ) ;
#104083=CARTESIAN_POINT ( 'NONE',  ( 19.90023153800532185, 1526.278758871497303, 235.2784539741592198 ) ) ;
#104087=EDGE_CURVE ( 'NONE', #58183, #44415, #83915, .T. ) ;
#104098=EDGE_CURVE ( 'NONE', #92019, #82365, #27432, .T. ) ;
#104101=CARTESIAN_POINT ( 'NONE',  ( -2.738357795398948635, 1525.795403383247276, 177.3070688927101060 ) ) ;
#104107=DIRECTION ( 'NONE',  ( -1.000000000000000000, 0.000000000000000000, 0.000000000000000000 ) ) ;
#104124=ADVANCED_FACE ( 'NONE', ( #14400 ), #36633, .F. ) ;
#104136=CARTESIAN_POINT ( 'NONE',  ( -32.86470158750949366, 1523.580203803270933, 201.0415738342975089 ) ) ;
#104144=DIRECTION ( 'NONE',  ( 0.7414773880254614813, -0.000000000000000000, -0.6709778558543786353 ) ) ;
#104148=CARTESIAN_POINT ( 'NONE',  ( -32.41382812665785451, 1525.581535527370079, 220.2604433702386189 ) ) ;
#104151=DIRECTION ( 'NONE',  ( -1.776356839400250859E-15, 0.000000000000000000, -1.000000000000000000 ) ) ;
#104165=CARTESIAN_POINT ( 'NONE',  ( 19.53786426059019021, 1512.187213306747481, 181.5239794925693388 ) ) ;
#104175=DIRECTION ( 'NONE',  ( -0.7414773880254711402, 0.000000000000000000, -0.6709778558543678662 ) ) ;
#104196=DIRECTION ( 'NONE',  ( -0.000000000000000000, -1.000000000000000000, -0.000000000000000000 ) ) ;
#104220=B_SPLINE_CURVE_WITH_KNOTS ( 'NONE', 3,
 ( #38685, #73412, #98038, #72860 ),
 .UNSPECIFIED., .F., .F.,
 ( 4, 4 ),
 ( 0.000000000000000000, 0.0002960034161023847310 ),
 .UNSPECIFIED. ) ;
#104225=CARTESIAN_POINT ( 'NONE',  ( -18.40343465886419949, 1525.402221411349274, 179.8532301504590407 ) ) ;
#104227=DIRECTION ( 'NONE',  ( 0.000000000000000000, 1.000000000000000000, 0.000000000000000000 ) ) ;
#104231=DIRECTION ( 'NONE',  ( -0.000000000000000000, -1.000000000000000000, -0.000000000000000000 ) ) ;
#104239=LINE ( 'NONE', #28077, #52077 ) ;
#104247=CARTESIAN_POINT ( 'NONE',  ( -32.36284091028927890, 1525.878013734321257, 218.9814869512302096 ) ) ;
#104248=CARTESIAN_POINT ( 'NONE',  ( -21.38516915557943321, 1522.382868172863937, 237.8497028174240313 ) ) ;
#104261=DIRECTION ( 'NONE',  ( 0.4978433412588781914, 0.000000000000000000, 0.8672669759446606230 ) ) ;
#104266=CARTESIAN_POINT ( 'NONE',  ( 29.86461515634908892, 1525.960063244516959, 197.2746849027934957 ) ) ;
#104329=EDGE_CURVE ( 'NONE', #110178, #50084, #12556, .T. ) ;
#104336=( BOUNDED_SURFACE ( )  B_SPLINE_SURFACE ( 3, 2, ( 
 ( #40889, #57176, #57725 ),
 ( #67223, #24070, #84546 ),
 ( #40339, #75071, #41458 ),
 ( #66675, #8380, #33033 ),
 ( #73961, #91843, #83995 ),
 ( #42004, #109219, #109755 ),
 ( #92384, #15121, #7835 ),
 ( #76152, #101321, #101881 ),
 ( #32505, #100779, #59376 ),
 ( #108091, #83437, #108651 ) ),
 .UNSPECIFIED., .F., .F., .F. ) 
 B_SPLINE_SURFACE_WITH_KNOTS ( ( 4, 2, 2, 2, 4 ),
 ( 3, 3 ),
 ( 1.570796326794896558, 1.963495408493620697, 2.356194490192344837, 2.748893571891068976, 3.141592653589793116 ),
 ( 0.000000000000000000, 1.000000000000000000 ),
 .UNSPECIFIED. ) 
 GEOMETRIC_REPRESENTATION_ITEM ( )  RATIONAL_B_SPLINE_SURFACE ( (
 ( 1.000000000000000000, 0.7071067811865857644, 1.000000000000000000),
 ( 1.000000000000000000, 0.7166207884818905915, 1.000000000000000000),
 ( 1.000000000000000000, 0.7259222650911381081, 1.000000000000000000),
 ( 1.000000000000000000, 0.7428408967926047879, 1.000000000000000000),
 ( 1.000000000000000000, 0.7504512394524444074, 1.000000000000000000),
 ( 1.000000000000000000, 0.7630177051950547407, 1.000000000000000000),
 ( 1.000000000000000000, 0.7679730451973306726, 1.000000000000000000),
 ( 1.000000000000000000, 0.7746454561797161409, 1.000000000000000000),
 ( 1.000000000000000000, 0.7763684247035325114, 1.000000000000000000),
 ( 1.000000000000000000, 0.7763623250684303922, 1.000000000000000000) ) ) 
 REPRESENTATION_ITEM ( '' )  SURFACE ( )  );
#104353=CARTESIAN_POINT ( 'NONE',  ( 2.902322711624676882E-15, 1518.913060387330006, 232.8211094035767985 ) ) ;
#104356=CARTESIAN_POINT ( 'NONE',  ( -2.356903266504112082, 1525.394057003702756, 241.9297787646439417 ) ) ;
#104364=CARTESIAN_POINT ( 'NONE',  ( -16.50400130224727135, 1525.907212628473872, 236.2546788475582105 ) ) ;
#104367=CARTESIAN_POINT ( 'NONE',  ( 30.37359097063835733, 1526.143142182266274, 216.9284661788419442 ) ) ;
#104370=EDGE_CURVE ( 'NONE', #109192, #36569, #53498, .T. ) ;
#104377=ORIENTED_EDGE ( 'NONE', *, *, #104518, .T. ) ;
#104380=DIRECTION ( 'NONE',  ( -0.2054769195713184726, -5.792241587466808811E-16, -0.9786619618251657382 ) ) ;
#104395=EDGE_LOOP ( 'NONE', ( #98469, #49930, #3124, #20319 ) ) ;
#104396=CARTESIAN_POINT ( 'NONE',  ( 18.83964618864519380, 1526.382868172863937, 185.4251846830098316 ) ) ;
#104402=FACE_OUTER_BOUND ( 'NONE', #101609, .T. ) ;
#104417=CARTESIAN_POINT ( 'NONE',  ( 2.038646110889678287, 1525.960063244516959, 177.0579350083066004 ) ) ;
#104418=DIRECTION ( 'NONE',  ( 0.000000000000000000, 0.000000000000000000, -1.000000000000000000 ) ) ;
#104434=FACE_OUTER_BOUND ( 'NONE', #77729, .T. ) ;
#104439=FACE_OUTER_BOUND ( 'NONE', #74569, .T. ) ;
#104448=CARTESIAN_POINT ( 'NONE',  ( 0.000000000000000000, 1526.382868172863937, 209.1218459616979999 ) ) ;
#104449=CARTESIAN_POINT ( 'NONE',  ( 21.37468300741550919, 1525.408337840050308, 233.4084488120059859 ) ) ;
#104452=CARTESIAN_POINT ( 'NONE',  ( -22.75273496409615603, 1523.382868172864164, 183.6728937936775310 ) ) ;
#104510=CARTESIAN_POINT ( 'NONE',  ( -21.83550407203936672, 1523.678648413191695, 183.2743720722710634 ) ) ;
#104518=EDGE_CURVE ( 'NONE', #90367, #58486, #26773, .T. ) ;
#104538=DIRECTION ( 'NONE',  ( 0.8672669759446693938, 6.017873532443186100E-15, 0.4978433412588624818 ) ) ;
#104549=DIRECTION ( 'NONE',  ( 0.000000000000000000, 0.000000000000000000, 1.000000000000000000 ) ) ;
#104560=CIRCLE ( 'NONE', #56288, 32.13701971169416538 ) ;
#104587=CARTESIAN_POINT ( 'NONE',  ( -2.470955845399090300, 1523.580203803270933, 242.8749759691355621 ) ) ;
#104592=CYLINDRICAL_SURFACE ( 'NONE', #69330, 1.999999999999994005 ) ;
#104593=CARTESIAN_POINT ( 'NONE',  ( -29.13898522074213560, 1526.069472839378477, 197.1409705599818381 ) ) ;
#104599=CIRCLE ( 'NONE', #56334, 0.9999999999999887867 ) ;
#104610=CARTESIAN_POINT ( 'NONE',  ( -22.08327125186908191, 1523.604703353109699, 233.8169256665491105 ) ) ;
#104618=ORIENTED_EDGE ( 'NONE', *, *, #45458, .F. ) ;
#104632=DIRECTION ( 'NONE',  ( -0.2054769195713186114, -6.237798632656567355E-16, 0.9786619618251657382 ) ) ;
#104637=DIRECTION ( 'NONE',  ( 0.000000000000000000, 1.000000000000000000, 0.000000000000000000 ) ) ;
#104638=CARTESIAN_POINT ( 'NONE',  ( 21.33281718256677451, 1523.429859730330236, 237.7590525783467683 ) ) ;
#104644=DIRECTION ( 'NONE',  ( 0.000000000000000000, -1.000000000000000000, 0.000000000000000000 ) ) ;
#104646=CARTESIAN_POINT ( 'NONE',  ( 31.44837959398592986, 1511.187213306747708, 220.9083067115976462 ) ) ;
#104673=CARTESIAN_POINT ( 'NONE',  ( -32.16538354509416564, 1524.524650307258071, 216.1007197859166808 ) ) ;
#104674=ORIENTED_EDGE ( 'NONE', *, *, #10708, .T. ) ;
#104676=ORIENTED_EDGE ( 'NONE', *, *, #31527, .T. ) ;
#104682=DIRECTION ( 'NONE',  ( -0.8672669759446604010, 0.000000000000000000, 0.4978433412588780804 ) ) ;
#104688=VERTEX_POINT ( 'NONE', #21706 ) ;
#104699=CARTESIAN_POINT ( 'NONE',  ( 31.62138935264962569, 1525.231887713385504, 201.5806591012467663 ) ) ;
#104705=FACE_OUTER_BOUND ( 'NONE', #62489, .T. ) ;
#104715=AXIS2_PLACEMENT_3D ( 'NONE', #90244, #13527, #39303 ) ;
#104716=CARTESIAN_POINT ( 'NONE',  ( 31.34137657934008558, 1523.382868172864164, 196.3411265156547358 ) ) ;
#104728=EDGE_LOOP ( 'NONE', ( #42972, #24268, #7040 ) ) ;
#104730=DIRECTION ( 'NONE',  ( 1.000000000000000000, -0.000000000000000000, 1.224646799147353207E-16 ) ) ;
#104734=ORIENTED_EDGE ( 'NONE', *, *, #105505, .F. ) ;
#104740=CYLINDRICAL_SURFACE ( 'NONE', #36856, 30.10786454236638576 ) ;
#104751=ORIENTED_EDGE ( 'NONE', *, *, #28913, .F. ) ;
#104754=ORIENTED_EDGE ( 'NONE', *, *, #28391, .F. ) ;
#104778=CARTESIAN_POINT ( 'NONE',  ( -20.68299398335333095, 1525.856065479256586, 233.9549332500229468 ) ) ;
#104798=CARTESIAN_POINT ( 'NONE',  ( -32.59719044532463528, 1523.982201850120191, 217.0485567930471120 ) ) ;
#104806=CARTESIAN_POINT ( 'NONE',  ( -16.81497685297394895, 1526.382868172864164, 183.7037134202652169 ) ) ;
#104809=DIRECTION ( 'NONE',  ( 0.000000000000000000, 1.000000000000000000, 0.000000000000000000 ) ) ;
#104818=CARTESIAN_POINT ( 'NONE',  ( 21.38516915557986309, 1522.382868172863937, 237.8497028174237471 ) ) ;
#104844=CARTESIAN_POINT ( 'NONE',  ( 21.38516915557964637, 1524.726013923371283, 180.3939891059721390 ) ) ;
#104861=EDGE_CURVE ( 'NONE', #23879, #101207, #80419, .T. ) ;
#104904=CARTESIAN_POINT ( 'NONE',  ( 28.27139721233038827, 1526.382868172863937, 198.6830693683571667 ) ) ;
#104907=EDGE_CURVE ( 'NONE', #94625, #81986, #28538, .T. ) ;
#104927=CARTESIAN_POINT ( 'NONE',  ( 29.37542415142312535, 1526.382868172864164, 217.2587022579320433 ) ) ;
#104948=DIRECTION ( 'NONE',  ( 0.000000000000000000, 1.000000000000000000, 0.000000000000000000 ) ) ;
#104951=EDGE_CURVE ( 'NONE', #85993, #95247, #92663, .T. ) ;
#104959=VECTOR ( 'NONE', #63946, 1000.000000000000000 ) ;
#104961=DIRECTION ( 'NONE',  ( 0.000000000000000000, 0.000000000000000000, -1.000000000000000000 ) ) ;
#104975=ADVANCED_FACE ( 'NONE', ( #99949 ), #57443, .T. ) ;
#104995=EDGE_CURVE ( 'NONE', #91781, #79695, #105443, .T. ) ;
#104997=CARTESIAN_POINT ( 'NONE',  ( 16.66936639845652479, 1523.456872492435195, 237.7608804993219280 ) ) ;
#105007=CARTESIAN_POINT ( 'NONE',  ( 20.88377839294442495, 1525.556090473946824, 233.6619242631579141 ) ) ;
#105017=ORIENTED_EDGE ( 'NONE', *, *, #55442, .T. ) ;
#105031=AXIS2_PLACEMENT_3D ( 'NONE', #88536, #3442, #108492 ) ;
#105032=CARTESIAN_POINT ( 'NONE',  ( 19.91074080903766230, 1526.211528530236592, 233.5136342147586674 ) ) ;
#105039=AXIS2_PLACEMENT_3D ( 'NONE', #17196, #34589, #18871 ) ;
#105040=DIRECTION ( 'NONE',  ( -0.4882662618185321102, -0.4884709562387601345, 0.7231819843448452634 ) ) ;
#105048=ORIENTED_EDGE ( 'NONE', *, *, #91702, .F. ) ;
#105069=CARTESIAN_POINT ( 'NONE',  ( -34.68852446352950381, 1522.382868172863937, 199.9946320047955624 ) ) ;
#105078=CARTESIAN_POINT ( 'NONE',  ( -19.53786426059057746, 1512.187213306747481, 181.5239794925695946 ) ) ;
#105086=CARTESIAN_POINT ( 'NONE',  ( -2.471036798109852217, 1525.556089352344543, 241.2503651499576165 ) ) ;
#105101=CARTESIAN_POINT ( 'NONE',  ( 30.31052258194597115, 1523.604703353109699, 222.4930856806589929 ) ) ;
#105104=CARTESIAN_POINT ( 'NONE',  ( 31.81407709660776817, 1522.862737210649584, 221.9534378623329474 ) ) ;
#105111=TOROIDAL_SURFACE ( 'NONE', #56840, 1.000000000000000000, 1.000000000000000000 ) ;
#105115=CARTESIAN_POINT ( 'NONE',  ( 22.75273496409577945, 1511.187213306747708, 183.6728937936772184 ) ) ;
#105120=AXIS2_PLACEMENT_3D ( 'NONE', #11889, #80746, #87501 ) ;
#105122=CARTESIAN_POINT ( 'NONE',  ( 2.596261494520225366, 1525.907212628473644, 240.7735774411713123 ) ) ;
#105124=ORIENTED_EDGE ( 'NONE', *, *, #100983, .F. ) ;
#105132=EDGE_CURVE ( 'NONE', #57779, #36364, #62549, .T. ) ;
#105133=EDGE_CURVE ( 'NONE', #40151, #30075, #55215, .T. ) ;
#105138=VERTEX_POINT ( 'NONE', #27130 ) ;
#105140=ORIENTED_EDGE ( 'NONE', *, *, #4401, .T. ) ;
#105167=AXIS2_PLACEMENT_3D ( 'NONE', #42878, #102746, #26040 ) ;
#105169=EDGE_CURVE ( 'NONE', #75901, #40683, #83990, .T. ) ;
#105180=ORIENTED_EDGE ( 'NONE', *, *, #20964, .T. ) ;
#105190=CIRCLE ( 'NONE', #37256, 1.000000000000000888 ) ;
#105193=VECTOR ( 'NONE', #53766, 1000.000000000000000 ) ;
#105198=CARTESIAN_POINT ( 'NONE',  ( 21.38516915557987375, 1522.382868172863937, 237.8497028174237755 ) ) ;
#105207=CARTESIAN_POINT ( 'NONE',  ( -28.96738428617770111, 1526.189899547014875, 197.4412607874185142 ) ) ;
#105210=DIRECTION ( 'NONE',  ( 0.000000000000000000, 1.000000000000000000, 0.000000000000000000 ) ) ;
#105233=CARTESIAN_POINT ( 'NONE',  ( -32.85805783624299892, 1523.678648413191695, 217.1983043299907763 ) ) ;
#105246=CARTESIAN_POINT ( 'NONE',  ( -32.86802468386296994, 1523.481610426287716, 201.0396662540046577 ) ) ;
#105250=EDGE_LOOP ( 'NONE', ( #10843, #86633, #29422, #107642 ) ) ;
#105256=CARTESIAN_POINT ( 'NONE',  ( 31.52384642521029789, 1525.730671215508664, 201.2079779568606455 ) ) ;
#105303=VERTEX_POINT ( 'NONE', #64611 ) ;
#105307=ORIENTED_EDGE ( 'NONE', *, *, #96189, .F. ) ;
#105326=CIRCLE ( 'NONE', #19466, 1.000000000000000888 ) ;
#105330=CARTESIAN_POINT ( 'NONE',  ( -17.61183580542381577, 1523.982201850120191, 180.5695639321406532 ) ) ;
#105332=CARTESIAN_POINT ( 'NONE',  ( -0.4151546846821903003, 1501.977400791986611, 244.9330574173806951 ) ) ;
#105333=( BOUNDED_CURVE ( )  B_SPLINE_CURVE ( 3, ( #6268, #40966, #39874, #23049 ),
 .UNSPECIFIED., .F., .F. ) 
 B_SPLINE_CURVE_WITH_KNOTS ( ( 4, 4 ),
 ( 4.712388980384689674, 6.283185307179586232 ),
 .UNSPECIFIED. ) 
 CURVE ( )  GEOMETRIC_REPRESENTATION_ITEM ( )  RATIONAL_B_SPLINE_CURVE ( ( 1.000000000000000000, 0.8047378541243649375, 0.8047378541243649375, 1.000000000000000000 ) ) 
 REPRESENTATION_ITEM ( '' )  );
#105345=FACE_OUTER_BOUND ( 'NONE', #95942, .T. ) ;
#105359=ADVANCED_FACE ( 'NONE', ( #47238 ), #107180, .T. ) ;
#105362=CARTESIAN_POINT ( 'NONE',  ( -17.12015336051603853, 1526.107876515966382, 182.3088662919814738 ) ) ;
#105381=CARTESIAN_POINT ( 'NONE',  ( 19.00259723423673464, 1526.382868173645875, 232.9129335399838112 ) ) ;
#105433=AXIS2_PLACEMENT_3D ( 'NONE', #102780, #83370, #26074 ) ;
#105443=CIRCLE ( 'NONE', #12474, 2.000000000000001776 ) ;
#105464=ADVANCED_FACE ( 'NONE', ( #99262 ), #55930, .F. ) ;
#105489=VERTEX_POINT ( 'NONE', #39380 ) ;
#105504=CARTESIAN_POINT ( 'NONE',  ( -31.23437356469455040, 1512.187213306747481, 196.3468678195118287 ) ) ;
#105505=EDGE_CURVE ( 'NONE', #44004, #54639, #7201, .T. ) ;
#105509=AXIS2_PLACEMENT_3D ( 'NONE', #62047, #105697, #1575 ) ;
#105511=EDGE_CURVE ( 'NONE', #36569, #96612, #27538, .T. ) ;
#105515=CARTESIAN_POINT ( 'NONE',  ( -31.03088476499778281, 1523.982201850120191, 196.3745419238244381 ) ) ;
#105553=DIRECTION ( 'NONE',  ( 0.000000000000000000, 0.3666799630584695047, 0.9303471420343265574 ) ) ;
#105572=DIRECTION ( 'NONE',  ( -0.2054769195713296304, 0.000000000000000000, 0.9786619618251631847 ) ) ;
#105581=B_SPLINE_CURVE_WITH_KNOTS ( 'NONE', 3,
 ( #48796, #5108, #20796, #98064 ),
 .UNSPECIFIED., .F., .F.,
 ( 4, 4 ),
 ( 0.000000000000000000, 0.0002960034161023848394 ),
 .UNSPECIFIED. ) ;
#105589=CIRCLE ( 'NONE', #71655, 1.000000000000000888 ) ;
#105590=CARTESIAN_POINT ( 'NONE',  ( 2.485536755124557740, 1523.919943579690425, 175.4381630812001731 ) ) ;
#105597=EDGE_CURVE ( 'NONE', #106841, #29992, #7111, .T. ) ;
#105605=ORIENTED_EDGE ( 'NONE', *, *, #92098, .T. ) ;
#105618=AXIS2_PLACEMENT_3D ( 'NONE', #44250, #95741, #53206 ) ;
#105620=CARTESIAN_POINT ( 'NONE',  ( 22.08327125186925599, 1523.604703353109699, 184.4267662568470598 ) ) ;
#105625=DIRECTION ( 'NONE',  ( -0.8090169943749548898, -0.000000000000000000, -0.5877852522924631451 ) ) ;
#105627=CARTESIAN_POINT ( 'NONE',  ( 21.84020450222056908, 1523.481610426287716, 234.9798068779740277 ) ) ;
#105628=EDGE_CURVE ( 'NONE', #63483, #69179, #77795, .T. ) ;
#105636=ADVANCED_FACE ( 'NONE', ( #39229 ), #35729, .T. ) ;
#105637=CARTESIAN_POINT ( 'NONE',  ( 16.66936639845631518, 1523.382868172864164, 180.4828114240739296 ) ) ;
#105639=CARTESIAN_POINT ( 'NONE',  ( 19.53786426059019021, 1512.187213306747481, 179.5239794925693388 ) ) ;
#105643=EDGE_LOOP ( 'NONE', ( #1362, #92883, #22072, #24143 ) ) ;
#105647=EDGE_CURVE ( 'NONE', #32282, #13288, #5272, .T. ) ;
#105651=FACE_OUTER_BOUND ( 'NONE', #21563, .T. ) ;
#105654=DIRECTION ( 'NONE',  ( -0.9948834766775036531, 1.294385792140559950E-15, -0.1010290445074239624 ) ) ;
#105697=DIRECTION ( 'NONE',  ( -0.000000000000000000, -1.000000000000000000, -0.000000000000000000 ) ) ;
#105709=CARTESIAN_POINT ( 'NONE',  ( -0.5890887500919903541, 1526.382868172863937, 243.2762031678882977 ) ) ;
#105714=CARTESIAN_POINT ( 'NONE',  ( -2.664386649677787045, 1523.844782250835124, 176.1122499388616234 ) ) ;
#105724=CARTESIAN_POINT ( 'NONE',  ( 0.000000000000000000, 1518.913060387330006, 209.1218459616979999 ) ) ;
#105727=VERTEX_POINT ( 'NONE', #103395 ) ;
#105739=EDGE_LOOP ( 'NONE', ( #43710, #53464, #35443, #6675 ) ) ;
#105742=ORIENTED_EDGE ( 'NONE', *, *, #4401, .F. ) ;
#105756=CARTESIAN_POINT ( 'NONE',  ( 3.302453616664800418, 1524.523992613103019, 241.8698019156646239 ) ) ;
#105760=CARTESIAN_POINT ( 'NONE',  ( 19.63708787179898962, 1526.382868172863937, 234.8228066531187324 ) ) ;
#105772=CARTESIAN_POINT ( 'NONE',  ( -32.16776790210110448, 1524.538969332612623, 202.1449104801618262 ) ) ;
#105779=CIRCLE ( 'NONE', #19990, 1.999999999999998668 ) ;
#105783=CARTESIAN_POINT ( 'NONE',  ( -16.83198307403168315, 1526.000688113731940, 235.9162354437811473 ) ) ;
#105788=CARTESIAN_POINT ( 'NONE',  ( 0.000000000000000000, 1512.187213306747481, 209.1218459616979999 ) ) ;
#105808=DIRECTION ( 'NONE',  ( 0.000000000000000000, 0.000000000000000000, 1.000000000000000000 ) ) ;
#105810=EDGE_CURVE ( 'NONE', #23280, #17035, #22987, .T. ) ;
#105816=ORIENTED_EDGE ( 'NONE', *, *, #84859, .F. ) ;
#105817=ADVANCED_FACE ( 'NONE', ( #107011 ), #110777, .T. ) ;
#105821=CARTESIAN_POINT ( 'NONE',  ( -29.78220350812331318, 1524.382868172863937, 221.7347658002330775 ) ) ;
#105823=CARTESIAN_POINT ( 'NONE',  ( 30.90487439922552682, 1525.907212628473644, 201.8101144455178257 ) ) ;
#105833=CARTESIAN_POINT ( 'NONE',  ( 33.28034951413926734, 1522.862737210650039, 200.8029765415138286 ) ) ;
#105834=ORIENTED_EDGE ( 'NONE', *, *, #68911, .T. ) ;
#105849=ORIENTED_EDGE ( 'NONE', *, *, #63675, .F. ) ;
#105871=CARTESIAN_POINT ( 'NONE',  ( -29.82178186784418727, 1526.306647125542440, 216.9179131060151633 ) ) ;
#105877=CARTESIAN_POINT ( 'NONE',  ( 19.53786426059019021, 1512.187213306747481, 181.5239794925693388 ) ) ;
#105887=CIRCLE ( 'NONE', #7557, 1.000000000000000000 ) ;
#105892=DIRECTION ( 'NONE',  ( 0.000000000000000000, 0.000000000000000000, 1.000000000000000000 ) ) ;
#105899=DIRECTION ( 'NONE',  ( 0.000000000000000000, 0.000000000000000000, 1.000000000000000000 ) ) ;
#105909=CARTESIAN_POINT ( 'NONE',  ( -21.33281718256813875, 1523.429859730331145, 237.7590525783452335 ) ) ;
#105916=EDGE_CURVE ( 'NONE', #27462, #41473, #42851, .T. ) ;
#105919=CYLINDRICAL_SURFACE ( 'NONE', #78097, 33.13701971169416538 ) ;
#105929=DIRECTION ( 'NONE',  ( 0.000000000000000000, 0.000000000000000000, 1.000000000000000000 ) ) ;
#105938=CARTESIAN_POINT ( 'NONE',  ( -30.11857922865454640, 1525.055427061272439, 196.5532548484356141 ) ) ;
#105939=LINE ( 'NONE', #3488, #104959 ) ;
#105960=LINE ( 'NONE', #81825, #21759 ) ;
#105963=LINE ( 'NONE', #29241, #41897 ) ;
#105973=ORIENTED_EDGE ( 'NONE', *, *, #48403, .T. ) ;
#105989=DIRECTION ( 'NONE',  ( -0.000000000000000000, -1.000000000000000000, -0.000000000000000000 ) ) ;
#105990=VERTEX_POINT ( 'NONE', #6204 ) ;
#106006=( BOUNDED_SURFACE ( )  B_SPLINE_SURFACE ( 3, 2, ( 
 ( #56459, #49718, #109073 ),
 ( #65981, #22259, #4934 ),
 ( #39078, #57023, #90593 ),
 ( #41306, #30692, #39651 ) ),
 .UNSPECIFIED., .F., .F., .F. ) 
 B_SPLINE_SURFACE_WITH_KNOTS ( ( 4, 4 ),
 ( 3, 3 ),
 ( 0.000000000000000000, 0.0002960034161023847852 ),
 ( 0.000000000000000000, 1.000000000000000000 ),
 .UNSPECIFIED. ) 
 GEOMETRIC_REPRESENTATION_ITEM ( )  RATIONAL_B_SPLINE_SURFACE ( (
 ( 1.000000000000000000, 0.8070209408750051994, 1.000000000000000000),
 ( 1.000000000000000000, 0.8071723757218238759, 1.000000000000000000),
 ( 1.000000000000000000, 0.8072480346917746408, 1.000000000000000000),
 ( 1.000000000000000000, 0.8072480644198114508, 1.000000000000000000) ) ) 
 REPRESENTATION_ITEM ( '' )  SURFACE ( )  );
#106053=CARTESIAN_POINT ( 'NONE',  ( -21.41971086555066606, 1511.187213306747708, 233.0798096144383749 ) ) ;
#106054=CARTESIAN_POINT ( 'NONE',  ( -22.07691437628720266, 1523.843263703804041, 184.4448114610363518 ) ) ;
#106107=CARTESIAN_POINT ( 'NONE',  ( -16.50400130224782558, 1525.907212628473644, 181.9890130758379598 ) ) ;
#106111=CARTESIAN_POINT ( 'NONE',  ( 19.53786426059039982, 1511.187213306747708, 237.7197124308265188 ) ) ;
#106129=CARTESIAN_POINT ( 'NONE',  ( -29.86461515634926656, 1525.960063244517187, 197.2746849027940925 ) ) ;
#106133=CARTESIAN_POINT ( 'NONE',  ( 20.21023357682329546, 1526.107880201381477, 233.6897414230651293 ) ) ;
#106143=ORIENTED_EDGE ( 'NONE', *, *, #84265, .F. ) ;
#106165=EDGE_LOOP ( 'NONE', ( #23455, #101203, #53272, #104006, #108228, #5319, #96257, #8130 ) ) ;
#106178=CARTESIAN_POINT ( 'NONE',  ( 2.383407846124329765, 1522.906363951597314, 243.2919566057095153 ) ) ;
#106218=CARTESIAN_POINT ( 'NONE',  ( 34.09113935470853818, 1523.429859730330008, 198.4929744671651974 ) ) ;
#106220=VERTEX_POINT ( 'NONE', #55947 ) ;
#106231=CARTESIAN_POINT ( 'NONE',  ( -30.04349656869200302, 1524.760046179776054, 222.3147819414557489 ) ) ;
#106235=ORIENTED_EDGE ( 'NONE', *, *, #8949, .F. ) ;
#106244=CIRCLE ( 'NONE', #52545, 2.000000000000004441 ) ;
#106249=EDGE_CURVE ( 'NONE', #21883, #91721, #16036, .T. ) ;
#106258=EDGE_LOOP ( 'NONE', ( #75904, #49888, #46508, #3527 ) ) ;
#106278=DIRECTION ( 'NONE',  ( 0.5877852522924673639, 0.000000000000000000, -0.8090169943749514481 ) ) ;
#106294=B_SPLINE_CURVE_WITH_KNOTS ( 'NONE', 3,
 ( #63774, #30695, #46973, #80561, #71087, #3876, #105772, #81095, #97890, #98988 ),
 .UNSPECIFIED., .F., .F.,
 ( 4, 2, 2, 2, 4 ),
 ( 0.000000000000000000, 0.0007189769279725866536, 0.001437953855945173307, 0.002156930783917760178, 0.002875907711890346614 ),
 .UNSPECIFIED. ) ;
#106295=FACE_OUTER_BOUND ( 'NONE', #94051, .T. ) ;
#106298=DIRECTION ( 'NONE',  ( 0.000000000000000000, 1.000000000000000000, 0.000000000000000000 ) ) ;
#106299=CARTESIAN_POINT ( 'NONE',  ( -22.03465957474591619, 1512.187213306747481, 182.8300405912331144 ) ) ;
#106307=CIRCLE ( 'NONE', #2676, 1.000000000000000888 ) ;
#106310=CARTESIAN_POINT ( 'NONE',  ( -1.912903644472999432, 1526.104292489133059, 240.8844628569841575 ) ) ;
#106312=AXIS2_PLACEMENT_3D ( 'NONE', #38801, #88682, #79732 ) ;
#106313=AXIS2_PLACEMENT_3D ( 'NONE', #39287, #21902, #64519 ) ;
#106320=CARTESIAN_POINT ( 'NONE',  ( 173.8335085727406693, 1526.382868172863937, 317.3879012941853830 ) ) ;
#106328=CARTESIAN_POINT ( 'NONE',  ( -31.30542570072097064, 1525.651285554137075, 216.2805821473968422 ) ) ;
#106348=CIRCLE ( 'NONE', #58090, 30.13701971169416183 ) ;
#106365=DIRECTION ( 'NONE',  ( 0.000000000000000000, 1.000000000000000000, 0.000000000000000000 ) ) ;
#106376=ADVANCED_FACE ( 'NONE', ( #87772 ), #35138, .T. ) ;
#106379=ORIENTED_EDGE ( 'NONE', *, *, #23299, .T. ) ;
#106394=EDGE_CURVE ( 'NONE', #32555, #105138, #54730, .T. ) ;
#106396=CARTESIAN_POINT ( 'NONE',  ( 16.56816485274985951, 1526.186458717543701, 235.6095862221665129 ) ) ;
#106407=EDGE_LOOP ( 'NONE', ( #68978, #75446, #54017, #59164 ) ) ;
#106409=CARTESIAN_POINT ( 'NONE',  ( -32.28466283162165240, 1512.187213306747481, 199.0684425896249081 ) ) ;
#106443=CARTESIAN_POINT ( 'NONE',  ( 32.85805783624304155, 1523.678648413191695, 201.0453875934054508 ) ) ;
#106458=CARTESIAN_POINT ( 'NONE',  ( 18.72690275718901987, 1526.278758871497985, 182.1127646906432744 ) ) ;
#106468=DIRECTION ( 'NONE',  ( 0.5117323852940846018, 0.8591449038673432126, 0.000000000000000000 ) ) ;
#106471=CARTESIAN_POINT ( 'NONE',  ( -16.66231036550682276, 1523.604703353109699, 237.7554842931448036 ) ) ;
#106478=CARTESIAN_POINT ( 'NONE',  ( -3.347801439296141712, 1523.382868172864164, 176.1543725841967500 ) ) ;
#106480=ORIENTED_EDGE ( 'NONE', *, *, #21508, .F. ) ;
#106484=DIRECTION ( 'NONE',  ( 0.000000000000000000, 0.000000000000000000, -1.000000000000000000 ) ) ;
#106487=CARTESIAN_POINT ( 'NONE',  ( -31.34137657934000387, 1501.977400791986611, 221.9025654077414345 ) ) ;
#106490=DIRECTION ( 'NONE',  ( 0.9125304618754029873, 0.000000000000000000, 0.4090087482554177756 ) ) ;
#106508=EDGE_LOOP ( 'NONE', ( #63816, #74349, #2039, #55431, #101972 ) ) ;
#106509=FACE_OUTER_BOUND ( 'NONE', #498, .T. ) ;
#106519=EDGE_CURVE ( 'NONE', #91721, #43187, #91192, .T. ) ;
#106522=AXIS2_PLACEMENT_3D ( 'NONE', #45830, #79963, #35195 ) ;
#106528=ORIENTED_EDGE ( 'NONE', *, *, #86399, .F. ) ;
#106529=VERTEX_POINT ( 'NONE', #25208 ) ;
#106541=EDGE_LOOP ( 'NONE', ( #51731, #71959, #45276, #53700 ) ) ;
#106555=B_SPLINE_CURVE_WITH_KNOTS ( 'NONE', 3,
 ( #65058, #4059, #79664, #38185, #56654, #55563, #81828, #13512 ),
 .UNSPECIFIED., .F., .F.,
 ( 4, 2, 2, 4 ),
 ( 0.000000000000000000, 0.001073044933456205339, 0.001609567400184348232, 0.002146089866912491342 ),
 .UNSPECIFIED. ) ;
#106567=ADVANCED_FACE ( 'NONE', ( #94080 ), #49899, .T. ) ;
#106568=DIRECTION ( 'NONE',  ( -0.000000000000000000, -1.000000000000000000, -0.000000000000000000 ) ) ;
#106570=ORIENTED_EDGE ( 'NONE', *, *, #4657, .T. ) ;
#106604=CARTESIAN_POINT ( 'NONE',  ( 32.22536377336281532, 1523.621879633029039, 216.8351145222429466 ) ) ;
#106627=ORIENTED_EDGE ( 'NONE', *, *, #863, .T. ) ;
#106645=CARTESIAN_POINT ( 'NONE',  ( 20.49599333844858151, 1525.960063244517187, 233.8638087104923216 ) ) ;
#106651=FACE_OUTER_BOUND ( 'NONE', #55936, .T. ) ;
#106654=COLOUR_RGB ( '', 0.31764706, 0.68627451, 0.89019608) ;
#106687=DIRECTION ( 'NONE',  ( -0.3090169943749382919, 0.000000000000000000, 0.9510565162951565288 ) ) ;
#106690=CARTESIAN_POINT ( 'NONE',  ( -32.97913964219446115, 1511.187213306747708, 197.9697544589750464 ) ) ;
#106694=CARTESIAN_POINT ( 'NONE',  ( 21.54116136312511998, 1523.382868172863709, 183.9310736446955445 ) ) ;
#106697=EDGE_LOOP ( 'NONE', ( #75293, #54686, #16191, #42908 ) ) ;
#106715=CARTESIAN_POINT ( 'NONE',  ( 0.4151546846839010985, 1522.906561336850928, 244.9330574173806951 ) ) ;
#106723=CARTESIAN_POINT ( 'NONE',  ( -2.570812331889315683, 1525.317349363550647, 241.4588417251712826 ) ) ;
#106734=ORIENTED_EDGE ( 'NONE', *, *, #67197, .F. ) ;
#106735=CARTESIAN_POINT ( 'NONE',  ( 29.99620953741488449, 1526.382868172863937, 198.4974435154498735 ) ) ;
#106740=EDGE_CURVE ( 'NONE', #44756, #237, #67967, .T. ) ;
#106741=CARTESIAN_POINT ( 'NONE',  ( 204.2714532754875449, 1524.382868172863937, 223.7095399770875304 ) ) ;
#106752=CARTESIAN_POINT ( 'NONE',  ( -2.372478608334043670, 1522.644714754858114, 243.3440112565160973 ) ) ;
#106757=CARTESIAN_POINT ( 'NONE',  ( 31.95643112691193366, 1526.329757971585877, 201.5629546934984262 ) ) ;
#106788=ADVANCED_FACE ( 'NONE', ( #13924 ), #48111, .T. ) ;
#106795=EDGE_LOOP ( 'NONE', ( #76542, #46994, #4217, #99350, #102651 ) ) ;
#106812=ORIENTED_EDGE ( 'NONE', *, *, #46140, .F. ) ;
#106820=DIRECTION ( 'NONE',  ( 0.000000000000000000, 0.000000000000000000, -1.000000000000000000 ) ) ;
#106821=CARTESIAN_POINT ( 'NONE',  ( 30.61443310214658453, 1523.462669333492840, 221.8243310972552536 ) ) ;
#106823=ADVANCED_FACE ( 'NONE', ( #64921 ), #82249, .T. ) ;
#106827=ORIENTED_EDGE ( 'NONE', *, *, #83746, .T. ) ;
#106841=VERTEX_POINT ( 'NONE', #6092 ) ;
#106844=DIRECTION ( 'NONE',  ( 0.000000000000000000, 0.000000000000000000, -1.000000000000000000 ) ) ;
#106848=AXIS2_PLACEMENT_3D ( 'NONE', #2119, #68767, #27290 ) ;
#106849=CARTESIAN_POINT ( 'NONE',  ( -16.73628186595804479, 1526.382868172864164, 234.1845039693045862 ) ) ;
#106857=EDGE_CURVE ( 'NONE', #53391, #79801, #84074, .T. ) ;
#106867=ORIENTED_EDGE ( 'NONE', *, *, #28546, .T. ) ;
#106873=ADVANCED_FACE ( 'NONE', ( #52529 ), #69340, .T. ) ;
#106875=CARTESIAN_POINT ( 'NONE',  ( 2.470168522032202940, 1523.481610118012441, 242.8787258960491897 ) ) ;
#106885=CARTESIAN_POINT ( 'NONE',  ( 19.33418355719911474, 1523.342713519622976, 239.2327152390723484 ) ) ;
#106898=DIRECTION ( 'NONE',  ( 0.000000000000000000, 1.000000000000000000, 0.000000000000000000 ) ) ;
#106908=EDGE_CURVE ( 'NONE', #43261, #107214, #50050, .T. ) ;
#106923=ORIENTED_EDGE ( 'NONE', *, *, #77087, .T. ) ;
#106925=CIRCLE ( 'NONE', #96152, 0.9999999999999976685 ) ;
#106935=CARTESIAN_POINT ( 'NONE',  ( 16.69297358003969123, 1526.382868172864164, 234.5473741529541201 ) ) ;
#106947=ORIENTED_EDGE ( 'NONE', *, *, #51184, .T. ) ;
#106951=CARTESIAN_POINT ( 'NONE',  ( -30.30078187369513643, 1526.189899547014875, 216.6986553323659166 ) ) ;
#106960=CARTESIAN_POINT ( 'NONE',  ( 30.00906687500045322, 1525.856064936156145, 197.1249949705187419 ) ) ;
#106977=ADVANCED_FACE ( 'NONE', ( #98918 ), #83065, .F. ) ;
#106995=EDGE_CURVE ( 'NONE', #82569, #29284, #50727, .T. ) ;
#107011=FACE_OUTER_BOUND ( 'NONE', #81656, .T. ) ;
#107015=AXIS2_PLACEMENT_3D ( 'NONE', #51970, #51406, #78260 ) ;
#107017=CARTESIAN_POINT ( 'NONE',  ( 18.66420869458052323, 1526.382868172864164, 232.7837831374276902 ) ) ;
#107024=CARTESIAN_POINT ( 'NONE',  ( 16.69366550187172038, 1526.382868172863937, 183.7020206129021176 ) ) ;
#107026=FACE_OUTER_BOUND ( 'NONE', #69107, .T. ) ;
#107030=AXIS2_PLACEMENT_3D ( 'NONE', #50633, #84765, #8062 ) ;
#107044=EDGE_CURVE ( 'NONE', #24484, #95178, #46543, .T. ) ;
#107075=VERTEX_POINT ( 'NONE', #27732 ) ;
#107103=CARTESIAN_POINT ( 'NONE',  ( -21.92916355573733966, 1523.390106123591067, 183.0654104491212877 ) ) ;
#107107=CIRCLE ( 'NONE', #82076, 0.9999999999999765743 ) ;
#107108=CARTESIAN_POINT ( 'NONE',  ( -18.19590854888121356, 1501.977400791986611, 238.2026672068777202 ) ) ;
#107117=CARTESIAN_POINT ( 'NONE',  ( -1.191524307911313585, 1526.382868172864164, 179.0083900503168479 ) ) ;
#107122=CARTESIAN_POINT ( 'NONE',  ( -31.32995031131208918, 1523.678648413191695, 196.3423562208917872 ) ) ;
#107133=CARTESIAN_POINT ( 'NONE',  ( 0.000000000000000000, 1512.187213306747481, 209.1218459616979999 ) ) ;
#107140=ADVANCED_FACE ( 'NONE', ( #104439 ), #78823, .F. ) ;
#107150=DIRECTION ( 'NONE',  ( 0.4090087482554177756, 0.000000000000000000, -0.9125304618754029873 ) ) ;
#107155=ADVANCED_FACE ( 'NONE', ( #4730 ), #75874, .F. ) ;
#107158=CARTESIAN_POINT ( 'NONE',  ( -19.30300490007812186, 1526.348417187222594, 185.0858834514397984 ) ) ;
#107180=TOROIDAL_SURFACE ( 'NONE', #3558, 24.69926344187880929, 1.000000000000000000 ) ;
#107194=EDGE_CURVE ( 'NONE', #29531, #66077, #82241, .T. ) ;
#107195=CARTESIAN_POINT ( 'NONE',  ( -31.33756686635658184, 1523.580204110583963, 196.3415365203911449 ) ) ;
#107200=CARTESIAN_POINT ( 'NONE',  ( 31.12456774391174719, 1525.960063244516959, 201.1524202391562710 ) ) ;
#107205=CARTESIAN_POINT ( 'NONE',  ( 22.08622291482331335, 1523.382868172864164, 184.4183880513174927 ) ) ;
#107214=VERTEX_POINT ( 'NONE', #36557 ) ;
#107221=AXIS2_PLACEMENT_3D ( 'NONE', #24261, #66855, #84720 ) ;
#107235=CARTESIAN_POINT ( 'NONE',  ( 29.86461515634913866, 1525.960063244516959, 197.2746849027935809 ) ) ;
#107262=( BOUNDED_SURFACE ( )  B_SPLINE_SURFACE ( 3, 2, ( 
 ( #107235, #49007, #6437 ),
 ( #65802, #99923, #29969 ),
 ( #82024, #30526, #98279 ),
 ( #31075, #5886, #49556 ),
 ( #65258, #21555, #13151 ),
 ( #38914, #73096, #64718 ) ),
 .UNSPECIFIED., .F., .F., .F. ) 
 B_SPLINE_SURFACE_WITH_KNOTS ( ( 4, 2, 4 ),
 ( 3, 3 ),
 ( -2.493664996716660198E-17, 0.001312027981647308043, 0.002624055963294641240 ),
 ( 0.000000000000000000, 1.000000000000000000 ),
 .UNSPECIFIED. ) 
 GEOMETRIC_REPRESENTATION_ITEM ( )  RATIONAL_B_SPLINE_SURFACE ( (
 ( 1.000000000000000000, 0.9376006582765884501, 1.000000000000000000),
 ( 1.000000000000000000, 0.9569320108029427674, 1.000000000000000000),
 ( 1.000000000000000000, 0.9725743441609863149, 1.000000000000000000),
 ( 1.000000000000000000, 0.9942095667144646987, 1.000000000000000000),
 ( 1.000000000000000000, 1.000043666450031843, 1.000000000000000000),
 ( 1.000000000000000000, 1.000000000000000000, 1.000000000000000000) ) ) 
 REPRESENTATION_ITEM ( '' )  SURFACE ( )  );
#107274=DIRECTION ( 'NONE',  ( 0.000000000000000000, 1.000000000000000000, 0.000000000000000000 ) ) ;
#107283=CARTESIAN_POINT ( 'NONE',  ( -2.700443415721282658, 1524.678872986499073, 241.8612037782705784 ) ) ;
#107296=DIRECTION ( 'NONE',  ( 0.000000000000000000, 1.000000000000000000, 0.000000000000000000 ) ) ;
#107316=CARTESIAN_POINT ( 'NONE',  ( 33.52308185467321522, 1525.402221411319715, 200.6636391946808828 ) ) ;
#107325=DIRECTION ( 'NONE',  ( 0.9125304618753908859, 0.000000000000000000, -0.4090087482554448095 ) ) ;
#107326=AXIS2_PLACEMENT_3D ( 'NONE', #31653, #65833, #13179 ) ;
#107333=AXIS2_PLACEMENT_3D ( 'NONE', #57501, #12717, #107325 ) ;
#107343=AXIS2_PLACEMENT_3D ( 'NONE', #52418, #96053, #20428 ) ;
#107369=ORIENTED_EDGE ( 'NONE', *, *, #32296, .T. ) ;
#107371=DIRECTION ( 'NONE',  ( 0.000000000000000000, 0.000000000000000000, 1.000000000000000000 ) ) ;
#107391=CARTESIAN_POINT ( 'NONE',  ( -0.8350686643532192477, 1526.382868172863937, 177.3106345060153046 ) ) ;
#107400=EDGE_LOOP ( 'NONE', ( #83510, #11087, #68101, #80127 ) ) ;
#107401=ORIENTED_EDGE ( 'NONE', *, *, #80874, .F. ) ;
#107405=DIRECTION ( 'NONE',  ( -0.3090169943749446757, 0.000000000000000000, 0.9510565162951544194 ) ) ;
#107406=AXIS2_PLACEMENT_3D ( 'NONE', #106409, #31344, #29693 ) ;
#107414=CARTESIAN_POINT ( 'NONE',  ( 32.31946296792703066, 1524.082582765195411, 216.0996188568618948 ) ) ;
#107423=VECTOR ( 'NONE', #28356, 1000.000000000000000 ) ;
#107437=ORIENTED_EDGE ( 'NONE', *, *, #98607, .T. ) ;
#107439=ORIENTED_EDGE ( 'NONE', *, *, #61737, .F. ) ;
#107440=LINE ( 'NONE', #90638, #58294 ) ;
#107445=CARTESIAN_POINT ( 'NONE',  ( -33.93019615848938031, 1522.382868172863937, 220.5829544587965927 ) ) ;
#107467=CARTESIAN_POINT ( 'NONE',  ( -17.17241001986462123, 1523.382868172864164, 237.6251415217917895 ) ) ;
#107472=CARTESIAN_POINT ( 'NONE',  ( 17.30126322264623084, 1523.462669333488975, 237.3930845918952741 ) ) ;
#107488=EDGE_CURVE ( 'NONE', #36910, #109511, #60852, .T. ) ;
#107515=CIRCLE ( 'NONE', #41346, 1.000000000000001332 ) ;
#107542=DIRECTION ( 'NONE',  ( 0.000000000000000000, 1.000000000000000000, 0.000000000000000000 ) ) ;
#107554=B_SPLINE_CURVE_WITH_KNOTS ( 'NONE', 3,
 ( #22788, #41278, #23360, #58093, #65950, #24451 ),
 .UNSPECIFIED., .F., .F.,
 ( 4, 2, 4 ),
 ( -1.285435071114701246E-05, 0.001079388306740486445, 0.002171630964192120157 ),
 .UNSPECIFIED. ) ;
#107560=CARTESIAN_POINT ( 'NONE',  ( -16.54281257266368144, 1524.843416604514232, 180.8453930184409160 ) ) ;
#107593=CARTESIAN_POINT ( 'NONE',  ( 17.84054676580441168, 1523.580203803270933, 237.8810931560534243 ) ) ;
#107597=AXIS2_PLACEMENT_3D ( 'NONE', #8963, #59397, #93508 ) ;
#107601=DIRECTION ( 'NONE',  ( 0.000000000000000000, 1.000000000000000000, 0.000000000000000000 ) ) ;
#107624=ORIENTED_EDGE ( 'NONE', *, *, #76153, .F. ) ;
#107626=CARTESIAN_POINT ( 'NONE',  ( -17.12015143466543066, 1526.107880201381477, 235.9348175143726394 ) ) ;
#107628=ORIENTED_EDGE ( 'NONE', *, *, #103447, .F. ) ;
#107635=FACE_OUTER_BOUND ( 'NONE', #97365, .T. ) ;
#107639=CARTESIAN_POINT ( 'NONE',  ( 30.29107669316897855, 1523.847248782568613, 222.4926083572483151 ) ) ;
#107642=ORIENTED_EDGE ( 'NONE', *, *, #63868, .F. ) ;
#107655=CARTESIAN_POINT ( 'NONE',  ( -22.08622291482314282, 1512.187213306747481, 233.8253038720786776 ) ) ;
#107674=CARTESIAN_POINT ( 'NONE',  ( -2.596261494520234248, 1525.907212628473644, 177.4701144822248011 ) ) ;
#107677=DIRECTION ( 'NONE',  ( 0.000000000000000000, -1.000000000000000000, 0.000000000000000000 ) ) ;
#107686=ORIENTED_EDGE ( 'NONE', *, *, #51811, .F. ) ;
#107690=DIRECTION ( 'NONE',  ( 0.000000000000000000, 0.000000000000000000, 1.000000000000000000 ) ) ;
#107695=AXIS2_PLACEMENT_3D ( 'NONE', #53174, #10611, #71098 ) ;
#107703=CARTESIAN_POINT ( 'NONE',  ( 22.69876404240098111, 1501.977400791986611, 236.8953202675778016 ) ) ;
#107708=CARTESIAN_POINT ( 'NONE',  ( -20.71343476517491311, 1512.187213306747481, 238.3377464195766890 ) ) ;
#107711=VECTOR ( 'NONE', #25560, 1000.000000000000000 ) ;
#107714=FACE_OUTER_BOUND ( 'NONE', #60414, .T. ) ;
#107719=CARTESIAN_POINT ( 'NONE',  ( 31.81407709660768646, 1522.862737210649811, 196.2902540610627682 ) ) ;
#107725=CARTESIAN_POINT ( 'NONE',  ( 17.34064885126017685, 1525.506916460683669, 236.9219916297327018 ) ) ;
#107737=ORIENTED_EDGE ( 'NONE', *, *, #58534, .F. ) ;
#107750=PRESENTATION_STYLE_ASSIGNMENT (( #99880 ) ) ;
#107756=CARTESIAN_POINT ( 'NONE',  ( -16.73628186595857059, 1526.382868172864164, 184.0591879540917546 ) ) ;
#107757=CARTESIAN_POINT ( 'NONE',  ( 21.92050665148286370, 1524.523992613103701, 233.6743653272424979 ) ) ;
#107763=CARTESIAN_POINT ( 'NONE',  ( -29.36670733769854991, 1526.000688113720798, 197.3383209345158491 ) ) ;
#107772=ORIENTED_EDGE ( 'NONE', *, *, #32373, .T. ) ;
#107775=EDGE_CURVE ( 'NONE', #41473, #35962, #76983, .T. ) ;
#107810=ORIENTED_EDGE ( 'NONE', *, *, #103447, .T. ) ;
#107815=CARTESIAN_POINT ( 'NONE',  ( 3.246772394788723481, 1512.187213306747481, 241.0944358625217774 ) ) ;
#107831=CARTESIAN_POINT ( 'NONE',  ( 3.347801439296144377, 1523.456872492435195, 242.0893193391992497 ) ) ;
#107832=CARTESIAN_POINT ( 'NONE',  ( 31.93052144186282604, 1525.394057003702756, 201.2251853851623196 ) ) ;
#107864=ORIENTED_EDGE ( 'NONE', *, *, #73570, .T. ) ;
#107880=CYLINDRICAL_SURFACE ( 'NONE', #82391, 30.10786454236638576 ) ;
#107898=CARTESIAN_POINT ( 'NONE',  ( -16.66701395081548398, 1523.530870145312292, 180.4846106723514083 ) ) ;
#107907=DIRECTION ( 'NONE',  ( -0.000000000000000000, -1.000000000000000000, -0.000000000000000000 ) ) ;
#107912=ADVANCED_FACE ( 'NONE', ( #5806 ), #98191, .T. ) ;
#107915=( BOUNDED_SURFACE ( )  B_SPLINE_SURFACE ( 3, 2, ( 
 ( #87751, #18847, #53043 ),
 ( #35668, #69855, #110721 ),
 ( #51931, #77138, #53608 ),
 ( #35115, #77677, #27828 ),
 ( #17172, #11033, #45200 ),
 ( #68205, #19404, #93905 ) ),
 .UNSPECIFIED., .F., .F., .F. ) 
 B_SPLINE_SURFACE_WITH_KNOTS ( ( 4, 2, 4 ),
 ( 3, 3 ),
 ( 3.469446951953614189E-18, 0.001312027981647208297, 0.002624055963294413124 ),
 ( 0.000000000000000000, 1.000000000000000000 ),
 .UNSPECIFIED. ) 
 GEOMETRIC_REPRESENTATION_ITEM ( )  RATIONAL_B_SPLINE_SURFACE ( (
 ( 1.000000000000000000, 0.9376006582765969988, 1.000000000000000000),
 ( 1.000000000000000000, 0.9569320108030995309, 1.000000000000000000),
 ( 1.000000000000000000, 0.9725743441607752615, 1.000000000000000000),
 ( 1.000000000000000000, 0.9942095667146912952, 1.000000000000000000),
 ( 1.000000000000000000, 1.000043666449861757, 1.000000000000000000),
 ( 1.000000000000000000, 1.000000000000000000, 1.000000000000000000) ) ) 
 REPRESENTATION_ITEM ( '' )  SURFACE ( )  );
#107925=LINE ( 'NONE', #41281, #44863 ) ;
#107953=ORIENTED_EDGE ( 'NONE', *, *, #46375, .T. ) ;
#107967=CARTESIAN_POINT ( 'NONE',  ( -32.38845791999490586, 1523.382868172864164, 216.1254071228449902 ) ) ;
#107972=DIRECTION ( 'NONE',  ( -0.8672669759446666182, 0.000000000000000000, -0.4978433412588672557 ) ) ;
#107975=ORIENTED_EDGE ( 'NONE', *, *, #100730, .T. ) ;
#107988=CIRCLE ( 'NONE', #70468, 24.69926344187880929 ) ;
#107996=CARTESIAN_POINT ( 'NONE',  ( -32.02808312589930040, 1511.187213306747708, 198.2787714533499752 ) ) ;
#108002=CARTESIAN_POINT ( 'NONE',  ( 3.059311260596259352, 1525.343710797494396, 176.8478414008731932 ) ) ;
#108006=CARTESIAN_POINT ( 'NONE',  ( 29.71163624023410321, 1526.333389947941441, 201.1407003069334678 ) ) ;
#108007=CIRCLE ( 'NONE', #68721, 0.9999999999999880096 ) ;
#108010=ORIENTED_EDGE ( 'NONE', *, *, #95558, .F. ) ;
#108014=CARTESIAN_POINT ( 'NONE',  ( -21.84020450222076448, 1523.382868172864164, 183.2638850454220858 ) ) ;
#108020=ORIENTED_EDGE ( 'NONE', *, *, #67878, .F. ) ;
#108025=ORIENTED_EDGE ( 'NONE', *, *, #92498, .F. ) ;
#108033=CARTESIAN_POINT ( 'NONE',  ( 16.75454338845089453, 1526.382868172571079, 234.5462402641960864 ) ) ;
#108057=CARTESIAN_POINT ( 'NONE',  ( 29.86283313086964597, 1525.137881624885267, 196.1139775505488956 ) ) ;
#108080=DIRECTION ( 'NONE',  ( 0.000000000000000000, 0.000000000000000000, -1.000000000000000000 ) ) ;
#108082=CARTESIAN_POINT ( 'NONE',  ( -22.41686883764721827, 1524.667648926078527, 236.2663900491539266 ) ) ;
#108085=CARTESIAN_POINT ( 'NONE',  ( 28.62143996450550176, 1526.335487865669620, 220.1875038795444937 ) ) ;
#108091=CARTESIAN_POINT ( 'NONE',  ( -0.4151546846821905778, 1522.382868172863937, 173.3106345060153046 ) ) ;
#108094=AXIS2_PLACEMENT_3D ( 'NONE', #8903, #50929, #85602 ) ;
#108102=VERTEX_POINT ( 'NONE', #44376 ) ;
#108103=CARTESIAN_POINT ( 'NONE',  ( -16.64711227028525897, 1523.843271061947462, 180.4998300114153267 ) ) ;
#108130=FACE_OUTER_BOUND ( 'NONE', #108151, .T. ) ;
#108146=CARTESIAN_POINT ( 'NONE',  ( -17.83486663330464950, 1523.678648413191695, 237.8759530894961074 ) ) ;
#108148=VECTOR ( 'NONE', #35966, 1000.000000000000114 ) ;
#108151=EDGE_LOOP ( 'NONE', ( #4185, #87645, #109529, #105816 ) ) ;
#108152=CARTESIAN_POINT ( 'NONE',  ( 22.74803453391442787, 1523.678648413191695, 183.6833808205261676 ) ) ;
#108161=DIRECTION ( 'NONE',  ( -0.000000000000000000, -1.000000000000000000, -0.000000000000000000 ) ) ;
#108165=DIRECTION ( 'NONE',  ( 0.9942586961433749204, -3.929125341476398997E-15, -0.1070030146457386366 ) ) ;
#108169=ORIENTED_EDGE ( 'NONE', *, *, #29514, .F. ) ;
#108178=CIRCLE ( 'NONE', #102799, 0.9999999999999976685 ) ;
#108180=CARTESIAN_POINT ( 'NONE',  ( 2.121003584631406813, 1512.187213306747481, 239.6750300321239138 ) ) ;
#108182=VERTEX_POINT ( 'NONE', #104266 ) ;
#108210=CARTESIAN_POINT ( 'NONE',  ( 31.26701299883995944, 1523.919943579690425, 221.8945623323605503 ) ) ;
#108228=ORIENTED_EDGE ( 'NONE', *, *, #80254, .F. ) ;
#108257=DIRECTION ( 'NONE',  ( 0.000000000000000000, 0.000000000000000000, 1.000000000000000000 ) ) ;
#108258=CARTESIAN_POINT ( 'NONE',  ( 32.48455292688698393, 1524.659148609483054, 217.0704923713155949 ) ) ;
#108269=DIRECTION ( 'NONE',  ( 0.8200914087127335605, -0.4884709562386523873, -0.2980708074717494660 ) ) ;
#108297=EDGE_CURVE ( 'NONE', #53518, #48271, #98099, .T. ) ;
#108349=CARTESIAN_POINT ( 'NONE',  ( -31.92108011125336375, 1511.187213306747708, 220.9591791661900686 ) ) ;
#108356=CIRCLE ( 'NONE', #108094, 1.999999999999995559 ) ;
#108365=CARTESIAN_POINT ( 'NONE',  ( 31.03088476499823045, 1523.982201850120191, 221.8691499995717606 ) ) ;
#108369=ORIENTED_EDGE ( 'NONE', *, *, #105916, .T. ) ;
#108376=EDGE_CURVE ( 'NONE', #76626, #38078, #17954, .T. ) ;
#108382=B_SPLINE_CURVE_WITH_KNOTS ( 'NONE', 3,
 ( #98151, #46139, #28757, #104356, #37162, #62961, #45586, #88676, #45034, #21425 ),
 .UNSPECIFIED., .F., .F.,
 ( 4, 2, 2, 2, 4 ),
 ( 1.301042606982605321E-18, 0.0007406479101618187273, 0.001481295820323636154, 0.002221943730485453471, 0.002962591640647271006 ),
 .UNSPECIFIED. ) ;
#108389=CARTESIAN_POINT ( 'NONE',  ( -17.61566626013477332, 1524.599984580802357, 237.5963446818502973 ) ) ;
#108391=CARTESIAN_POINT ( 'NONE',  ( -32.38601544705593938, 1523.530935881284904, 202.1199691060090515 ) ) ;
#108393=CARTESIAN_POINT ( 'NONE',  ( 2.470168521978398868, 1501.977400791986611, 175.3649660270905315 ) ) ;
#108452=ORIENTED_EDGE ( 'NONE', *, *, #91858, .F. ) ;
#108458=CARTESIAN_POINT ( 'NONE',  ( -16.66231036550741607, 1523.604703353109699, 180.4882076302515372 ) ) ;
#108463=DIRECTION ( 'NONE',  ( -0.000000000000000000, -1.000000000000000000, -0.000000000000000000 ) ) ;
#108470=FACE_OUTER_BOUND ( 'NONE', #62210, .T. ) ;
#108480=B_SPLINE_CURVE_WITH_KNOTS ( 'NONE', 3,
 ( #8816, #461, #100135, #23420 ),
 .UNSPECIFIED., .F., .F.,
 ( 4, 4 ),
 ( 0.000000000000000000, 0.0002960034161023844057 ),
 .UNSPECIFIED. ) ;
#108489=CARTESIAN_POINT ( 'NONE',  ( 31.34137657907887231, 1523.481610118014260, 221.9025654077128991 ) ) ;
#108492=DIRECTION ( 'NONE',  ( 0.000000000000000000, 0.000000000000000000, 1.000000000000000000 ) ) ;
#108496=CARTESIAN_POINT ( 'NONE',  ( 0.000000000000000000, 1512.187213306747481, 209.1218459616979999 ) ) ;
#108507=FACE_OUTER_BOUND ( 'NONE', #76945, .T. ) ;
#108510=VERTEX_POINT ( 'NONE', #68668 ) ;
#108511=CYLINDRICAL_SURFACE ( 'NONE', #55111, 2.000000000000003109 ) ;
#108517=CARTESIAN_POINT ( 'NONE',  ( -16.75454338844117430, 1526.382868173645875, 234.5462402642023108 ) ) ;
#108526=CARTESIAN_POINT ( 'NONE',  ( 32.59719044532317866, 1523.982201850120191, 217.0485567930457762 ) ) ;
#108529=ADVANCED_FACE ( 'NONE', ( #60829 ), #76492, .T. ) ;
#108535=FACE_OUTER_BOUND ( 'NONE', #63507, .T. ) ;
#108544=CYLINDRICAL_SURFACE ( 'NONE', #80454, 2.000000000000000000 ) ;
#108548=ADVANCED_FACE ( 'NONE', ( #912, #59707 ), #69215, .F. ) ;
#108554=DIRECTION ( 'NONE',  ( -0.000000000000000000, -1.000000000000000000, -0.000000000000000000 ) ) ;
#108565=AXIS2_PLACEMENT_3D ( 'NONE', #30407, #98716, #5776 ) ;
#108566=CARTESIAN_POINT ( 'NONE',  ( -32.28466283162165240, 1501.977400791986611, 199.0684425896249081 ) ) ;
#108575=( BOUNDED_CURVE ( )  B_SPLINE_CURVE ( 3, ( #56455, #22256, #46967, #97342 ),
 .UNSPECIFIED., .F., .F. ) 
 B_SPLINE_CURVE_WITH_KNOTS ( ( 4, 4 ),
 ( 3.141592653589793116, 4.712388980384689674 ),
 .UNSPECIFIED. ) 
 CURVE ( )  GEOMETRIC_REPRESENTATION_ITEM ( )  RATIONAL_B_SPLINE_CURVE ( ( 1.000000000000000000, 0.8047378541243649375, 0.8047378541243649375, 1.000000000000000000 ) ) 
 REPRESENTATION_ITEM ( '' )  );
#108583=VERTEX_POINT ( 'NONE', #106111 ) ;
#108588=ORIENTED_EDGE ( 'NONE', *, *, #48069, .T. ) ;
#108589=EDGE_LOOP ( 'NONE', ( #82700, #68273, #31686, #39186 ) ) ;
#108592=VERTEX_POINT ( 'NONE', #88766 ) ;
#108618=CARTESIAN_POINT ( 'NONE',  ( 29.35073940689247962, 1526.211523310372058, 220.5206201286387113 ) ) ;
#108623=ORIENTED_EDGE ( 'NONE', *, *, #51793, .T. ) ;
#108639=CARTESIAN_POINT ( 'NONE',  ( -29.35747451427760168, 1526.382868173645875, 201.0438982057195290 ) ) ;
#108640=CARTESIAN_POINT ( 'NONE',  ( 17.83486663330488042, 1523.678648413191695, 180.3677388338999776 ) ) ;
#108646=AXIS2_PLACEMENT_3D ( 'NONE', #84681, #68467, #16356 ) ;
#108649=DIRECTION ( 'NONE',  ( -0.000000000000000000, -1.000000000000000000, -0.000000000000000000 ) ) ;
#108651=CARTESIAN_POINT ( 'NONE',  ( -2.372478608332517336, 1522.382868172863937, 174.8996806668726549 ) ) ;
#108674=CARTESIAN_POINT ( 'NONE',  ( -19.39983987835377732, 1522.382868172864164, 239.2921289694226061 ) ) ;
#108680=CARTESIAN_POINT ( 'NONE',  ( -21.83863730835998140, 1523.580203803270933, 234.9763103460708180 ) ) ;
#108687=ADVANCED_FACE ( 'NONE', ( #18223 ), #44777, .T. ) ;
#108692=DIRECTION ( 'NONE',  ( 0.000000000000000000, -1.000000000000000000, -0.000000000000000000 ) ) ;
#108696=CIRCLE ( 'NONE', #26437, 1.000000000000000888 ) ;
#108700=VERTEX_POINT ( 'NONE', #54635 ) ;
#108725=ORIENTED_EDGE ( 'NONE', *, *, #95558, .T. ) ;
#108737=CARTESIAN_POINT ( 'NONE',  ( 29.85692059557557343, 1525.159177407156221, 222.1259724534683073 ) ) ;
#108749=CARTESIAN_POINT ( 'NONE',  ( 21.10560967990464576, 1525.661276915132476, 233.3100090447210562 ) ) ;
#108759=AXIS2_PLACEMENT_3D ( 'NONE', #78819, #2133, #96165 ) ;
#108764=CARTESIAN_POINT ( 'NONE',  ( -21.95754362317823549, 1524.412928176730020, 233.6990317443709273 ) ) ;
#108770=CARTESIAN_POINT ( 'NONE',  ( -1.590879946460538319, 1526.333389948038530, 178.3980910637346255 ) ) ;
#108783=ORIENTED_EDGE ( 'NONE', *, *, #79618, .F. ) ;
#108813=CARTESIAN_POINT ( 'NONE',  ( 31.92312126443668419, 1524.775785348138015, 216.6640869107574758 ) ) ;
#108815=CARTESIAN_POINT ( 'NONE',  ( 3.687149994097108433E-15, 1511.187213306747708, 239.2297105040643714 ) ) ;
#108825=CARTESIAN_POINT ( 'NONE',  ( 17.10337015680181239, 1524.478200376951690, 237.2711292833226366 ) ) ;
#108827=CARTESIAN_POINT ( 'NONE',  ( -29.66215386746315374, 1526.345556099435726, 201.2527107338347321 ) ) ;
#108849=DIRECTION ( 'NONE',  ( 0.000000000000000000, 0.000000000000000000, 1.000000000000000000 ) ) ;
#108859=VERTEX_POINT ( 'NONE', #71997 ) ;
#108860=EDGE_CURVE ( 'NONE', #13119, #13894, #55570, .T. ) ;
#108874=ORIENTED_EDGE ( 'NONE', *, *, #36650, .F. ) ;
#108894=EDGE_CURVE ( 'NONE', #47496, #80799, #45684, .T. ) ;
#108905=ADVANCED_FACE ( 'NONE', ( #99337 ), #89508, .T. ) ;
#108916=CARTESIAN_POINT ( 'NONE',  ( 29.99620953741496621, 1526.382868172863937, 219.7462484079458704 ) ) ;
#108917=ORIENTED_EDGE ( 'NONE', *, *, #34328, .T. ) ;
#108922=DIRECTION ( 'NONE',  ( -0.2054769195713184726, 3.564456361518036305E-16, 0.9786619618251657382 ) ) ;
#108932=CIRCLE ( 'NONE', #85647, 2.000000000000000444 ) ;
#108936=CARTESIAN_POINT ( 'NONE',  ( 20.28160989817542870, 1526.000688113705564, 184.8337570730933237 ) ) ;
#108945=CARTESIAN_POINT ( 'NONE',  ( -32.38845791999504797, 1523.456872492435195, 202.1182848005516632 ) ) ;
#108958=B_SPLINE_CURVE_WITH_KNOTS ( 'NONE', 3,
 ( #43012, #77169, #92292, #49763 ),
 .UNSPECIFIED., .F., .F.,
 ( 4, 4 ),
 ( 0.000000000000000000, 0.0002960034161023848936 ),
 .UNSPECIFIED. ) ;
#108964=DIRECTION ( 'NONE',  ( -0.1070030146457317810, 0.000000000000000000, 0.9942586961433755866 ) ) ;
#108983=ADVANCED_FACE ( 'NONE', ( #2457 ), #36033, .T. ) ;
#108986=CARTESIAN_POINT ( 'NONE',  ( -18.86688640473622414, 1511.187213306747708, 180.7825021045441076 ) ) ;
#108990=CARTESIAN_POINT ( 'NONE',  ( 2.165176160181189857, 1526.186458717540972, 240.2894009330130132 ) ) ;
#109011=ORIENTED_EDGE ( 'NONE', *, *, #104098, .T. ) ;
#109026=EDGE_LOOP ( 'NONE', ( #27411, #14414, #66730, #44975, #8133 ) ) ;
#109028=CARTESIAN_POINT ( 'NONE',  ( -28.82451532742324929, 1526.348417187219184, 220.0525736641747017 ) ) ;
#109032=AXIS2_PLACEMENT_3D ( 'NONE', #13458, #8791, #24486 ) ;
#109035=DIRECTION ( 'NONE',  ( 0.000000000000000000, 0.000000000000000000, 1.000000000000000000 ) ) ;
#109056=TOROIDAL_SURFACE ( 'NONE', #23191, 2.000000000000000000, 1.000000000000000000 ) ;
#109060=ORIENTED_EDGE ( 'NONE', *, *, #49397, .F. ) ;
#109073=CARTESIAN_POINT ( 'NONE',  ( -21.83550407203940580, 1523.678648413191695, 183.2743720722710350 ) ) ;
#109092=CARTESIAN_POINT ( 'NONE',  ( -2.470168521978398868, 1512.187213306747481, 175.3649660270905315 ) ) ;
#109096=CARTESIAN_POINT ( 'NONE',  ( 31.97190655716360652, 1524.330813522192102, 216.6896206998345349 ) ) ;
#109105=CARTESIAN_POINT ( 'NONE',  ( 3.347801439296143933, 1523.382868172864164, 242.0893193391992497 ) ) ;
#109107=AXIS2_PLACEMENT_3D ( 'NONE', #97839, #87253, #18918 ) ;
#109110=CARTESIAN_POINT ( 'NONE',  ( -22.08327125186908191, 1523.604703353109699, 233.8169256665491105 ) ) ;
#109121=CARTESIAN_POINT ( 'NONE',  ( -21.10560967990489090, 1525.661276915132476, 184.9336828786751141 ) ) ;
#109135=ADVANCED_FACE ( 'NONE', ( #44295 ), #10688, .T. ) ;
#109161=CARTESIAN_POINT ( 'NONE',  ( -0.4151546846821903003, 1512.187213306747481, 175.3106345060153046 ) ) ;
#109162=CARTESIAN_POINT ( 'NONE',  ( -32.38845791999490586, 1518.913060387330006, 216.1254071228449902 ) ) ;
#109173=AXIS2_PLACEMENT_3D ( 'NONE', #26939, #8462, #9569 ) ;
#109187=CARTESIAN_POINT ( 'NONE',  ( 29.86461515634920971, 1525.960063244517187, 220.9690070206020494 ) ) ;
#109192=VERTEX_POINT ( 'NONE', #29129 ) ;
#109194=AXIS2_PLACEMENT_3D ( 'NONE', #43457, #33929, #77604 ) ;
#109219=CARTESIAN_POINT ( 'NONE',  ( -2.180465155517639531, 1524.667648926078755, 173.9851435850430335 ) ) ;
#109220=DIRECTION ( 'NONE',  ( -0.9942586961433751425, 0.000000000000000000, 0.1070030146457376097 ) ) ;
#109225=ORIENTED_EDGE ( 'NONE', *, *, #92721, .T. ) ;
#109228=CARTESIAN_POINT ( 'NONE',  ( 34.18677586421189574, 1512.187213306747481, 219.7932833225211766 ) ) ;
#109280=CIRCLE ( 'NONE', #61020, 1.000000000000002442 ) ;
#109283=DIRECTION ( 'NONE',  ( 0.5877852522924709167, 0.000000000000000000, 0.8090169943749491166 ) ) ;
#109286=CARTESIAN_POINT ( 'NONE',  ( -22.08622291482368283, 1518.913060387330006, 184.4183880513178337 ) ) ;
#109305=ORIENTED_EDGE ( 'NONE', *, *, #38125, .F. ) ;
#109328=ORIENTED_EDGE ( 'NONE', *, *, #110238, .F. ) ;
#109331=DIRECTION ( 'NONE',  ( -0.000000000000000000, -1.000000000000000000, -0.000000000000000000 ) ) ;
#109335=CARTESIAN_POINT ( 'NONE',  ( 0.000000000000000000, 1511.187213306747708, 209.1218459616979999 ) ) ;
#109355=CARTESIAN_POINT ( 'NONE',  ( -32.38845791999490586, 1523.382868172864164, 216.1254071228449902 ) ) ;
#109371=CARTESIAN_POINT ( 'NONE',  ( 21.76695791008653558, 1524.152349020271004, 234.8391556417741697 ) ) ;
#109376=CARTESIAN_POINT ( 'NONE',  ( 32.02808312589916540, 1511.187213306747708, 197.2787714533495489 ) ) ;
#109378=CARTESIAN_POINT ( 'NONE',  ( -30.61619818474167687, 1525.211477436245787, 221.5983981500683058 ) ) ;
#109393=DIRECTION ( 'NONE',  ( -0.000000000000000000, -1.000000000000000000, -0.000000000000000000 ) ) ;
#109395=CARTESIAN_POINT ( 'NONE',  ( 16.48227125551174765, 1525.651285554128663, 236.6829039301441924 ) ) ;
#109425=ORIENTED_EDGE ( 'NONE', *, *, #23434, .T. ) ;
#109434=ORIENTED_EDGE ( 'NONE', *, *, #89772, .T. ) ;
#109465=AXIS2_PLACEMENT_3D ( 'NONE', #54276, #95699, #62689 ) ;
#109467=CARTESIAN_POINT ( 'NONE',  ( -3.347801439296150150, 1523.382868172864164, 242.0893193391992497 ) ) ;
#109476=ORIENTED_EDGE ( 'NONE', *, *, #13717, .T. ) ;
#109491=CARTESIAN_POINT ( 'NONE',  ( 19.39983987835422496, 1501.977400791986611, 239.2921289694223219 ) ) ;
#109492=DIRECTION ( 'NONE',  ( 0.000000000000000000, 0.000000000000000000, 1.000000000000000000 ) ) ;
#109494=DIRECTION ( 'NONE',  ( 0.000000000000000000, 1.000000000000000000, 0.000000000000000000 ) ) ;
#109496=EDGE_CURVE ( 'NONE', #100644, #50057, #39484, .T. ) ;
#109508=ORIENTED_EDGE ( 'NONE', *, *, #65823, .T. ) ;
#109511=VERTEX_POINT ( 'NONE', #30935 ) ;
#109513=CARTESIAN_POINT ( 'NONE',  ( 33.36586802512179162, 1511.187213306747708, 216.3367586934468818 ) ) ;
#109514=CARTESIAN_POINT ( 'NONE',  ( -18.66420869458028520, 1526.382868172864164, 232.7837831374281166 ) ) ;
#109529=ORIENTED_EDGE ( 'NONE', *, *, #32373, .F. ) ;
#109561=ADVANCED_FACE ( 'NONE', ( #87413 ), #35909, .F. ) ;
#109568=DIRECTION ( 'NONE',  ( -0.000000000000000000, -1.000000000000000000, -0.000000000000000000 ) ) ;
#109587=ORIENTED_EDGE ( 'NONE', *, *, #23926, .T. ) ;
#109588=CARTESIAN_POINT ( 'NONE',  ( -3.355893228018326457, 1523.847248782568613, 242.0621646443070745 ) ) ;
#109592=CARTESIAN_POINT ( 'NONE',  ( 16.81464677261734764, 1526.382868172863937, 183.7052044321627022 ) ) ;
#109606=CARTESIAN_POINT ( 'NONE',  ( 3.017180836140621825, 1525.408327360769817, 176.9098388056617068 ) ) ;
#109618=ORIENTED_EDGE ( 'NONE', *, *, #15380, .T. ) ;
#109619=EDGE_CURVE ( 'NONE', #82949, #40736, #109626, .T. ) ;
#109623=EDGE_CURVE ( 'NONE', #71455, #16677, #66812, .T. ) ;
#109626=B_SPLINE_CURVE_WITH_KNOTS ( 'NONE', 3,
 ( #90695, #82308, #106951, #105871, #97458, #47068, #97993, #22365 ),
 .UNSPECIFIED., .F., .F.,
 ( 4, 2, 2, 4 ),
 ( 2.428612866367530240E-17, 0.001073044933456045527, 0.001609567400184072844, 0.002146089866912100162 ),
 .UNSPECIFIED. ) ;
#109636=ADVANCED_FACE ( 'NONE', ( #72818 ), #71738, .T. ) ;
#109643=DIRECTION ( 'NONE',  ( 0.000000000000000000, 1.000000000000000000, 0.000000000000000000 ) ) ;
#109653=DIRECTION ( 'NONE',  ( 0.000000000000000000, 0.8724564897876694314, -0.4886917979947875135 ) ) ;
#109657=ORIENTED_EDGE ( 'NONE', *, *, #4657, .F. ) ;
#109659=CARTESIAN_POINT ( 'NONE',  ( 16.68062049856724016, 1524.382868172863937, 236.8314524626096045 ) ) ;
#109680=ORIENTED_EDGE ( 'NONE', *, *, #44798, .F. ) ;
#109682=CARTESIAN_POINT ( 'NONE',  ( -2.700472180932728783, 1524.678541297861329, 176.3823254397200344 ) ) ;
#109689=EDGE_LOOP ( 'NONE', ( #21907, #85865, #58371, #74333, #3020 ) ) ;
#109722=CARTESIAN_POINT ( 'NONE',  ( 30.16752008203805602, 1524.964158026966061, 196.5181576271968140 ) ) ;
#109743=AXIS2_PLACEMENT_3D ( 'NONE', #62925, #20299, #54503 ) ;
#109752=DIRECTION ( 'NONE',  ( 0.000000000000000000, 1.000000000000000000, 0.000000000000000000 ) ) ;
#109755=CARTESIAN_POINT ( 'NONE',  ( -2.456601303385837820, 1523.611961620354123, 175.3003469896239039 ) ) ;
#109760=DIRECTION ( 'NONE',  ( 0.000000000000000000, 0.000000000000000000, -1.000000000000000000 ) ) ;
#109764=CARTESIAN_POINT ( 'NONE',  ( 34.18677586421189574, 1522.382868172863937, 219.7932833225211766 ) ) ;
#109774=TOROIDAL_SURFACE ( 'NONE', #70482, 1.000000000000000000, 1.000000000000000000 ) ;
#109780=CARTESIAN_POINT ( 'NONE',  ( 32.38114538885250226, 1523.604703353109699, 202.1233279672528624 ) ) ;
#109787=DIRECTION ( 'NONE',  ( 0.000000000000000000, 0.000000000000000000, 1.000000000000000000 ) ) ;
#109794=EDGE_CURVE ( 'NONE', #105489, #36910, #64855, .T. ) ;
#109812=EDGE_CURVE ( 'NONE', #81031, #56488, #107925, .T. ) ;
#109814=ORIENTED_EDGE ( 'NONE', *, *, #88704, .T. ) ;
#109830=ORIENTED_EDGE ( 'NONE', *, *, #16426, .F. ) ;
#109831=ORIENTED_EDGE ( 'NONE', *, *, #37764, .T. ) ;
#109832=CIRCLE ( 'NONE', #20446, 1.999999999999998668 ) ;
#109871=CARTESIAN_POINT ( 'NONE',  ( -21.42841630977142131, 1524.678872986499073, 234.0212620058165385 ) ) ;
#109883=DIRECTION ( 'NONE',  ( -0.000000000000000000, -1.000000000000000000, -0.000000000000000000 ) ) ;
#109887=CARTESIAN_POINT ( 'NONE',  ( -32.28466283162143213, 1511.187213306747708, 219.1752493337717738 ) ) ;
#109891=CARTESIAN_POINT ( 'NONE',  ( -32.38601978689771244, 1523.530870145309336, 216.1237258104784758 ) ) ;
#109906=CIRCLE ( 'NONE', #32997, 2.000000000000001776 ) ;
#109910=CARTESIAN_POINT ( 'NONE',  ( -30.15954682509861584, 1524.412928176728883, 195.8337490977937989 ) ) ;
#109921=DIRECTION ( 'NONE',  ( 0.000000000000000000, 1.000000000000000000, 0.000000000000000000 ) ) ;
#109931=CARTESIAN_POINT ( 'NONE',  ( 16.49871405536215363, 1525.320849883639994, 181.2023611689214135 ) ) ;
#109936=CARTESIAN_POINT ( 'NONE',  ( 16.92737834737011582, 1525.317349363549965, 236.7941106564731513 ) ) ;
#109959=DIRECTION ( 'NONE',  ( 0.000000000000000000, 0.000000000000000000, 1.000000000000000000 ) ) ;
#109961=LINE ( 'NONE', #33240, #60453 ) ;
#109994=AXIS2_PLACEMENT_3D ( 'NONE', #6125, #48154, #47054 ) ;
#110023=FACE_OUTER_BOUND ( 'NONE', #101534, .T. ) ;
#110033=CARTESIAN_POINT ( 'NONE',  ( -21.78062404853642064, 1524.843178112495480, 184.6507237701596580 ) ) ;
#110037=ORIENTED_EDGE ( 'NONE', *, *, #97878, .T. ) ;
#110056=ORIENTED_EDGE ( 'NONE', *, *, #90057, .T. ) ;
#110076=CIRCLE ( 'NONE', #61843, 0.9999999999999074074 ) ;
#110085=CARTESIAN_POINT ( 'NONE',  ( 0.000000000000000000, 0.000000000000000000, 0.000000000000000000 ) ) ;
#110115=DIRECTION ( 'NONE',  ( 0.000000000000000000, 1.000000000000000000, 0.000000000000000000 ) ) ;
#110148=EDGE_CURVE ( 'NONE', #31391, #102452, #82410, .T. ) ;
#110152=CARTESIAN_POINT ( 'NONE',  ( 18.19590854888146580, 1512.187213306747481, 180.0410247165184217 ) ) ;
#110154=CARTESIAN_POINT ( 'NONE',  ( -32.28466283162165240, 1512.187213306747481, 199.0684425896249081 ) ) ;
#110178=VERTEX_POINT ( 'NONE', #32674 ) ;
#110208=EDGE_CURVE ( 'NONE', #81551, #71185, #50290, .T. ) ;
#110219=CARTESIAN_POINT ( 'NONE',  ( -33.28034951413935971, 1522.382868172863937, 200.8029765415142549 ) ) ;
#110230=CARTESIAN_POINT ( 'NONE',  ( 49.24962907673571522, 1524.382868172863937, 10.34030387146701813 ) ) ;
#110238=EDGE_CURVE ( 'NONE', #36007, #5947, #184, .T. ) ;
#110239=ORIENTED_EDGE ( 'NONE', *, *, #2998, .T. ) ;
#110241=DIRECTION ( 'NONE',  ( 0.000000000000000000, 1.000000000000000000, 0.000000000000000000 ) ) ;
#110245=B_SPLINE_CURVE_WITH_KNOTS ( 'NONE', 3,
 ( #93039, #15218, #108749, #41555, #7390, #92482, #93580, #8476, #42650, #24710 ),
 .UNSPECIFIED., .F., .F.,
 ( 4, 2, 2, 2, 4 ),
 ( 0.000000000000000000, 0.0007189769279726049766, 0.001437953855945209953, 0.002156930783917814821, 0.002875907711890419906 ),
 .UNSPECIFIED. ) ;
#110263=CARTESIAN_POINT ( 'NONE',  ( 30.24979188206187786, 1524.075000532257036, 195.7694503965884394 ) ) ;
#110268=CARTESIAN_POINT ( 'NONE',  ( 3.062921356683458551, 1525.320849883635901, 241.4068844367821782 ) ) ;
#110270=CARTESIAN_POINT ( 'NONE',  ( -32.86802468363566732, 1523.481610118013805, 201.0396662541351418 ) ) ;
#110288=CARTESIAN_POINT ( 'NONE',  ( -29.33952678943997228, 1526.382868172864164, 201.1028049641089694 ) ) ;
#110306=CARTESIAN_POINT ( 'NONE',  ( 1.393816646507355150, 1511.187213306747708, 243.1385343369520342 ) ) ;
#110308=DIRECTION ( 'NONE',  ( -0.1070030146457317810, 0.000000000000000000, 0.9942586961433755866 ) ) ;
#110309=LINE ( 'NONE', #59385, #72996 ) ;
#110318=CARTESIAN_POINT ( 'NONE',  ( 2.038847259689231084, 1501.977400791986611, 244.9330574173806951 ) ) ;
#110324=DIRECTION ( 'NONE',  ( -0.000000000000000000, -1.000000000000000000, -0.000000000000000000 ) ) ;
#110330=ADVANCED_FACE ( 'NONE', ( #32547 ), #37951, .F. ) ;
#110343=DIRECTION ( 'NONE',  ( -0.000000000000000000, -1.000000000000000000, -0.000000000000000000 ) ) ;
#110345=CARTESIAN_POINT ( 'NONE',  ( -30.90487439922528168, 1525.907212628473644, 216.4335774778784582 ) ) ;
#110355=EDGE_LOOP ( 'NONE', ( #72841, #83119, #97455, #7155 ) ) ;
#110372=ORIENTED_EDGE ( 'NONE', *, *, #31065, .T. ) ;
#110374=VECTOR ( 'NONE', #94300, 1000.000000000000000 ) ;
#110389=ORIENTED_EDGE ( 'NONE', *, *, #37244, .F. ) ;
#110396=ORIENTED_EDGE ( 'NONE', *, *, #16591, .T. ) ;
#110431=EDGE_CURVE ( 'NONE', #42994, #41235, #33442, .T. ) ;
#110441=EDGE_CURVE ( 'NONE', #40151, #47989, #91356, .T. ) ;
#110459=CARTESIAN_POINT ( 'NONE',  ( 29.30029655192942073, 1525.907212628473644, 196.8717316207784620 ) ) ;
#110468=DIRECTION ( 'NONE',  ( 0.000000000000000000, 0.000000000000000000, 1.000000000000000000 ) ) ;
#110469=AXIS2_PLACEMENT_3D ( 'NONE', #71985, #71443, #63577 ) ;
#110476=CARTESIAN_POINT ( 'NONE',  ( 16.99777429700839093, 1524.964158026965379, 181.1932245048199377 ) ) ;
#110483=FACE_OUTER_BOUND ( 'NONE', #55464, .T. ) ;
#110484=DIRECTION ( 'NONE',  ( -0.06728379684271972028, -0.9969860201949397593, 0.03862338952348403492 ) ) ;
#110486=CARTESIAN_POINT ( 'NONE',  ( -9.373950541344154175, 1512.187213306747481, 228.8708405320809902 ) ) ;
#110487=AXIS2_PLACEMENT_3D ( 'NONE', #52234, #19708, #18585 ) ;
#110491=CARTESIAN_POINT ( 'NONE',  ( -21.38516915558007625, 1512.187213306747481, 180.3939891059723664 ) ) ;
#110495=ORIENTED_EDGE ( 'NONE', *, *, #31181, .F. ) ;
#110517=ORIENTED_EDGE ( 'NONE', *, *, #1118, .T. ) ;
#110540=CARTESIAN_POINT ( 'NONE',  ( 20.98221433429012350, 1524.841055067851130, 181.0917269138614358 ) ) ;
#110543=AXIS2_PLACEMENT_3D ( 'NONE', #59643, #6603, #40753 ) ;
#110566=VECTOR ( 'NONE', #78116, 1000.000000000000000 ) ;
#110571=EDGE_CURVE ( 'NONE', #23046, #70982, #60060, .T. ) ;
#110573=CARTESIAN_POINT ( 'NONE',  ( -34.09113935471027190, 1523.429859730330918, 219.7507174562243506 ) ) ;
#110582=FACE_OUTER_BOUND ( 'NONE', #27096, .T. ) ;
#110606=ORIENTED_EDGE ( 'NONE', *, *, #10300, .F. ) ;
#110608=DIRECTION ( 'NONE',  ( -0.7414773880254761362, 0.000000000000000000, -0.6709778558543624261 ) ) ;
#110620=CIRCLE ( 'NONE', #81998, 0.9999999999999997780 ) ;
#110639=CARTESIAN_POINT ( 'NONE',  ( 2.225543501807631053, 1525.712835404586031, 241.5729910383504659 ) ) ;
#110649=CARTESIAN_POINT ( 'NONE',  ( -76.99707197885047094, 1524.382868172863937, 398.8876973329340672 ) ) ;
#110664=AXIS2_PLACEMENT_3D ( 'NONE', #42793, #7528, #103221 ) ;
#110688=CIRCLE ( 'NONE', #44529, 1.999999999999996225 ) ;
#110699=CARTESIAN_POINT ( 'NONE',  ( 2.708195641335804371, 1524.374578187332872, 176.2568186770878356 ) ) ;
#110701=UNCERTAINTY_MEASURE_WITH_UNIT (LENGTH_MEASURE( 1.000000000000000082E-05 ), #31586, 'distance_accuracy_value', 'NONE');
#110702=CARTESIAN_POINT ( 'NONE',  ( -30.51231035492526900, 1526.382868172863937, 200.0858385050243555 ) ) ;
#110705=DIRECTION ( 'NONE',  ( 0.2113515706023144647, 0.000000000000000000, 0.9774101051267757301 ) ) ;
#110711=CARTESIAN_POINT ( 'NONE',  ( 2.737416067801674124, 1524.382868172804365, 241.6058578387444982 ) ) ;
#110721=CARTESIAN_POINT ( 'NONE',  ( 29.61692403811556673, 1526.104292489129421, 220.7563138442888828 ) ) ;
#110731=CARTESIAN_POINT ( 'NONE',  ( 34.31402925621713962, 1524.244163922423695, 218.0340858097454202 ) ) ;
#110740=CARTESIAN_POINT ( 'NONE',  ( 31.34137657934008558, 1523.481610426287716, 196.3411265156547358 ) ) ;
#110745=CARTESIAN_POINT ( 'NONE',  ( -21.83550407203883736, 1523.678648413191695, 234.9693198511253627 ) ) ;
#110757=CARTESIAN_POINT ( 'NONE',  ( -18.02257621027615642, 1524.382868172863937, 182.8951942368373977 ) ) ;
#110758=DIRECTION ( 'NONE',  ( 0.000000000000000000, 1.000000000000000000, 0.000000000000000000 ) ) ;
#110777=TOROIDAL_SURFACE ( 'NONE', #14213, 30.13701971169416538, 3.000000000000000000 ) ;
#110781=CARTESIAN_POINT ( 'NONE',  ( -3.062921356683425245, 1525.320849883635901, 176.8368074866138215 ) ) ;
#110786=DIRECTION ( 'NONE',  ( -0.3090169943749383474, -0.000000000000000000, 0.9510565162951566398 ) ) ;
#110795=DIRECTION ( 'NONE',  ( -0.1070030146457454923, 0.000000000000000000, -0.9942586961433741433 ) ) ;
#110805=ORIENTED_EDGE ( 'NONE', *, *, #33532, .T. ) ;
#110820=CARTESIAN_POINT ( 'NONE',  ( 30.12464261468161197, 1524.523992613102564, 195.8613510089864747 ) ) ;
ENDSEC;
END-ISO-10303-21;
